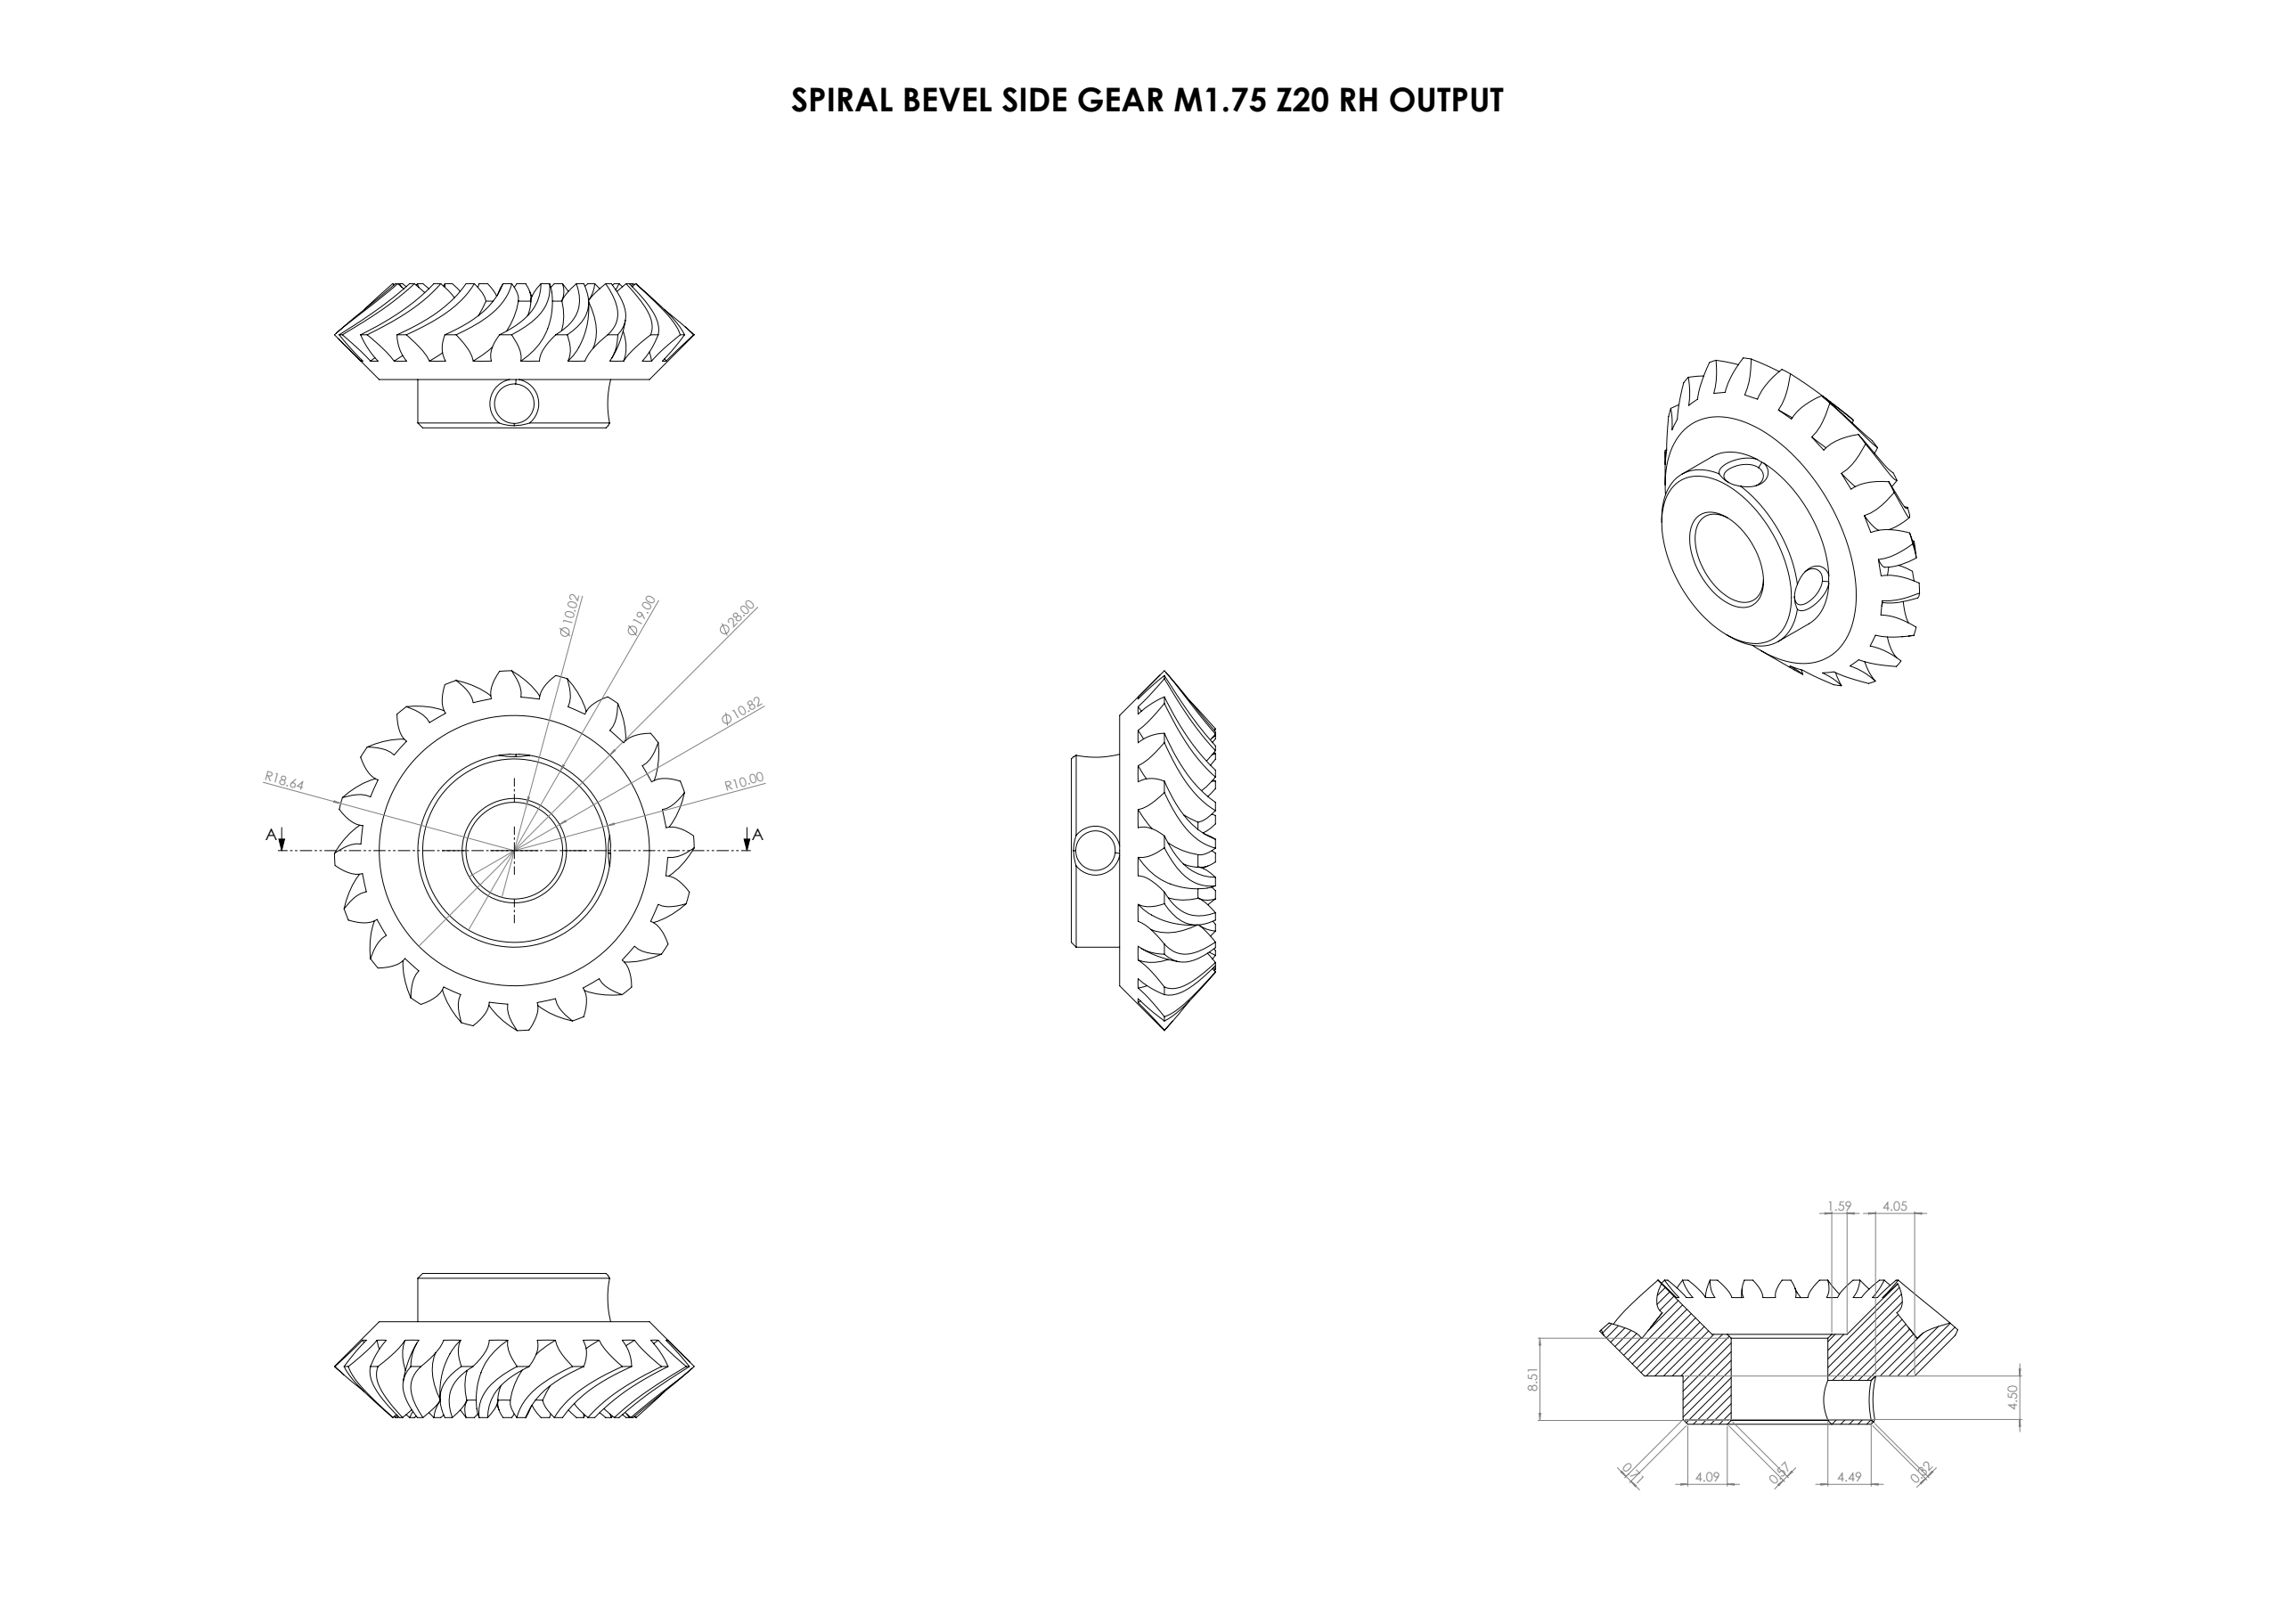
ISO-10303-21;
HEADER;
/* Generated by software containing ST-Developer
 * from STEP Tools, Inc. (www.steptools.com) 
 */

FILE_DESCRIPTION(
/* description */ (''),
/* implementation_level */ '2;1');

FILE_NAME(
/* name */ 
'04_Spiral_Bevel_Side_Gear_m1.75_z20_RH_Output.step',
/* time_stamp */ '2026-10-22T00:21:42-07:00',
/* author */ (''),
/* organization */ (''),
/* preprocessor_version */ 'ST-DEVELOPER v20.2',
/* originating_system */ 'Autodesk Translation Framework v15.15.0.0',
/* authorisation */ '');

FILE_SCHEMA (('AUTOMOTIVE_DESIGN { 1 0 10303 214 3 1 1 }'));
ENDSEC;

DATA;
#10=MECHANICAL_DESIGN_GEOMETRIC_PRESENTATION_REPRESENTATION('',(#208),#31638);
#186=SHAPE_REPRESENTATION_RELATIONSHIP('SRR','None',#31708,#197);
#197=ADVANCED_BREP_SHAPE_REPRESENTATION('',(#219),#31630);
#208=STYLED_ITEM('',(#31823),#219);
#219=MANIFOLD_SOLID_BREP('Spiral bevel gear',#12483);
#272=CYLINDRICAL_SURFACE('',#12901,1.);
#273=CYLINDRICAL_SURFACE('',#12905,1.);
#274=CYLINDRICAL_SURFACE('',#12908,0.205);
#275=CYLINDRICAL_SURFACE('',#12909,0.205);
#276=CYLINDRICAL_SURFACE('',#12981,0.501);
#406=CONICAL_SURFACE('',#12910,0.975,0.785398163397446);
#407=CONICAL_SURFACE('',#12912,1.63192209588552,0.785398163397448);
#408=CONICAL_SURFACE('',#12934,1.56260147929642,0.850360450324169);
#409=CONICAL_SURFACE('',#12936,1.56260147929642,0.850360450324169);
#410=CONICAL_SURFACE('',#12938,1.56260147929642,0.850360450324169);
#411=CONICAL_SURFACE('',#12940,1.56260147929642,0.850360450324169);
#412=CONICAL_SURFACE('',#12942,1.56260147929642,0.850360450324169);
#413=CONICAL_SURFACE('',#12944,1.56260147929642,0.850360450324169);
#414=CONICAL_SURFACE('',#12946,1.56260147929642,0.850360450324169);
#415=CONICAL_SURFACE('',#12948,1.56260147929642,0.850360450324169);
#416=CONICAL_SURFACE('',#12950,1.56260147929642,0.850360450324169);
#417=CONICAL_SURFACE('',#12952,1.56260147929642,0.850360450324169);
#418=CONICAL_SURFACE('',#12954,1.56260147929642,0.850360450324169);
#419=CONICAL_SURFACE('',#12956,1.56260147929642,0.850360450324169);
#420=CONICAL_SURFACE('',#12958,1.56260147929642,0.850360450324169);
#421=CONICAL_SURFACE('',#12960,1.56260147929642,0.850360450324169);
#422=CONICAL_SURFACE('',#12962,1.56260147929642,0.850360450324169);
#423=CONICAL_SURFACE('',#12964,1.56260147929642,0.850360450324169);
#424=CONICAL_SURFACE('',#12966,1.56260147929642,0.850360450324169);
#425=CONICAL_SURFACE('',#12968,1.56260147929642,0.850360450324169);
#426=CONICAL_SURFACE('',#12970,1.56260147929642,0.850360450324169);
#427=CONICAL_SURFACE('',#12972,0.980679383410898,0.785398163397448);
#428=CONICAL_SURFACE('',#12975,1.56260147929642,0.850360450324169);
#429=CONICAL_SURFACE('',#12979,0.521,0.785398163397448);
#430=CONICAL_SURFACE('',#12983,0.521,0.785398163397451);
#723=B_SPLINE_CURVE_WITH_KNOTS('',3,(#21270,#21271,#21272,#21273,#21274,
#21275,#21276,#21277,#21278,#21279,#21280,#21281,#21282,#21283,#21284,#21285,
#21286,#21287,#21288,#21289,#21290,#21291,#21292,#21293,#21294,#21295,#21296,
#21297,#21298,#21299,#21300,#21301,#21302,#21303),.UNSPECIFIED.,.F.,.F.,
(4,3,3,3,3,3,3,3,3,3,3,4),(0.,0.0110116267986798,0.0198365927950272,0.0393688637311641,
0.0455583406049715,0.0493231568143408,0.0527005792502689,0.056916196494854,
0.0651768568763584,0.0788461297337949,0.0828398890027903,0.100882854089343),
 .UNSPECIFIED.);
#724=B_SPLINE_CURVE_WITH_KNOTS('',3,(#21305,#21306,#21307,#21308,#21309,
#21310,#21311,#21312,#21313,#21314,#21315,#21316,#21317,#21318),
 .UNSPECIFIED.,.F.,.F.,(4,1,1,1,1,1,1,1,1,2,4),(-0.889886066635509,-0.843971490026765,
-0.78979558357151,-0.749163653730069,-0.681443770661001,-0.654355817433373,
-0.627267864205746,-0.600179910978118,-0.573091957750491,-0.464740144839981,
-0.44137654239973),.UNSPECIFIED.);
#725=B_SPLINE_CURVE_WITH_KNOTS('',3,(#21320,#21321,#21322,#21323,#21324,
#21325,#21326,#21327,#21328,#21329,#21330,#21331),.UNSPECIFIED.,.F.,.F.,
(4,2,2,2,2,4),(0.,0.0358257028990328,0.131952299625094,0.148884451735932,
0.157379698574708,0.16223106694039),.UNSPECIFIED.);
#726=B_SPLINE_CURVE_WITH_KNOTS('',3,(#21333,#21334,#21335,#21336),
 .UNSPECIFIED.,.F.,.F.,(4,4),(0.549999999941368,1.),.UNSPECIFIED.);
#727=B_SPLINE_CURVE_WITH_KNOTS('',3,(#21338,#21339,#21340,#21341,#21342,
#21343,#21344,#21345,#21346,#21347,#21348,#21349,#21350,#21351,#21352,#21353),
 .UNSPECIFIED.,.F.,.F.,(4,1,2,1,1,1,1,1,1,1,1,1,4),(0.310721506882948,0.387730825861464,
0.464740144839981,0.573091957750491,0.600179910978118,0.627267864205746,
0.654355817433373,0.681443770661001,0.749163653730069,0.78979558357151,
0.843971490026765,0.89814739648202,0.929489890414014),.UNSPECIFIED.);
#728=B_SPLINE_CURVE_WITH_KNOTS('',3,(#21354,#21355,#21356,#21357,#21358,
#21359,#21360,#21361,#21362,#21363,#21364,#21365,#21366,#21367,#21368,#21369,
#21370),.UNSPECIFIED.,.F.,.F.,(4,1,1,1,1,1,1,1,1,1,1,1,1,1,4),(0.929489890414014,
0.952323302937276,1.00649920939253,1.06067511584779,1.11485102230304,1.1690269287583,
1.22320283521355,1.26383476505499,1.33155464812406,1.35864260135169,1.38573055457932,
1.41281850780694,1.43990646103457,1.49408236748983,1.54825827394508),
 .UNSPECIFIED.);
#729=B_SPLINE_CURVE_WITH_KNOTS('',3,(#21372,#21373,#21374,#21375,#21376,
#21377,#21378,#21379,#21380,#21381,#21382,#21383,#21384,#21385),
 .UNSPECIFIED.,.F.,.F.,(4,2,2,2,2,2,4),(0.16223106694039,0.163967550885131,
0.171180716857468,0.182777598096348,0.205784524866042,0.262730804446443,
0.324280670363194),.UNSPECIFIED.);
#730=B_SPLINE_CURVE_WITH_KNOTS('',3,(#21386,#21387,#21388,#21389,#21390,
#21391,#21392,#21393,#21394,#21395,#21396,#21397,#21398,#21399),
 .UNSPECIFIED.,.F.,.F.,(4,1,1,1,1,1,1,1,1,1,1,4),(-1.4176032384283,-1.41281850780694,
-1.38573055457932,-1.35864260135169,-1.33155464812406,-1.26383476505499,
-1.22320283521355,-1.1690269287583,-1.11485102230304,-1.06067511584779,
-1.00649920939253,-0.969093714192518),.UNSPECIFIED.);
#731=B_SPLINE_CURVE_WITH_KNOTS('',3,(#21406,#21407,#21408,#21409,#21410,
#21411,#21412,#21413,#21414,#21415,#21416,#21417),.UNSPECIFIED.,.F.,.F.,
(4,1,1,1,1,1,1,2,4),(-1.50954599357819,-1.43295998077967,-1.38938999215504,
-1.34582000353042,-1.25868002628116,-1.21511003765654,-1.17154004903191,
-1.08440007178266,-1.06103646934241),.UNSPECIFIED.);
#732=B_SPLINE_CURVE_WITH_KNOTS('',3,(#21423,#21424,#21425,#21426,#21427,
#21428,#21429,#21430,#21431,#21432,#21433,#21434,#21435,#21436),
 .UNSPECIFIED.,.F.,.F.,(4,1,1,1,2,2,1,1,1,4),(-2.03726316537097,-2.03275764211163,
-2.01344899085789,-1.93621438584296,-1.85897978082803,-1.78151988977668,
-1.71616490683974,-1.69437991252743,-1.60723993527817,-1.58875364113519),
 .UNSPECIFIED.);
#733=B_SPLINE_CURVE_WITH_KNOTS('',3,(#21442,#21443,#21444,#21445,#21446,
#21447,#21448,#21449,#21450,#21451),.UNSPECIFIED.,.F.,.F.,(4,2,2,2,4),(0.,
0.0782721603764034,0.156544320752807,0.234729089704077,0.312913858655347),
 .UNSPECIFIED.);
#734=B_SPLINE_CURVE_WITH_KNOTS('',3,(#21452,#21453,#21454,#21455,#21456,
#21457,#21458,#21459,#21460,#21461,#21462,#21463,#21464,#21465,#21466,#21467,
#21468,#21469,#21470,#21471,#21472,#21473,#21474,#21475,#21476,#21477),
 .UNSPECIFIED.,.F.,.F.,(4,2,2,2,2,2,2,2,2,2,2,2,4),(0.312913858655347,0.391098627606618,
0.469283396557888,0.547555556934292,0.625827717310695,0.704099877687098,
0.782372038063502,0.860556807014772,0.938741575966043,1.01692634491731,
1.09511111386858,1.17338327424499,1.25165543462139),.UNSPECIFIED.);
#735=B_SPLINE_CURVE_WITH_KNOTS('',3,(#21590,#21591,#21592,#21593,#21594,
#21595,#21596,#21597,#21598,#21599,#21600,#21601,#21602,#21603,#21604,#21605,
#21606,#21607,#21608,#21609,#21610,#21611,#21612,#21613,#21614,#21615,#21616,
#21617,#21618,#21619,#21620,#21621,#21622,#21623,#21624,#21625,#21626),
 .UNSPECIFIED.,.F.,.F.,(4,3,3,3,3,3,3,3,3,3,3,3,4),(0.,0.0140126898858465,
0.0198365927950119,0.0393688637311589,0.0455583406050571,0.0493231568139791,
0.0527005792494364,0.0569161964938546,0.0651768568751002,0.0683276956644967,
0.0828398890011837,0.0964479725722503,0.100882854087323),.UNSPECIFIED.);
#736=B_SPLINE_CURVE_WITH_KNOTS('',3,(#21628,#21629,#21630,#21631,#21632,
#21633,#21634,#21635,#21636,#21637,#21638,#21639),.UNSPECIFIED.,.F.,.F.,
(4,2,2,2,2,4),(0.,0.0358257028990433,0.131952299625135,0.148884451735976,
0.157379698574799,0.162231066940522),.UNSPECIFIED.);
#737=B_SPLINE_CURVE_WITH_KNOTS('',3,(#21641,#21642,#21643,#21644),
 .UNSPECIFIED.,.F.,.F.,(4,4),(0.549999999941368,1.),.UNSPECIFIED.);
#738=B_SPLINE_CURVE_WITH_KNOTS('',3,(#21646,#21647,#21648,#21649,#21650,
#21651,#21652,#21653,#21654,#21655,#21656,#21657,#21658,#21659),
 .UNSPECIFIED.,.F.,.F.,(4,1,2,1,1,1,1,1,1,1,4),(0.930381433825624,1.00739075280414,
1.08440007178266,1.17154004903191,1.21511003765654,1.25868002628116,1.34582000353042,
1.38938999215504,1.43295998077967,1.52009995802892,1.54914981735669),
 .UNSPECIFIED.);
#739=B_SPLINE_CURVE_WITH_KNOTS('',3,(#21660,#21661,#21662,#21663,#21664,
#21665,#21666,#21667,#21668,#21669,#21670,#21671,#21672,#21673,#21674,#21675,
#21676,#21677),.UNSPECIFIED.,.F.,.F.,(4,1,1,1,1,1,2,2,1,1,1,1,1,4),(1.54914981735669,
1.56366994665355,1.58545494096586,1.60723993527817,1.69437991252743,1.71616490683974,
1.78151988977668,1.85897978082803,1.93621438584296,2.01344899085789,2.03275764211163,
2.05206629336536,2.09068359587282,2.16791820088776),.UNSPECIFIED.);
#740=B_SPLINE_CURVE_WITH_KNOTS('',3,(#21678,#21679,#21680,#21681,#21682,
#21683,#21684,#21685,#21686,#21687,#21688,#21689,#21690,#21691),
 .UNSPECIFIED.,.F.,.F.,(4,2,2,2,2,2,4),(0.162231066940522,0.163967550885278,
0.171180716857662,0.182777598096494,0.205784524865831,0.262730804445425,
0.324280670361326),.UNSPECIFIED.);
#741=B_SPLINE_CURVE_WITH_KNOTS('',3,(#21695,#21696,#21697,#21698,#21699,
#21700,#21701,#21702,#21703,#21704,#21705,#21706,#21707,#21708,#21709,#21710,
#21711,#21712,#21713,#21714,#21715,#21716,#21717,#21718,#21719,#21720),
 .UNSPECIFIED.,.F.,.F.,(4,2,2,2,2,2,2,2,2,2,2,2,4),(0.,0.0782721603764034,
0.156544320752807,0.234729089704077,0.312913858655348,0.391098627606618,
0.469283396557888,0.547555556934292,0.625827717310695,0.704099877687099,
0.782372038063502,0.860556807014772,0.938741575966043),.UNSPECIFIED.);
#742=B_SPLINE_CURVE_WITH_KNOTS('',3,(#21721,#21722,#21723,#21724,#21725,
#21726,#21727,#21728,#21729,#21730),.UNSPECIFIED.,.F.,.F.,(4,2,2,2,4),(0.938741575966043,
1.01692634491731,1.09511111386858,1.17338327424499,1.25165543462139),
 .UNSPECIFIED.);
#743=B_SPLINE_CURVE_WITH_KNOTS('',3,(#21762,#21763,#21764,#21765,#21766,
#21767),.UNSPECIFIED.,.F.,.F.,(4,2,4),(0.,0.138207529108851,0.257151380447634),
 .UNSPECIFIED.);
#744=B_SPLINE_CURVE_WITH_KNOTS('',3,(#21769,#21770,#21771,#21772,#21773,
#21774),.UNSPECIFIED.,.F.,.F.,(4,2,4),(0.0638119305867455,0.434740434623819,
0.895232561311264),.UNSPECIFIED.);
#745=B_SPLINE_CURVE_WITH_KNOTS('',3,(#21776,#21777,#21778,#21779,#21780,
#21781,#21782,#21783),.UNSPECIFIED.,.F.,.F.,(4,2,2,4),(0.0650199495982317,
0.170565165416136,0.226763969189742,0.268056752438448),.UNSPECIFIED.);
#746=B_SPLINE_CURVE_WITH_KNOTS('',3,(#21784,#21785,#21786,#21787,#21788,
#21789,#21790,#21791),.UNSPECIFIED.,.F.,.F.,(4,2,2,4),(0.0747583116411992,
0.415738779002342,0.772551101530307,1.04863108973719),.UNSPECIFIED.);
#747=B_SPLINE_CURVE_WITH_KNOTS('',3,(#21818,#21819,#21820,#21821,#21822,
#21823,#21824,#21825),.UNSPECIFIED.,.F.,.F.,(4,2,2,4),(0.0535030672285043,
0.137418922872643,0.199655718694958,0.252976612949483),.UNSPECIFIED.);
#748=B_SPLINE_CURVE_WITH_KNOTS('',3,(#21827,#21828,#21829,#21830,#21831,
#21832,#21833,#21834),.UNSPECIFIED.,.F.,.F.,(4,2,2,4),(0.11834343350373,
0.512336851961602,0.931707568041671,1.28239107793921),.UNSPECIFIED.);
#749=B_SPLINE_CURVE_WITH_KNOTS('',3,(#21836,#21837,#21838,#21839,#21840,
#21841),.UNSPECIFIED.,.F.,.F.,(4,2,4),(0.,0.208309927739493,0.384486154932789),
 .UNSPECIFIED.);
#750=B_SPLINE_CURVE_WITH_KNOTS('',3,(#21842,#21843,#21844,#21845,#21846,
#21847),.UNSPECIFIED.,.F.,.F.,(4,2,4),(0.0638119305867455,0.434740434623819,
0.895232561311264),.UNSPECIFIED.);
#751=B_SPLINE_CURVE_WITH_KNOTS('',3,(#21864,#21865,#21866,#21867,#21868,
#21869,#21870),.UNSPECIFIED.,.F.,.F.,(4,3,4),(0.,0.064975255706308,0.13035708562273),
 .UNSPECIFIED.);
#752=B_SPLINE_CURVE_WITH_KNOTS('',3,(#21871,#21872,#21873,#21874,#21875,
#21876,#21877),.UNSPECIFIED.,.F.,.F.,(4,3,4),(0.,0.0981730480407086,0.191890424805344),
 .UNSPECIFIED.);
#753=B_SPLINE_CURVE_WITH_KNOTS('',3,(#21884,#21885,#21886,#21887),
 .UNSPECIFIED.,.F.,.F.,(4,4),(0.331995637616086,0.384486154832915),
 .UNSPECIFIED.);
#754=B_SPLINE_CURVE_WITH_KNOTS('',3,(#21891,#21892,#21893,#21894,#21895,
#21896,#21897,#21898),.UNSPECIFIED.,.F.,.F.,(4,2,2,4),(0.0542087124698116,
0.203323725897707,0.32378750142016,0.520894956620335),.UNSPECIFIED.);
#755=B_SPLINE_CURVE_WITH_KNOTS('',3,(#21900,#21901,#21902,#21903,#21904,
#21905,#21906),.UNSPECIFIED.,.F.,.F.,(4,3,4),(0.,0.0981730480406908,0.191890424805207),
 .UNSPECIFIED.);
#756=B_SPLINE_CURVE_WITH_KNOTS('',3,(#21908,#21909,#21910,#21911,#21912,
#21913),.UNSPECIFIED.,.F.,.F.,(4,2,4),(0.,0.208309927750236,0.384486155029173),
 .UNSPECIFIED.);
#757=B_SPLINE_CURVE_WITH_KNOTS('',3,(#21917,#21918,#21919,#21920,#21921,
#21922,#21923,#21924),.UNSPECIFIED.,.F.,.F.,(4,2,2,4),(0.0650199496529384,
0.170565165647366,0.226763969524849,0.268056752853526),.UNSPECIFIED.);
#758=B_SPLINE_CURVE_WITH_KNOTS('',3,(#21926,#21927,#21928,#21929,#21930,
#21931,#21932),.UNSPECIFIED.,.F.,.F.,(4,3,4),(0.,0.0981730480406766,0.191890424805293),
 .UNSPECIFIED.);
#759=B_SPLINE_CURVE_WITH_KNOTS('',3,(#21934,#21935,#21936,#21937,#21938,
#21939),.UNSPECIFIED.,.F.,.F.,(4,2,4),(0.,0.208309927746205,0.38448615499989),
 .UNSPECIFIED.);
#760=B_SPLINE_CURVE_WITH_KNOTS('',3,(#21943,#21944,#21945,#21946,#21947,
#21948,#21949,#21950),.UNSPECIFIED.,.F.,.F.,(4,2,2,4),(0.0650199495839021,
0.170565165355256,0.226763969103251,0.268056752329737),.UNSPECIFIED.);
#761=B_SPLINE_CURVE_WITH_KNOTS('',3,(#21952,#21953,#21954,#21955,#21956,
#21957,#21958),.UNSPECIFIED.,.F.,.F.,(4,3,4),(0.,0.0981730480407384,0.191890424805265),
 .UNSPECIFIED.);
#762=B_SPLINE_CURVE_WITH_KNOTS('',3,(#21960,#21961,#21962,#21963,#21964,
#21965),.UNSPECIFIED.,.F.,.F.,(4,2,4),(0.,0.208309927742208,0.384486154882329),
 .UNSPECIFIED.);
#763=B_SPLINE_CURVE_WITH_KNOTS('',3,(#21969,#21970,#21971,#21972,#21973,
#21974,#21975,#21976),.UNSPECIFIED.,.F.,.F.,(4,2,2,4),(0.0650199495860717,
0.170565165364572,0.226763969117006,0.26805675235156),.UNSPECIFIED.);
#764=B_SPLINE_CURVE_WITH_KNOTS('',3,(#21978,#21979,#21980,#21981,#21982,
#21983,#21984),.UNSPECIFIED.,.F.,.F.,(4,3,4),(0.,0.098173048040732,0.191890424805364),
 .UNSPECIFIED.);
#765=B_SPLINE_CURVE_WITH_KNOTS('',3,(#21986,#21987,#21988,#21989,#21990,
#21991),.UNSPECIFIED.,.F.,.F.,(4,2,4),(0.,0.208309927745551,0.38448615497379),
 .UNSPECIFIED.);
#766=B_SPLINE_CURVE_WITH_KNOTS('',3,(#21995,#21996,#21997,#21998,#21999,
#22000,#22001,#22002),.UNSPECIFIED.,.F.,.F.,(4,2,2,4),(0.0650199495587532,
0.170565165249151,0.226763968946711,0.268056752139196),.UNSPECIFIED.);
#767=B_SPLINE_CURVE_WITH_KNOTS('',3,(#22004,#22005,#22006,#22007,#22008,
#22009,#22010),.UNSPECIFIED.,.F.,.F.,(4,3,4),(0.,0.098173048040845,0.191890424805652),
 .UNSPECIFIED.);
#768=B_SPLINE_CURVE_WITH_KNOTS('',3,(#22012,#22013,#22014,#22015,#22016,
#22017),.UNSPECIFIED.,.F.,.F.,(4,2,4),(0.,0.208309927731817,0.384486154823123),
 .UNSPECIFIED.);
#769=B_SPLINE_CURVE_WITH_KNOTS('',3,(#22021,#22022,#22023,#22024,#22025,
#22026,#22027,#22028),.UNSPECIFIED.,.F.,.F.,(4,2,2,4),(0.054208712440581,
0.203323725621083,0.32378750087977,0.520894955605601),.UNSPECIFIED.);
#770=B_SPLINE_CURVE_WITH_KNOTS('',3,(#22030,#22031,#22032,#22033,#22034,
#22035,#22036),.UNSPECIFIED.,.F.,.F.,(4,3,4),(0.,0.0981730480406625,0.19189042480521),
 .UNSPECIFIED.);
#771=B_SPLINE_CURVE_WITH_KNOTS('',3,(#22038,#22039,#22040,#22041,#22042,
#22043),.UNSPECIFIED.,.F.,.F.,(4,2,4),(0.,0.208309927743994,0.384486154966103),
 .UNSPECIFIED.);
#772=B_SPLINE_CURVE_WITH_KNOTS('',3,(#22047,#22048,#22049,#22050,#22051,
#22052,#22053,#22054),.UNSPECIFIED.,.F.,.F.,(4,2,2,4),(0.0650199496372336,
0.170565165580817,0.226763969430302,0.268056752734932),.UNSPECIFIED.);
#773=B_SPLINE_CURVE_WITH_KNOTS('',3,(#22056,#22057,#22058,#22059,#22060,
#22061,#22062),.UNSPECIFIED.,.F.,.F.,(4,3,4),(0.,0.0981730480407077,0.191890424805375),
 .UNSPECIFIED.);
#774=B_SPLINE_CURVE_WITH_KNOTS('',3,(#22064,#22065,#22066,#22067,#22068,
#22069),.UNSPECIFIED.,.F.,.F.,(4,2,4),(0.,0.20830992773469,0.384486154871887),
 .UNSPECIFIED.);
#775=B_SPLINE_CURVE_WITH_KNOTS('',3,(#22073,#22074,#22075,#22076,#22077,
#22078,#22079,#22080),.UNSPECIFIED.,.F.,.F.,(4,2,2,4),(0.0650199495866873,
0.170565165367095,0.226763969117418,0.268056752346729),.UNSPECIFIED.);
#776=B_SPLINE_CURVE_WITH_KNOTS('',3,(#22082,#22083,#22084,#22085,#22086,
#22087,#22088),.UNSPECIFIED.,.F.,.F.,(4,3,4),(0.,0.0981730480407126,0.191890424805348),
 .UNSPECIFIED.);
#777=B_SPLINE_CURVE_WITH_KNOTS('',3,(#22090,#22091,#22092,#22093,#22094,
#22095),.UNSPECIFIED.,.F.,.F.,(4,2,4),(0.,0.208309927751894,0.384486154960954),
 .UNSPECIFIED.);
#778=B_SPLINE_CURVE_WITH_KNOTS('',3,(#22099,#22100,#22101,#22102,#22103,
#22104,#22105,#22106),.UNSPECIFIED.,.F.,.F.,(4,2,2,4),(0.0650199495073989,
0.170565165032043,0.226763968637804,0.268056751759602),.UNSPECIFIED.);
#779=B_SPLINE_CURVE_WITH_KNOTS('',3,(#22108,#22109,#22110,#22111,#22112,
#22113,#22114),.UNSPECIFIED.,.F.,.F.,(4,3,4),(0.,0.0981730480406239,0.191890424805078),
 .UNSPECIFIED.);
#780=B_SPLINE_CURVE_WITH_KNOTS('',3,(#22116,#22117,#22118,#22119,#22120,
#22121),.UNSPECIFIED.,.F.,.F.,(4,2,4),(0.,0.20830992772829,0.384486154840441),
 .UNSPECIFIED.);
#781=B_SPLINE_CURVE_WITH_KNOTS('',3,(#22126,#22127,#22128,#22129,#22130,
#22131,#22132,#22133),.UNSPECIFIED.,.F.,.F.,(4,2,2,4),(0.0542611019730315,
0.202920016768632,0.323128184799993,0.520330951478027),.UNSPECIFIED.);
#782=B_SPLINE_CURVE_WITH_KNOTS('',3,(#22135,#22136,#22137,#22138,#22139,
#22140,#22141),.UNSPECIFIED.,.F.,.F.,(4,3,4),(0.,0.0981730480406862,0.19189042480528),
 .UNSPECIFIED.);
#783=B_SPLINE_CURVE_WITH_KNOTS('',3,(#22143,#22144,#22145,#22146,#22147,
#22148),.UNSPECIFIED.,.F.,.F.,(4,2,4),(0.,0.208309927742973,0.38448615495736),
 .UNSPECIFIED.);
#784=B_SPLINE_CURVE_WITH_KNOTS('',3,(#22152,#22153,#22154,#22155,#22156,
#22157,#22158,#22159),.UNSPECIFIED.,.F.,.F.,(4,2,2,4),(0.0650199495256298,
0.170565165109065,0.226763968747303,0.268056751893518),.UNSPECIFIED.);
#785=B_SPLINE_CURVE_WITH_KNOTS('',3,(#22161,#22162,#22163,#22164,#22165,
#22166,#22167),.UNSPECIFIED.,.F.,.F.,(4,3,4),(0.,0.0981730480407225,0.191890424805355),
 .UNSPECIFIED.);
#786=B_SPLINE_CURVE_WITH_KNOTS('',3,(#22169,#22170,#22171,#22172,#22173,
#22174),.UNSPECIFIED.,.F.,.F.,(4,2,4),(0.,0.208309927727119,0.384486154806359),
 .UNSPECIFIED.);
#787=B_SPLINE_CURVE_WITH_KNOTS('',3,(#22178,#22179,#22180,#22181,#22182,
#22183,#22184,#22185),.UNSPECIFIED.,.F.,.F.,(4,2,2,4),(0.0650199496379536,
0.170565165583986,0.22676396943225,0.26805675273395),.UNSPECIFIED.);
#788=B_SPLINE_CURVE_WITH_KNOTS('',3,(#22187,#22188,#22189,#22190,#22191,
#22192,#22193),.UNSPECIFIED.,.F.,.F.,(4,3,4),(0.,0.0981730480407346,0.191890424805321),
 .UNSPECIFIED.);
#789=B_SPLINE_CURVE_WITH_KNOTS('',3,(#22195,#22196,#22197,#22198,#22199,
#22200),.UNSPECIFIED.,.F.,.F.,(4,2,4),(0.,0.208309927739911,0.384486154953153),
 .UNSPECIFIED.);
#790=B_SPLINE_CURVE_WITH_KNOTS('',3,(#22204,#22205,#22206,#22207,#22208,
#22209,#22210,#22211),.UNSPECIFIED.,.F.,.F.,(4,2,2,4),(0.0650199495498999,
0.170565165211631,0.226763968890252,0.268056752070099),.UNSPECIFIED.);
#791=B_SPLINE_CURVE_WITH_KNOTS('',3,(#22213,#22214,#22215,#22216,#22217,
#22218,#22219),.UNSPECIFIED.,.F.,.F.,(4,3,4),(0.,0.098173048040742,0.191890424805327),
 .UNSPECIFIED.);
#792=B_SPLINE_CURVE_WITH_KNOTS('',3,(#22221,#22222,#22223,#22224,#22225,
#22226),.UNSPECIFIED.,.F.,.F.,(4,2,4),(0.,0.208309927725018,0.384486154743549),
 .UNSPECIFIED.);
#793=B_SPLINE_CURVE_WITH_KNOTS('',3,(#22230,#22231,#22232,#22233,#22234,
#22235,#22236,#22237),.UNSPECIFIED.,.F.,.F.,(4,2,2,4),(0.0650199494135083,
0.170565164635192,0.22676396805462,0.268056751043425),.UNSPECIFIED.);
#794=B_SPLINE_CURVE_WITH_KNOTS('',3,(#22239,#22240,#22241,#22242,#22243,
#22244,#22245),.UNSPECIFIED.,.F.,.F.,(4,3,4),(0.,0.098173048040714,0.191890424805356),
 .UNSPECIFIED.);
#795=B_SPLINE_CURVE_WITH_KNOTS('',3,(#22247,#22248,#22249,#22250,#22251,
#22252),.UNSPECIFIED.,.F.,.F.,(4,2,4),(0.,0.208309927737883,0.384486154890492),
 .UNSPECIFIED.);
#796=B_SPLINE_CURVE_WITH_KNOTS('',3,(#22256,#22257,#22258,#22259,#22260,
#22261,#22262,#22263),.UNSPECIFIED.,.F.,.F.,(4,2,2,4),(0.0542087124218259,
0.203323725443623,0.323787500531832,0.520894954944429),.UNSPECIFIED.);
#797=B_SPLINE_CURVE_WITH_KNOTS('',3,(#22265,#22266,#22267,#22268,#22269,
#22270,#22271),.UNSPECIFIED.,.F.,.F.,(4,3,4),(0.,0.098173048040669,0.191890424805223),
 .UNSPECIFIED.);
#798=B_SPLINE_CURVE_WITH_KNOTS('',3,(#22273,#22274,#22275,#22276,#22277,
#22278),.UNSPECIFIED.,.F.,.F.,(4,2,4),(0.,0.208309927750018,0.384486155023449),
 .UNSPECIFIED.);
#799=B_SPLINE_CURVE_WITH_KNOTS('',3,(#22282,#22283,#22284,#22285,#22286,
#22287,#22288,#22289),.UNSPECIFIED.,.F.,.F.,(4,2,2,4),(0.0650199496369929,
0.170565165579854,0.226763969431761,0.268056752734831),.UNSPECIFIED.);
#800=B_SPLINE_CURVE_WITH_KNOTS('',3,(#22291,#22292,#22293,#22294,#22295,
#22296,#22297),.UNSPECIFIED.,.F.,.F.,(4,3,4),(0.,0.098173048040829,0.191890424805588),
 .UNSPECIFIED.);
#801=B_SPLINE_CURVE_WITH_KNOTS('',3,(#22299,#22300,#22301,#22302,#22303,
#22304),.UNSPECIFIED.,.F.,.F.,(4,2,4),(0.,0.208309927736197,0.384486154842889),
 .UNSPECIFIED.);
#802=B_SPLINE_CURVE_WITH_KNOTS('',3,(#22308,#22309,#22310,#22311,#22312,
#22313,#22314,#22315),.UNSPECIFIED.,.F.,.F.,(4,2,2,4),(0.0650199495839219,
0.170565165355339,0.226763969103371,0.268056752329883),.UNSPECIFIED.);
#803=B_SPLINE_CURVE_WITH_KNOTS('',3,(#22317,#22318,#22319,#22320,#22321,
#22322,#22323),.UNSPECIFIED.,.F.,.F.,(4,3,4),(0.,0.0981730480406805,0.191890424805183),
 .UNSPECIFIED.);
#804=B_SPLINE_CURVE_WITH_KNOTS('',3,(#22325,#22326,#22327,#22328,#22329,
#22330),.UNSPECIFIED.,.F.,.F.,(4,2,4),(0.,0.208309927742222,0.384486154882313),
 .UNSPECIFIED.);
#805=B_SPLINE_CURVE_WITH_KNOTS('',3,(#22334,#22335,#22336,#22337,#22338,
#22339,#22340,#22341),.UNSPECIFIED.,.F.,.F.,(4,2,2,4),(0.0650199495861818,
0.170565165365035,0.226763969117688,0.268056752352361),.UNSPECIFIED.);
#806=B_SPLINE_CURVE_WITH_KNOTS('',3,(#22343,#22344,#22345,#22346,#22347,
#22348,#22349),.UNSPECIFIED.,.F.,.F.,(4,3,4),(0.,0.0981730480406793,0.191890424805241),
 .UNSPECIFIED.);
#807=B_SPLINE_CURVE_WITH_KNOTS('',3,(#22351,#22352,#22353,#22354,#22355,
#22356),.UNSPECIFIED.,.F.,.F.,(4,2,4),(0.,0.208309927745549,0.384486154973776),
 .UNSPECIFIED.);
#808=B_SPLINE_CURVE_WITH_KNOTS('',3,(#22360,#22361,#22362,#22363,#22364,
#22365,#22366,#22367),.UNSPECIFIED.,.F.,.F.,(4,2,2,4),(0.0650199495195806,
0.1705651650837,0.226763968706434,0.268056751843866),.UNSPECIFIED.);
#809=B_SPLINE_CURVE_WITH_KNOTS('',3,(#22369,#22370,#22371,#22372,#22373,
#22374,#22375),.UNSPECIFIED.,.F.,.F.,(4,3,4),(0.,0.0981730480406788,0.191890424805225),
 .UNSPECIFIED.);
#810=B_SPLINE_CURVE_WITH_KNOTS('',3,(#22376,#22377,#22378,#22379,#22380,
#22381),.UNSPECIFIED.,.F.,.F.,(4,2,4),(0.,0.208309927731304,0.331995637616086),
 .UNSPECIFIED.);
#811=B_SPLINE_CURVE_WITH_KNOTS('',3,(#22385,#22386,#22387,#22388,#22389,
#22390,#22391,#22392),.UNSPECIFIED.,.F.,.F.,(4,2,2,4),(0.0747583116412021,
0.415738779002311,0.753026862713569,1.0479673638265),.UNSPECIFIED.);
#812=B_SPLINE_CURVE_WITH_KNOTS('',3,(#22395,#22396,#22397,#22398,#22399,
#22400,#22401,#22402),.UNSPECIFIED.,.F.,.F.,(4,2,2,4),(0.154059232628148,
0.534434525764867,0.968745967316882,1.33329265533026),.UNSPECIFIED.);
#813=B_SPLINE_CURVE_WITH_KNOTS('',3,(#22430,#22431,#22432,#22433,#22434,
#22435),.UNSPECIFIED.,.F.,.F.,(4,2,4),(0.,0.138207529109353,0.25715138045422),
 .UNSPECIFIED.);
#814=B_SPLINE_CURVE_WITH_KNOTS('',3,(#22436,#22437,#22438,#22439,#22440,
#22441),.UNSPECIFIED.,.F.,.F.,(4,2,4),(0.0638119305867454,0.434740434623819,
0.895232561311264),.UNSPECIFIED.);
#815=B_SPLINE_CURVE_WITH_KNOTS('',3,(#22442,#22443,#22444,#22445,#22446,
#22447,#22448,#22449),.UNSPECIFIED.,.F.,.F.,(4,2,2,4),(0.0747583116411993,
0.415738779002422,0.772551101530389,1.0486310897372),.UNSPECIFIED.);
#816=B_SPLINE_CURVE_WITH_KNOTS('',3,(#22475,#22476,#22477,#22478,#22479,
#22480,#22481,#22482),.UNSPECIFIED.,.F.,.F.,(4,2,2,4),(0.053503067227966,
0.137418922870269,0.199655718696157,0.252976612954111),.UNSPECIFIED.);
#817=B_SPLINE_CURVE_WITH_KNOTS('',3,(#22483,#22484,#22485,#22486,#22487,
#22488),.UNSPECIFIED.,.F.,.F.,(4,2,4),(0.0638119305867453,0.434740434623819,
0.895232561311263),.UNSPECIFIED.);
#818=B_SPLINE_CURVE_WITH_KNOTS('',3,(#22505,#22506,#22507,#22508,#22509,
#22510,#22511),.UNSPECIFIED.,.F.,.F.,(4,3,4),(0.,0.0649752557063318,0.130357085622803),
 .UNSPECIFIED.);
#819=B_SPLINE_CURVE_WITH_KNOTS('',3,(#22514,#22515,#22516,#22517,#22518,
#22519,#22520,#22521),.UNSPECIFIED.,.F.,.F.,(4,2,2,4),(0.154059232628334,
0.534434525767114,0.968745967322665,1.33329265533901),.UNSPECIFIED.);
#820=B_SPLINE_CURVE_WITH_KNOTS('',3,(#22549,#22550,#22551,#22552,#22553,
#22554),.UNSPECIFIED.,.F.,.F.,(4,2,4),(0.,0.138207529109416,0.257151380444098),
 .UNSPECIFIED.);
#821=B_SPLINE_CURVE_WITH_KNOTS('',3,(#22555,#22556,#22557,#22558,#22559,
#22560),.UNSPECIFIED.,.F.,.F.,(4,2,4),(0.0638119305867455,0.434740434623819,
0.895232561311264),.UNSPECIFIED.);
#822=B_SPLINE_CURVE_WITH_KNOTS('',3,(#22561,#22562,#22563,#22564,#22565,
#22566,#22567,#22568),.UNSPECIFIED.,.F.,.F.,(4,2,2,4),(0.0747583116412007,
0.41573877900245,0.772551101530441,1.04863108973726),.UNSPECIFIED.);
#823=B_SPLINE_CURVE_WITH_KNOTS('',3,(#22594,#22595,#22596,#22597,#22598,
#22599,#22600,#22601),.UNSPECIFIED.,.F.,.F.,(4,2,2,4),(0.0535030672291814,
0.137418922876081,0.19965571870634,0.252976612971294),.UNSPECIFIED.);
#824=B_SPLINE_CURVE_WITH_KNOTS('',3,(#22602,#22603,#22604,#22605,#22606,
#22607),.UNSPECIFIED.,.F.,.F.,(4,2,4),(0.0638119305867455,0.434740434623819,
0.895232561311264),.UNSPECIFIED.);
#825=B_SPLINE_CURVE_WITH_KNOTS('',3,(#22624,#22625,#22626,#22627,#22628,
#22629,#22630),.UNSPECIFIED.,.F.,.F.,(4,3,4),(0.,0.0649752557062639,0.130357085622636),
 .UNSPECIFIED.);
#826=B_SPLINE_CURVE_WITH_KNOTS('',3,(#22633,#22634,#22635,#22636,#22637,
#22638,#22639,#22640),.UNSPECIFIED.,.F.,.F.,(4,2,2,4),(0.154059232628307,
0.534434525766854,0.968745967321853,1.33329265533773),.UNSPECIFIED.);
#827=B_SPLINE_CURVE_WITH_KNOTS('',3,(#22668,#22669,#22670,#22671,#22672,
#22673),.UNSPECIFIED.,.F.,.F.,(4,2,4),(0.,0.138207529110581,0.257151380456836),
 .UNSPECIFIED.);
#828=B_SPLINE_CURVE_WITH_KNOTS('',3,(#22674,#22675,#22676,#22677,#22678,
#22679),.UNSPECIFIED.,.F.,.F.,(4,2,4),(0.0638119305867455,0.434740434623819,
0.895232561311264),.UNSPECIFIED.);
#829=B_SPLINE_CURVE_WITH_KNOTS('',3,(#22680,#22681,#22682,#22683,#22684,
#22685,#22686,#22687),.UNSPECIFIED.,.F.,.F.,(4,2,2,4),(0.0747583116412006,
0.415738779002382,0.772551101530378,1.04863108973727),.UNSPECIFIED.);
#830=B_SPLINE_CURVE_WITH_KNOTS('',3,(#22713,#22714,#22715,#22716,#22717,
#22718,#22719,#22720),.UNSPECIFIED.,.F.,.F.,(4,2,2,4),(0.0535030672284625,
0.137418922872139,0.199655718694633,0.252976612947559),.UNSPECIFIED.);
#831=B_SPLINE_CURVE_WITH_KNOTS('',3,(#22721,#22722,#22723,#22724,#22725,
#22726),.UNSPECIFIED.,.F.,.F.,(4,2,4),(0.0638119305867455,0.434740434623819,
0.895232561311264),.UNSPECIFIED.);
#832=B_SPLINE_CURVE_WITH_KNOTS('',3,(#22743,#22744,#22745,#22746,#22747,
#22748,#22749),.UNSPECIFIED.,.F.,.F.,(4,3,4),(0.,0.0649752557062745,0.130357085622644),
 .UNSPECIFIED.);
#833=B_SPLINE_CURVE_WITH_KNOTS('',3,(#22752,#22753,#22754,#22755,#22756,
#22757,#22758,#22759),.UNSPECIFIED.,.F.,.F.,(4,2,2,4),(0.154059232628089,
0.534434525764075,0.968745967315031,1.33329265532752),.UNSPECIFIED.);
#834=B_SPLINE_CURVE_WITH_KNOTS('',3,(#22787,#22788,#22789,#22790,#22791,
#22792),.UNSPECIFIED.,.F.,.F.,(4,2,4),(0.,0.138207529113509,0.257151380470495),
 .UNSPECIFIED.);
#835=B_SPLINE_CURVE_WITH_KNOTS('',3,(#22793,#22794,#22795,#22796,#22797,
#22798),.UNSPECIFIED.,.F.,.F.,(4,2,4),(0.0638119305867455,0.434740434623819,
0.895232561311264),.UNSPECIFIED.);
#836=B_SPLINE_CURVE_WITH_KNOTS('',3,(#22799,#22800,#22801,#22802,#22803,
#22804,#22805,#22806),.UNSPECIFIED.,.F.,.F.,(4,2,2,4),(0.0747583116412008,
0.415738779002339,0.752886816639909,1.04796308482473),.UNSPECIFIED.);
#837=B_SPLINE_CURVE_WITH_KNOTS('',3,(#22832,#22833,#22834,#22835,#22836,
#22837,#22838,#22839),.UNSPECIFIED.,.F.,.F.,(4,2,2,4),(0.0535030672285657,
0.137418922872968,0.199655718696181,0.252976612951919),.UNSPECIFIED.);
#838=B_SPLINE_CURVE_WITH_KNOTS('',3,(#22840,#22841,#22842,#22843,#22844,
#22845),.UNSPECIFIED.,.F.,.F.,(4,2,4),(0.0638119305867455,0.434740434623819,
0.895232561311264),.UNSPECIFIED.);
#839=B_SPLINE_CURVE_WITH_KNOTS('',3,(#22862,#22863,#22864,#22865,#22866,
#22867,#22868),.UNSPECIFIED.,.F.,.F.,(4,3,4),(0.,0.0649752557062603,0.130357085622615),
 .UNSPECIFIED.);
#840=B_SPLINE_CURVE_WITH_KNOTS('',3,(#22871,#22872,#22873,#22874,#22875,
#22876,#22877,#22878),.UNSPECIFIED.,.F.,.F.,(4,2,2,4),(0.118343433503666,
0.512336851960316,0.93170756803854,1.28239107793455),.UNSPECIFIED.);
#841=B_SPLINE_CURVE_WITH_KNOTS('',3,(#22906,#22907,#22908,#22909,#22910,
#22911),.UNSPECIFIED.,.F.,.F.,(4,2,4),(0.,0.138207529110136,0.257151380458292),
 .UNSPECIFIED.);
#842=B_SPLINE_CURVE_WITH_KNOTS('',3,(#22912,#22913,#22914,#22915,#22916,
#22917),.UNSPECIFIED.,.F.,.F.,(4,2,4),(0.0638119305867455,0.434740434623819,
0.895232561311264),.UNSPECIFIED.);
#843=B_SPLINE_CURVE_WITH_KNOTS('',3,(#22918,#22919,#22920,#22921,#22922,
#22923,#22924,#22925),.UNSPECIFIED.,.F.,.F.,(4,2,2,4),(0.0747583116411991,
0.415738779002339,0.772551101530305,1.04863108973718),.UNSPECIFIED.);
#844=B_SPLINE_CURVE_WITH_KNOTS('',3,(#22951,#22952,#22953,#22954,#22955,
#22956,#22957,#22958),.UNSPECIFIED.,.F.,.F.,(4,2,2,4),(0.0535030672288839,
0.137418922874274,0.199655718698583,0.252976612955408),.UNSPECIFIED.);
#845=B_SPLINE_CURVE_WITH_KNOTS('',3,(#22959,#22960,#22961,#22962,#22963,
#22964),.UNSPECIFIED.,.F.,.F.,(4,2,4),(0.0638119305867455,0.434740434623819,
0.895232561311264),.UNSPECIFIED.);
#846=B_SPLINE_CURVE_WITH_KNOTS('',3,(#22981,#22982,#22983,#22984,#22985,
#22986,#22987),.UNSPECIFIED.,.F.,.F.,(4,3,4),(0.,0.0649752557063269,0.130357085622762),
 .UNSPECIFIED.);
#847=B_SPLINE_CURVE_WITH_KNOTS('',3,(#22990,#22991,#22992,#22993,#22994,
#22995,#22996,#22997),.UNSPECIFIED.,.F.,.F.,(4,2,2,4),(0.154059232628121,
0.53443452576449,0.968745967316035,1.33329265532902),.UNSPECIFIED.);
#848=B_SPLINE_CURVE_WITH_KNOTS('',3,(#23025,#23026,#23027,#23028,#23029,
#23030),.UNSPECIFIED.,.F.,.F.,(4,2,4),(0.,0.138207529111244,0.257151380457893),
 .UNSPECIFIED.);
#849=B_SPLINE_CURVE_WITH_KNOTS('',3,(#23031,#23032,#23033,#23034,#23035,
#23036),.UNSPECIFIED.,.F.,.F.,(4,2,4),(0.0638119305867455,0.434740434623819,
0.895232561311264),.UNSPECIFIED.);
#850=B_SPLINE_CURVE_WITH_KNOTS('',3,(#23037,#23038,#23039,#23040,#23041,
#23042,#23043,#23044),.UNSPECIFIED.,.F.,.F.,(4,2,2,4),(0.074758311641198,
0.415738779002409,0.772551101530352,1.04863108973713),.UNSPECIFIED.);
#851=B_SPLINE_CURVE_WITH_KNOTS('',3,(#23070,#23071,#23072,#23073,#23074,
#23075,#23076,#23077),.UNSPECIFIED.,.F.,.F.,(4,2,2,4),(0.0535030672292633,
0.137418922876037,0.199655718701109,0.252976612961143),.UNSPECIFIED.);
#852=B_SPLINE_CURVE_WITH_KNOTS('',3,(#23078,#23079,#23080,#23081,#23082,
#23083),.UNSPECIFIED.,.F.,.F.,(4,2,4),(0.0638119305867455,0.434740434623819,
0.895232561311264),.UNSPECIFIED.);
#853=B_SPLINE_CURVE_WITH_KNOTS('',3,(#23100,#23101,#23102,#23103,#23104,
#23105,#23106),.UNSPECIFIED.,.F.,.F.,(4,3,4),(0.,0.064975255706295,0.130357085622655),
 .UNSPECIFIED.);
#854=B_SPLINE_CURVE_WITH_KNOTS('',3,(#23109,#23110,#23111,#23112,#23113,
#23114,#23115,#23116),.UNSPECIFIED.,.F.,.F.,(4,2,2,4),(0.154059232628213,
0.53443452576567,0.968745967318966,1.33329265533342),.UNSPECIFIED.);
#855=B_SPLINE_CURVE_WITH_KNOTS('',3,(#23144,#23145,#23146,#23147,#23148,
#23149),.UNSPECIFIED.,.F.,.F.,(4,2,4),(0.,0.138207529110641,0.257151380449519),
 .UNSPECIFIED.);
#856=B_SPLINE_CURVE_WITH_KNOTS('',3,(#23150,#23151,#23152,#23153,#23154,
#23155),.UNSPECIFIED.,.F.,.F.,(4,2,4),(0.0638119305867454,0.434740434623819,
0.895232561311263),.UNSPECIFIED.);
#857=B_SPLINE_CURVE_WITH_KNOTS('',3,(#23156,#23157,#23158,#23159,#23160,
#23161,#23162,#23163),.UNSPECIFIED.,.F.,.F.,(4,2,2,4),(0.0747583116411987,
0.415738779002504,0.772551101530452,1.04863108973715),.UNSPECIFIED.);
#858=B_SPLINE_CURVE_WITH_KNOTS('',3,(#23189,#23190,#23191,#23192,#23193,
#23194,#23195,#23196),.UNSPECIFIED.,.F.,.F.,(4,2,2,4),(0.0535030672291719,
0.137418922876308,0.199655718705506,0.252976612970481),.UNSPECIFIED.);
#859=B_SPLINE_CURVE_WITH_KNOTS('',3,(#23197,#23198,#23199,#23200,#23201,
#23202),.UNSPECIFIED.,.F.,.F.,(4,2,4),(0.0638119305867453,0.434740434623819,
0.895232561311264),.UNSPECIFIED.);
#860=B_SPLINE_CURVE_WITH_KNOTS('',3,(#23219,#23220,#23221,#23222,#23223,
#23224,#23225),.UNSPECIFIED.,.F.,.F.,(4,3,4),(0.,0.0649752557063512,0.130357085622858),
 .UNSPECIFIED.);
#861=B_SPLINE_CURVE_WITH_KNOTS('',3,(#23228,#23229,#23230,#23231,#23232,
#23233,#23234,#23235),.UNSPECIFIED.,.F.,.F.,(4,2,2,4),(0.15405923262826,
0.534434525766248,0.968745967320369,1.33329265533552),.UNSPECIFIED.);
#862=B_SPLINE_CURVE_WITH_KNOTS('',3,(#23263,#23264,#23265,#23266,#23267,
#23268),.UNSPECIFIED.,.F.,.F.,(4,2,4),(0.,0.138207529110164,0.257151380454439),
 .UNSPECIFIED.);
#863=B_SPLINE_CURVE_WITH_KNOTS('',3,(#23269,#23270,#23271,#23272,#23273,
#23274),.UNSPECIFIED.,.F.,.F.,(4,2,4),(0.0638119305867455,0.434740434623819,
0.895232561311264),.UNSPECIFIED.);
#864=B_SPLINE_CURVE_WITH_KNOTS('',3,(#23275,#23276,#23277,#23278,#23279,
#23280,#23281,#23282),.UNSPECIFIED.,.F.,.F.,(4,2,2,4),(0.0747583116411995,
0.415738779002478,0.772551101530437,1.04863108973718),.UNSPECIFIED.);
#865=B_SPLINE_CURVE_WITH_KNOTS('',3,(#23308,#23309,#23310,#23311,#23312,
#23313,#23314,#23315),.UNSPECIFIED.,.F.,.F.,(4,2,2,4),(0.0535030672281601,
0.137418922870713,0.199655718691404,0.252976612943466),.UNSPECIFIED.);
#866=B_SPLINE_CURVE_WITH_KNOTS('',3,(#23316,#23317,#23318,#23319,#23320,
#23321),.UNSPECIFIED.,.F.,.F.,(4,2,4),(0.0638119305867454,0.434740434623819,
0.895232561311264),.UNSPECIFIED.);
#867=B_SPLINE_CURVE_WITH_KNOTS('',3,(#23338,#23339,#23340,#23341,#23342,
#23343,#23344),.UNSPECIFIED.,.F.,.F.,(4,3,4),(0.,0.0649752557063186,0.130357085622797),
 .UNSPECIFIED.);
#868=B_SPLINE_CURVE_WITH_KNOTS('',3,(#23347,#23348,#23349,#23350,#23351,
#23352,#23353,#23354),.UNSPECIFIED.,.F.,.F.,(4,2,2,4),(0.154059232628401,
0.534434525767925,0.968745967324708,1.33329265534209),.UNSPECIFIED.);
#869=B_SPLINE_CURVE_WITH_KNOTS('',3,(#23382,#23383,#23384,#23385,#23386,
#23387),.UNSPECIFIED.,.F.,.F.,(4,2,4),(0.,0.138207529107339,0.257151380437116),
 .UNSPECIFIED.);
#870=B_SPLINE_CURVE_WITH_KNOTS('',3,(#23388,#23389,#23390,#23391,#23392,
#23393),.UNSPECIFIED.,.F.,.F.,(4,2,4),(0.0638119305867455,0.434740434623819,
0.895232561311264),.UNSPECIFIED.);
#871=B_SPLINE_CURVE_WITH_KNOTS('',3,(#23394,#23395,#23396,#23397,#23398,
#23399,#23400,#23401),.UNSPECIFIED.,.F.,.F.,(4,2,2,4),(0.0747583116412006,
0.41573877900234,0.752886816639902,1.0479630848247),.UNSPECIFIED.);
#872=B_SPLINE_CURVE_WITH_KNOTS('',3,(#23427,#23428,#23429,#23430),
 .UNSPECIFIED.,.F.,.F.,(4,4),(0.053503067228538,0.100640802838924),
 .UNSPECIFIED.);
#873=B_SPLINE_CURVE_WITH_KNOTS('',3,(#23432,#23433,#23434,#23435,#23436,
#23437),.UNSPECIFIED.,.F.,.F.,(4,2,4),(0.0638119305867455,0.434740434623819,
0.895232561311264),.UNSPECIFIED.);
#874=B_SPLINE_CURVE_WITH_KNOTS('',3,(#23438,#23439,#23440,#23441,#23442,
#23443,#23444,#23445),.UNSPECIFIED.,.F.,.F.,(4,2,2,4),(0.100640802838924,
0.13741892287284,0.199655718695611,0.252976612950919),.UNSPECIFIED.);
#875=B_SPLINE_CURVE_WITH_KNOTS('',3,(#23462,#23463,#23464,#23465,#23466,
#23467,#23468),.UNSPECIFIED.,.F.,.F.,(4,3,4),(0.,0.0649752557062351,0.130357085622553),
 .UNSPECIFIED.);
#876=B_SPLINE_CURVE_WITH_KNOTS('',3,(#23471,#23472,#23473,#23474,#23475,
#23476,#23477,#23478),.UNSPECIFIED.,.F.,.F.,(4,2,2,4),(0.11834343350374,
0.512336851961745,0.931707568042095,1.28239107793988),.UNSPECIFIED.);
#877=B_SPLINE_CURVE_WITH_KNOTS('',3,(#23506,#23507,#23508,#23509,#23510,
#23511),.UNSPECIFIED.,.F.,.F.,(4,2,4),(0.,0.138207529109375,0.257151380450338),
 .UNSPECIFIED.);
#878=B_SPLINE_CURVE_WITH_KNOTS('',3,(#23512,#23513,#23514,#23515,#23516,
#23517),.UNSPECIFIED.,.F.,.F.,(4,2,4),(0.0638119305867455,0.434740434623819,
0.895232561311264),.UNSPECIFIED.);
#879=B_SPLINE_CURVE_WITH_KNOTS('',3,(#23518,#23519,#23520,#23521,#23522,
#23523,#23524,#23525),.UNSPECIFIED.,.F.,.F.,(4,2,2,4),(0.0747583116412016,
0.415738779002347,0.772551101530358,1.04863108973731),.UNSPECIFIED.);
#880=B_SPLINE_CURVE_WITH_KNOTS('',3,(#23551,#23552,#23553,#23554,#23555,
#23556,#23557,#23558),.UNSPECIFIED.,.F.,.F.,(4,2,2,4),(0.0535030672288559,
0.13741892287429,0.199655718700123,0.252976612958485),.UNSPECIFIED.);
#881=B_SPLINE_CURVE_WITH_KNOTS('',3,(#23559,#23560,#23561,#23562,#23563,
#23564),.UNSPECIFIED.,.F.,.F.,(4,2,4),(0.0638119305867455,0.434740434623819,
0.895232561311264),.UNSPECIFIED.);
#882=B_SPLINE_CURVE_WITH_KNOTS('',3,(#23581,#23582,#23583,#23584,#23585,
#23586,#23587),.UNSPECIFIED.,.F.,.F.,(4,3,4),(0.,0.0649752557062924,0.130357085622708),
 .UNSPECIFIED.);
#883=B_SPLINE_CURVE_WITH_KNOTS('',3,(#23590,#23591,#23592,#23593,#23594,
#23595,#23596,#23597),.UNSPECIFIED.,.F.,.F.,(4,2,2,4),(0.154059232628241,
0.534434525766006,0.968745967319776,1.33329265533462),.UNSPECIFIED.);
#884=B_SPLINE_CURVE_WITH_KNOTS('',3,(#23625,#23626,#23627,#23628,#23629,
#23630),.UNSPECIFIED.,.F.,.F.,(4,2,4),(0.,0.138207529111243,0.257151380457902),
 .UNSPECIFIED.);
#885=B_SPLINE_CURVE_WITH_KNOTS('',3,(#23631,#23632,#23633,#23634,#23635,
#23636),.UNSPECIFIED.,.F.,.F.,(4,2,4),(0.0638119305867455,0.434740434623819,
0.895232561311264),.UNSPECIFIED.);
#886=B_SPLINE_CURVE_WITH_KNOTS('',3,(#23637,#23638,#23639,#23640,#23641,
#23642,#23643,#23644),.UNSPECIFIED.,.F.,.F.,(4,2,2,4),(0.0747583116411995,
0.415738779002564,0.772551101530526,1.04863108973719),.UNSPECIFIED.);
#887=B_SPLINE_CURVE_WITH_KNOTS('',3,(#23670,#23671,#23672,#23673,#23674,
#23675,#23676,#23677),.UNSPECIFIED.,.F.,.F.,(4,2,2,4),(0.0535030672292643,
0.13741892287604,0.199655718701115,0.252976612961142),.UNSPECIFIED.);
#888=B_SPLINE_CURVE_WITH_KNOTS('',3,(#23678,#23679,#23680,#23681,#23682,
#23683),.UNSPECIFIED.,.F.,.F.,(4,2,4),(0.0638119305867455,0.434740434623819,
0.895232561311264),.UNSPECIFIED.);
#889=B_SPLINE_CURVE_WITH_KNOTS('',3,(#23700,#23701,#23702,#23703,#23704,
#23705,#23706),.UNSPECIFIED.,.F.,.F.,(4,3,4),(0.,0.0649752557062854,0.130357085622667),
 .UNSPECIFIED.);
#890=B_SPLINE_CURVE_WITH_KNOTS('',3,(#23709,#23710,#23711,#23712,#23713,
#23714,#23715,#23716),.UNSPECIFIED.,.F.,.F.,(4,2,2,4),(0.154059232628168,
0.534434525765134,0.968745967317506,1.33329265533118),.UNSPECIFIED.);
#891=B_SPLINE_CURVE_WITH_KNOTS('',3,(#23744,#23745,#23746,#23747,#23748,
#23749),.UNSPECIFIED.,.F.,.F.,(4,2,4),(0.,0.138207529112972,0.257151380462745),
 .UNSPECIFIED.);
#892=B_SPLINE_CURVE_WITH_KNOTS('',3,(#23750,#23751,#23752,#23753,#23754,
#23755),.UNSPECIFIED.,.F.,.F.,(4,2,4),(0.0638119305867454,0.434740434623819,
0.895232561311263),.UNSPECIFIED.);
#893=B_SPLINE_CURVE_WITH_KNOTS('',3,(#23756,#23757,#23758,#23759,#23760,
#23761,#23762,#23763),.UNSPECIFIED.,.F.,.F.,(4,2,2,4),(0.0747583116411983,
0.415738779002571,0.772551101530515,1.04863108973714),.UNSPECIFIED.);
#894=B_SPLINE_CURVE_WITH_KNOTS('',3,(#23789,#23790,#23791,#23792,#23793,
#23794,#23795,#23796),.UNSPECIFIED.,.F.,.F.,(4,2,2,4),(0.0535030672291713,
0.137418922876305,0.199655718705507,0.252976612970469),.UNSPECIFIED.);
#895=B_SPLINE_CURVE_WITH_KNOTS('',3,(#23797,#23798,#23799,#23800,#23801,
#23802),.UNSPECIFIED.,.F.,.F.,(4,2,4),(0.0638119305867453,0.434740434623819,
0.895232561311264),.UNSPECIFIED.);
#896=B_SPLINE_CURVE_WITH_KNOTS('',3,(#23819,#23820,#23821,#23822,#23823,
#23824,#23825),.UNSPECIFIED.,.F.,.F.,(4,3,4),(0.,0.0649752557062912,0.130357085622682),
 .UNSPECIFIED.);
#897=B_SPLINE_CURVE_WITH_KNOTS('',3,(#23828,#23829,#23830,#23831,#23832,
#23833,#23834,#23835),.UNSPECIFIED.,.F.,.F.,(4,2,2,4),(0.154059232628393,
0.534434525767844,0.968745967324445,1.33329265534166),.UNSPECIFIED.);
#898=B_SPLINE_CURVE_WITH_KNOTS('',3,(#23863,#23864,#23865,#23866,#23867,
#23868),.UNSPECIFIED.,.F.,.F.,(4,2,4),(0.,0.138207529110578,0.257151380453696),
 .UNSPECIFIED.);
#899=B_SPLINE_CURVE_WITH_KNOTS('',3,(#23869,#23870,#23871,#23872,#23873,
#23874),.UNSPECIFIED.,.F.,.F.,(4,2,4),(0.0638119305867454,0.434740434623819,
0.895232561311264),.UNSPECIFIED.);
#900=B_SPLINE_CURVE_WITH_KNOTS('',3,(#23875,#23876,#23877,#23878,#23879,
#23880,#23881,#23882),.UNSPECIFIED.,.F.,.F.,(4,2,2,4),(0.0747583116412008,
0.415738779002461,0.77255110153044,1.04863108973723),.UNSPECIFIED.);
#901=B_SPLINE_CURVE_WITH_KNOTS('',3,(#23908,#23909,#23910,#23911,#23912,
#23913,#23914,#23915),.UNSPECIFIED.,.F.,.F.,(4,2,2,4),(0.0535030672281967,
0.137418922870822,0.199655718691029,0.252976612941727),.UNSPECIFIED.);
#902=B_SPLINE_CURVE_WITH_KNOTS('',3,(#23916,#23917,#23918,#23919,#23920,
#23921),.UNSPECIFIED.,.F.,.F.,(4,2,4),(0.0638119305867454,0.434740434623819,
0.895232561311264),.UNSPECIFIED.);
#903=B_SPLINE_CURVE_WITH_KNOTS('',3,(#23938,#23939,#23940,#23941,#23942,
#23943,#23944),.UNSPECIFIED.,.F.,.F.,(4,3,4),(0.,0.0649752557062974,0.130357085622712),
 .UNSPECIFIED.);
#904=B_SPLINE_CURVE_WITH_KNOTS('',3,(#23947,#23948,#23949,#23950,#23951,
#23952,#23953,#23954),.UNSPECIFIED.,.F.,.F.,(4,2,2,4),(0.154059232628199,
0.534434525765498,0.968745967318458,1.33329265533263),.UNSPECIFIED.);
#905=B_SPLINE_CURVE_WITH_KNOTS('',3,(#23982,#23983,#23984,#23985,#23986,
#23987),.UNSPECIFIED.,.F.,.F.,(4,2,4),(0.,0.138207529113734,0.257151380471648),
 .UNSPECIFIED.);
#906=B_SPLINE_CURVE_WITH_KNOTS('',3,(#23988,#23989,#23990,#23991,#23992,
#23993),.UNSPECIFIED.,.F.,.F.,(4,2,4),(0.0638119305867455,0.434740434623819,
0.895232561311264),.UNSPECIFIED.);
#907=B_SPLINE_CURVE_WITH_KNOTS('',3,(#23994,#23995,#23996,#23997,#23998,
#23999,#24000,#24001),.UNSPECIFIED.,.F.,.F.,(4,2,2,4),(0.074758311641198,
0.41573877900249,0.752886816639918,1.0479630848246),.UNSPECIFIED.);
#908=B_SPLINE_CURVE_WITH_KNOTS('',3,(#24027,#24028,#24029,#24030,#24031,
#24032,#24033,#24034),.UNSPECIFIED.,.F.,.F.,(4,2,2,4),(0.0535030672285459,
0.137418922872875,0.199655718695463,0.252976612950634),.UNSPECIFIED.);
#909=B_SPLINE_CURVE_WITH_KNOTS('',3,(#24035,#24036,#24037,#24038,#24039,
#24040),.UNSPECIFIED.,.F.,.F.,(4,2,4),(0.0638119305867455,0.434740434623819,
0.895232561311264),.UNSPECIFIED.);
#910=B_SPLINE_CURVE_WITH_KNOTS('',3,(#24057,#24058,#24059,#24060,#24061,
#24062,#24063),.UNSPECIFIED.,.F.,.F.,(4,3,4),(0.,0.0649752557063032,0.130357085622734),
 .UNSPECIFIED.);
#911=B_SPLINE_CURVE_WITH_KNOTS('',3,(#24066,#24067,#24068,#24069,#24070,
#24071,#24072,#24073),.UNSPECIFIED.,.F.,.F.,(4,2,2,4),(0.118343433503678,
0.512336851960549,0.931707568039129,1.28239107793543),.UNSPECIFIED.);
#912=B_SPLINE_CURVE_WITH_KNOTS('',3,(#24101,#24102,#24103,#24104,#24105,
#24106),.UNSPECIFIED.,.F.,.F.,(4,2,4),(0.,0.138207529112825,0.257151380461063),
 .UNSPECIFIED.);
#913=B_SPLINE_CURVE_WITH_KNOTS('',3,(#24107,#24108,#24109,#24110,#24111,
#24112),.UNSPECIFIED.,.F.,.F.,(4,2,4),(0.0638119305867454,0.434740434623819,
0.895232561311264),.UNSPECIFIED.);
#914=B_SPLINE_CURVE_WITH_KNOTS('',3,(#24113,#24114,#24115,#24116,#24117,
#24118,#24119,#24120),.UNSPECIFIED.,.F.,.F.,(4,2,2,4),(0.0747583116412005,
0.415738779002413,0.772551101530409,1.04863108973728),.UNSPECIFIED.);
#915=B_SPLINE_CURVE_WITH_KNOTS('',3,(#24146,#24147,#24148,#24149,#24150,
#24151,#24152,#24153),.UNSPECIFIED.,.F.,.F.,(4,2,2,4),(0.0535030672285232,
0.137418922872583,0.199655718694823,0.252976612949017),.UNSPECIFIED.);
#916=B_SPLINE_CURVE_WITH_KNOTS('',3,(#24154,#24155,#24156,#24157,#24158,
#24159),.UNSPECIFIED.,.F.,.F.,(4,2,4),(0.0638119305867454,0.434740434623819,
0.895232561311264),.UNSPECIFIED.);
#917=B_SPLINE_CURVE_WITH_KNOTS('',3,(#24176,#24177,#24178,#24179,#24180,
#24181,#24182),.UNSPECIFIED.,.F.,.F.,(4,3,4),(0.,0.0649752557062746,0.130357085622654),
 .UNSPECIFIED.);
#918=B_SPLINE_CURVE_WITH_KNOTS('',3,(#24185,#24186,#24187,#24188,#24189,
#24190,#24191,#24192),.UNSPECIFIED.,.F.,.F.,(4,2,2,4),(0.154059232628271,
0.534434525766387,0.968745967320721,1.33329265533604),.UNSPECIFIED.);
#919=B_SPLINE_CURVE_WITH_KNOTS('',3,(#24220,#24221,#24222,#24223,#24224,
#24225),.UNSPECIFIED.,.F.,.F.,(4,2,4),(0.,0.138207529114044,0.257151380464847),
 .UNSPECIFIED.);
#920=B_SPLINE_CURVE_WITH_KNOTS('',3,(#24226,#24227,#24228,#24229,#24230,
#24231),.UNSPECIFIED.,.F.,.F.,(4,2,4),(0.0638119305867455,0.434740434623819,
0.895232561311264),.UNSPECIFIED.);
#921=B_SPLINE_CURVE_WITH_KNOTS('',3,(#24232,#24233,#24234,#24235,#24236,
#24237,#24238,#24239),.UNSPECIFIED.,.F.,.F.,(4,2,2,4),(0.0747583116412018,
0.415738779002431,0.772551101530457,1.04863108973735),.UNSPECIFIED.);
#922=B_SPLINE_CURVE_WITH_KNOTS('',3,(#24265,#24266,#24267,#24268,#24269,
#24270,#24271,#24272),.UNSPECIFIED.,.F.,.F.,(4,2,2,4),(0.053503067228947,
0.137418922874791,0.199655718705812,0.252976612970407),.UNSPECIFIED.);
#923=B_SPLINE_CURVE_WITH_KNOTS('',3,(#24273,#24274,#24275,#24276,#24277,
#24278),.UNSPECIFIED.,.F.,.F.,(4,2,4),(0.0638119305867455,0.434740434623819,
0.895232561311264),.UNSPECIFIED.);
#924=B_SPLINE_CURVE_WITH_KNOTS('',3,(#24295,#24296,#24297,#24298,#24299,
#24300,#24301),.UNSPECIFIED.,.F.,.F.,(4,3,4),(0.,0.0649752557062623,0.130357085622632),
 .UNSPECIFIED.);
#925=B_SPLINE_CURVE_WITH_KNOTS('',3,(#24304,#24305,#24306,#24307,#24308,
#24309,#24310,#24311),.UNSPECIFIED.,.F.,.F.,(4,2,2,4),(0.154059232628193,
0.534434525765401,0.968745967318279,1.33329265533237),.UNSPECIFIED.);
#926=B_SPLINE_CURVE_WITH_KNOTS('',3,(#24339,#24340,#24341,#24342,#24343,
#24344),.UNSPECIFIED.,.F.,.F.,(4,2,4),(0.,0.13820752911105,0.257151380454454),
 .UNSPECIFIED.);
#927=B_SPLINE_CURVE_WITH_KNOTS('',3,(#24345,#24346,#24347,#24348,#24349,
#24350),.UNSPECIFIED.,.F.,.F.,(4,2,4),(0.0638119305867455,0.434740434623819,
0.895232561311264),.UNSPECIFIED.);
#928=B_SPLINE_CURVE_WITH_KNOTS('',3,(#24351,#24352,#24353,#24354,#24355,
#24356,#24357,#24358),.UNSPECIFIED.,.F.,.F.,(4,2,2,4),(0.074758311641201,
0.415738779002626,0.772551101530626,1.0486310897373),.UNSPECIFIED.);
#929=B_SPLINE_CURVE_WITH_KNOTS('',3,(#24384,#24385,#24386,#24387,#24388,
#24389,#24390,#24391),.UNSPECIFIED.,.F.,.F.,(4,2,2,4),(0.0535030672290782,
0.137418922874952,0.199655718700024,0.252976612958131),.UNSPECIFIED.);
#930=B_SPLINE_CURVE_WITH_KNOTS('',3,(#24392,#24393,#24394,#24395,#24396,
#24397),.UNSPECIFIED.,.F.,.F.,(4,2,4),(0.0638119305867455,0.434740434623819,
0.895232561311264),.UNSPECIFIED.);
#931=B_SPLINE_CURVE_WITH_KNOTS('',3,(#24414,#24415,#24416,#24417,#24418,
#24419,#24420),.UNSPECIFIED.,.F.,.F.,(4,3,4),(0.,0.0649752557062915,0.130357085622713),
 .UNSPECIFIED.);
#932=B_SPLINE_CURVE_WITH_KNOTS('',3,(#24423,#24424,#24425,#24426,#24427,
#24428,#24429,#24430),.UNSPECIFIED.,.F.,.F.,(4,2,2,4),(0.154059232628257,
0.534434525766122,0.968745967320132,1.33329265533518),.UNSPECIFIED.);
#933=B_SPLINE_CURVE_WITH_KNOTS('',3,(#24457,#24458,#24459,#24460,#24461,
#24462),.UNSPECIFIED.,.F.,.F.,(4,2,4),(0.0638119305867453,0.434740434623819,
0.895232561311263),.UNSPECIFIED.);
#934=B_SPLINE_CURVE_WITH_KNOTS('',3,(#24463,#24464,#24465,#24466,#24467,
#24468,#24469,#24470),.UNSPECIFIED.,.F.,.F.,(4,2,2,4),(0.0535030672280216,
0.137418922870031,0.199655718689467,0.2529766129386),.UNSPECIFIED.);
#935=B_SPLINE_CURVE_WITH_KNOTS('',3,(#24488,#24489,#24490,#24491,#24492,
#24493),.UNSPECIFIED.,.F.,.F.,(4,2,4),(0.0638119305867453,0.434740434623819,
0.895232561311264),.UNSPECIFIED.);
#936=B_SPLINE_CURVE_WITH_KNOTS('',3,(#24494,#24495,#24496,#24497,#24498,
#24499,#24500),.UNSPECIFIED.,.F.,.F.,(4,3,4),(0.,0.0649752557062552,0.130357085622604),
 .UNSPECIFIED.);
#937=B_SPLINE_CURVE_WITH_KNOTS('',3,(#24526,#24527,#24528,#24529,#24530,
#24531,#24532,#24533),.UNSPECIFIED.,.F.,.F.,(4,2,2,4),(0.074758311641199,
0.415738779002503,0.77255110153046,1.04863108973717),.UNSPECIFIED.);
#938=B_SPLINE_CURVE_WITH_KNOTS('',3,(#24534,#24535,#24536,#24537,#24538,
#24539),.UNSPECIFIED.,.F.,.F.,(4,2,4),(0.,0.138207529110333,0.257151380458365),
 .UNSPECIFIED.);
#939=B_SPLINE_CURVE_WITH_KNOTS('',3,(#24565,#24566,#24567,#24568,#24569,
#24570),.UNSPECIFIED.,.F.,.F.,(4,2,4),(0.0638119305867455,0.434740434623819,
0.895232561311264),.UNSPECIFIED.);
#940=B_SPLINE_CURVE_WITH_KNOTS('',3,(#24572,#24573,#24574,#24575,#24576,
#24577,#24578,#24579),.UNSPECIFIED.,.F.,.F.,(4,2,2,4),(0.0535030672285654,
0.137418922872966,0.199655718695898,0.252976612951402),.UNSPECIFIED.);
#941=B_SPLINE_CURVE_WITH_KNOTS('',3,(#24580,#24581,#24582,#24583,#24584,
#24585,#24586,#24587),.UNSPECIFIED.,.F.,.F.,(4,2,2,4),(0.154059232628261,
0.534434525766262,0.96874596732043,1.33329265533561),.UNSPECIFIED.);
#942=B_SPLINE_CURVE_WITH_KNOTS('',3,(#24605,#24606,#24607,#24608,#24609,
#24610),.UNSPECIFIED.,.F.,.F.,(4,2,4),(0.0638119305867455,0.434740434623819,
0.895232561311264),.UNSPECIFIED.);
#943=B_SPLINE_CURVE_WITH_KNOTS('',3,(#24611,#24612,#24613,#24614,#24615,
#24616,#24617),.UNSPECIFIED.,.F.,.F.,(4,3,4),(0.,0.0649752557063237,0.130357085622785),
 .UNSPECIFIED.);
#944=B_SPLINE_CURVE_WITH_KNOTS('',3,(#24642,#24643,#24644,#24645,#24646,
#24647),.UNSPECIFIED.,.F.,.F.,(4,2,4),(0.,0.13820752910729,0.257151380436842),
 .UNSPECIFIED.);
#1268=B_SPLINE_SURFACE_WITH_KNOTS('',3,3,((#21152,#21153,#21154,#21155,
#21156,#21157,#21158,#21159,#21160,#21161,#21162,#21163,#21164,#21165,#21166,
#21167,#21168,#21169,#21170,#21171,#21172,#21173,#21174,#21175,#21176,#21177,
#21178,#21179,#21180),(#21181,#21182,#21183,#21184,#21185,#21186,#21187,
#21188,#21189,#21190,#21191,#21192,#21193,#21194,#21195,#21196,#21197,#21198,
#21199,#21200,#21201,#21202,#21203,#21204,#21205,#21206,#21207,#21208,#21209),
(#21210,#21211,#21212,#21213,#21214,#21215,#21216,#21217,#21218,#21219,
#21220,#21221,#21222,#21223,#21224,#21225,#21226,#21227,#21228,#21229,#21230,
#21231,#21232,#21233,#21234,#21235,#21236,#21237,#21238),(#21239,#21240,
#21241,#21242,#21243,#21244,#21245,#21246,#21247,#21248,#21249,#21250,#21251,
#21252,#21253,#21254,#21255,#21256,#21257,#21258,#21259,#21260,#21261,#21262,
#21263,#21264,#21265,#21266,#21267)),.UNSPECIFIED.,.F.,.T.,.F.,(4,4),(4,
1,2,1,1,1,1,1,1,1,1,1,1,1,1,1,1,1,1,1,1,1,1,1,1,4),(0.,1.),(0.310721506882948,
0.387730825861464,0.464740144839981,0.573091957750491,0.600179910978118,
0.627267864205746,0.654355817433373,0.681443770661001,0.749163653730069,
0.78979558357151,0.843971490026765,0.89814739648202,0.952323302937276,1.00649920939253,
1.06067511584779,1.11485102230304,1.1690269287583,1.22320283521355,1.26383476505499,
1.33155464812406,1.35864260135169,1.38573055457932,1.41281850780694,1.43990646103457,
1.49408236748983,1.54825827394508),.UNSPECIFIED.);
#1269=B_SPLINE_SURFACE_WITH_KNOTS('',3,3,((#21478,#21479,#21480,#21481,
#21482,#21483,#21484,#21485,#21486,#21487,#21488,#21489,#21490,#21491,#21492,
#21493,#21494,#21495,#21496,#21497,#21498,#21499,#21500,#21501,#21502,#21503,
#21504,#21505),(#21506,#21507,#21508,#21509,#21510,#21511,#21512,#21513,
#21514,#21515,#21516,#21517,#21518,#21519,#21520,#21521,#21522,#21523,#21524,
#21525,#21526,#21527,#21528,#21529,#21530,#21531,#21532,#21533),(#21534,
#21535,#21536,#21537,#21538,#21539,#21540,#21541,#21542,#21543,#21544,#21545,
#21546,#21547,#21548,#21549,#21550,#21551,#21552,#21553,#21554,#21555,#21556,
#21557,#21558,#21559,#21560,#21561),(#21562,#21563,#21564,#21565,#21566,
#21567,#21568,#21569,#21570,#21571,#21572,#21573,#21574,#21575,#21576,#21577,
#21578,#21579,#21580,#21581,#21582,#21583,#21584,#21585,#21586,#21587,#21588,
#21589)),.UNSPECIFIED.,.F.,.T.,.F.,(4,4),(4,1,2,1,1,1,1,1,1,1,1,1,1,1,1,
2,2,1,1,1,1,1,4),(0.,1.),(0.930381433825624,1.00739075280414,1.08440007178266,
1.17154004903191,1.21511003765654,1.25868002628116,1.34582000353042,1.38938999215504,
1.43295998077967,1.52009995802892,1.56366994665355,1.58545494096586,1.60723993527817,
1.69437991252743,1.71616490683974,1.78151988977668,1.85897978082803,1.93621438584296,
2.01344899085789,2.03275764211163,2.05206629336536,2.09068359587282,2.16791820088776),
 .UNSPECIFIED.);
#1270=B_SPLINE_SURFACE_WITH_KNOTS('',3,3,((#21736,#21737,#21738,#21739),
(#21740,#21741,#21742,#21743),(#21744,#21745,#21746,#21747),(#21748,#21749,
#21750,#21751),(#21752,#21753,#21754,#21755),(#21756,#21757,#21758,#21759)),
 .UNSPECIFIED.,.F.,.F.,.F.,(4,1,1,4),(4,4),(0.,0.243643268493762,0.487286536987524,
0.852751439728166),(0.0593287711114826,0.89552230135485),.UNSPECIFIED.);
#1271=B_SPLINE_SURFACE_WITH_KNOTS('',3,3,((#21792,#21793,#21794,#21795),
(#21796,#21797,#21798,#21799),(#21800,#21801,#21802,#21803),(#21804,#21805,
#21806,#21807),(#21808,#21809,#21810,#21811),(#21812,#21813,#21814,#21815)),
 .UNSPECIFIED.,.F.,.F.,.F.,(4,1,1,4),(4,4),(0.145114332397141,0.511493904226938,
0.755746952113469,1.),(0.0593282329032902,0.895635080262268),
 .UNSPECIFIED.);
#1272=B_SPLINE_SURFACE_WITH_KNOTS('',3,3,((#21848,#21849,#21850,#21851),
(#21852,#21853,#21854,#21855),(#21856,#21857,#21858,#21859),(#21860,#21861,
#21862,#21863)),.UNSPECIFIED.,.F.,.F.,.F.,(4,4),(4,4),(0.,1.),(0.0638119305867453,
0.897818175643156),.UNSPECIFIED.);
#1273=B_SPLINE_SURFACE_WITH_KNOTS('',3,3,((#22404,#22405,#22406,#22407),
(#22408,#22409,#22410,#22411),(#22412,#22413,#22414,#22415),(#22416,#22417,
#22418,#22419),(#22420,#22421,#22422,#22423),(#22424,#22425,#22426,#22427)),
 .UNSPECIFIED.,.F.,.F.,.F.,(4,1,1,4),(4,4),(0.,0.182732451370321,0.365464902740643,
0.852751439728166),(0.0593287711114824,0.895522301354867),.UNSPECIFIED.);
#1274=B_SPLINE_SURFACE_WITH_KNOTS('',3,3,((#22450,#22451,#22452,#22453),
(#22454,#22455,#22456,#22457),(#22458,#22459,#22460,#22461),(#22462,#22463,
#22464,#22465),(#22466,#22467,#22468,#22469),(#22470,#22471,#22472,#22473)),
 .UNSPECIFIED.,.F.,.F.,.F.,(4,1,1,4),(4,4),(0.145491947870824,0.63378226337321,
0.816891131686605,1.),(0.0593282329020183,0.895635080262244),
 .UNSPECIFIED.);
#1275=B_SPLINE_SURFACE_WITH_KNOTS('',3,3,((#22489,#22490,#22491,#22492),
(#22493,#22494,#22495,#22496),(#22497,#22498,#22499,#22500),(#22501,#22502,
#22503,#22504)),.UNSPECIFIED.,.F.,.F.,.F.,(4,4),(4,4),(0.,1.),(0.0638119305867452,
0.897818175643156),.UNSPECIFIED.);
#1276=B_SPLINE_SURFACE_WITH_KNOTS('',3,3,((#22523,#22524,#22525,#22526),
(#22527,#22528,#22529,#22530),(#22531,#22532,#22533,#22534),(#22535,#22536,
#22537,#22538),(#22539,#22540,#22541,#22542),(#22543,#22544,#22545,#22546)),
 .UNSPECIFIED.,.F.,.F.,.F.,(4,1,1,4),(4,4),(0.,0.182732451370321,0.365464902740643,
0.852751439728167),(0.0593287711114828,0.895522301354858),.UNSPECIFIED.);
#1277=B_SPLINE_SURFACE_WITH_KNOTS('',3,3,((#22569,#22570,#22571,#22572),
(#22573,#22574,#22575,#22576),(#22577,#22578,#22579,#22580),(#22581,#22582,
#22583,#22584),(#22585,#22586,#22587,#22588),(#22589,#22590,#22591,#22592)),
 .UNSPECIFIED.,.F.,.F.,.F.,(4,1,1,4),(4,4),(0.145491947870788,0.633782263373195,
0.816891131686597,1.),(0.0593282329020185,0.89563508026229),
 .UNSPECIFIED.);
#1278=B_SPLINE_SURFACE_WITH_KNOTS('',3,3,((#22608,#22609,#22610,#22611),
(#22612,#22613,#22614,#22615),(#22616,#22617,#22618,#22619),(#22620,#22621,
#22622,#22623)),.UNSPECIFIED.,.F.,.F.,.F.,(4,4),(4,4),(0.,1.),(0.0638119305867454,
0.897818175643156),.UNSPECIFIED.);
#1279=B_SPLINE_SURFACE_WITH_KNOTS('',3,3,((#22642,#22643,#22644,#22645),
(#22646,#22647,#22648,#22649),(#22650,#22651,#22652,#22653),(#22654,#22655,
#22656,#22657),(#22658,#22659,#22660,#22661),(#22662,#22663,#22664,#22665)),
 .UNSPECIFIED.,.F.,.F.,.F.,(4,1,1,4),(4,4),(0.,0.182732451370321,0.365464902740643,
0.852751439728166),(0.0593287711114824,0.895522301354853),.UNSPECIFIED.);
#1280=B_SPLINE_SURFACE_WITH_KNOTS('',3,3,((#22688,#22689,#22690,#22691),
(#22692,#22693,#22694,#22695),(#22696,#22697,#22698,#22699),(#22700,#22701,
#22702,#22703),(#22704,#22705,#22706,#22707),(#22708,#22709,#22710,#22711)),
 .UNSPECIFIED.,.F.,.F.,.F.,(4,1,1,4),(4,4),(0.145491947870791,0.633782263373196,
0.816891131686598,1.),(0.0593282329020185,0.895635080262257),
 .UNSPECIFIED.);
#1281=B_SPLINE_SURFACE_WITH_KNOTS('',3,3,((#22727,#22728,#22729,#22730),
(#22731,#22732,#22733,#22734),(#22735,#22736,#22737,#22738),(#22739,#22740,
#22741,#22742)),.UNSPECIFIED.,.F.,.F.,.F.,(4,4),(4,4),(0.,1.),(0.0638119305867454,
0.897818175643157),.UNSPECIFIED.);
#1282=B_SPLINE_SURFACE_WITH_KNOTS('',3,3,((#22761,#22762,#22763,#22764),
(#22765,#22766,#22767,#22768),(#22769,#22770,#22771,#22772),(#22773,#22774,
#22775,#22776),(#22777,#22778,#22779,#22780),(#22781,#22782,#22783,#22784)),
 .UNSPECIFIED.,.F.,.F.,.F.,(4,1,1,4),(4,4),(0.,0.243691231740892,0.487382463481784,
0.852919311093121),(0.0593287711114826,0.895503416457802),.UNSPECIFIED.);
#1283=B_SPLINE_SURFACE_WITH_KNOTS('',3,3,((#22807,#22808,#22809,#22810),
(#22811,#22812,#22813,#22814),(#22815,#22816,#22817,#22818),(#22819,#22820,
#22821,#22822),(#22823,#22824,#22825,#22826),(#22827,#22828,#22829,#22830)),
 .UNSPECIFIED.,.F.,.F.,.F.,(4,1,1,4),(4,4),(0.145491947870838,0.511709684497622,
0.755854842248811,1.),(0.0593282329020186,0.895635080262274),
 .UNSPECIFIED.);
#1284=B_SPLINE_SURFACE_WITH_KNOTS('',3,3,((#22846,#22847,#22848,#22849),
(#22850,#22851,#22852,#22853),(#22854,#22855,#22856,#22857),(#22858,#22859,
#22860,#22861)),.UNSPECIFIED.,.F.,.F.,.F.,(4,4),(4,4),(0.,1.),(0.0638119305867452,
0.897818175643157),.UNSPECIFIED.);
#1285=B_SPLINE_SURFACE_WITH_KNOTS('',3,3,((#22880,#22881,#22882,#22883),
(#22884,#22885,#22886,#22887),(#22888,#22889,#22890,#22891),(#22892,#22893,
#22894,#22895),(#22896,#22897,#22898,#22899),(#22900,#22901,#22902,#22903)),
 .UNSPECIFIED.,.F.,.F.,.F.,(4,1,1,4),(4,4),(0.,0.182732451370321,0.365464902740643,
0.852751439728166),(0.0593287711114825,0.895522301354848),.UNSPECIFIED.);
#1286=B_SPLINE_SURFACE_WITH_KNOTS('',3,3,((#22926,#22927,#22928,#22929),
(#22930,#22931,#22932,#22933),(#22934,#22935,#22936,#22937),(#22938,#22939,
#22940,#22941),(#22942,#22943,#22944,#22945),(#22946,#22947,#22948,#22949)),
 .UNSPECIFIED.,.F.,.F.,.F.,(4,1,1,4),(4,4),(0.145114332397166,0.511493904226952,
0.755746952113476,1.),(0.0593282329032902,0.895635080262249),
 .UNSPECIFIED.);
#1287=B_SPLINE_SURFACE_WITH_KNOTS('',3,3,((#22965,#22966,#22967,#22968),
(#22969,#22970,#22971,#22972),(#22973,#22974,#22975,#22976),(#22977,#22978,
#22979,#22980)),.UNSPECIFIED.,.F.,.F.,.F.,(4,4),(4,4),(0.,1.),(0.0638119305867454,
0.897818175643156),.UNSPECIFIED.);
#1288=B_SPLINE_SURFACE_WITH_KNOTS('',3,3,((#22999,#23000,#23001,#23002),
(#23003,#23004,#23005,#23006),(#23007,#23008,#23009,#23010),(#23011,#23012,
#23013,#23014),(#23015,#23016,#23017,#23018),(#23019,#23020,#23021,#23022)),
 .UNSPECIFIED.,.F.,.F.,.F.,(4,1,1,4),(4,4),(0.,0.182732451370321,0.365464902740642,
0.852751439728166),(0.0593287711114824,0.895522301354846),.UNSPECIFIED.);
#1289=B_SPLINE_SURFACE_WITH_KNOTS('',3,3,((#23045,#23046,#23047,#23048),
(#23049,#23050,#23051,#23052),(#23053,#23054,#23055,#23056),(#23057,#23058,
#23059,#23060),(#23061,#23062,#23063,#23064),(#23065,#23066,#23067,#23068)),
 .UNSPECIFIED.,.F.,.F.,.F.,(4,1,1,4),(4,4),(0.145491947870832,0.511709684497618,
0.755854842248809,1.),(0.0593282329020186,0.895635080262275),
 .UNSPECIFIED.);
#1290=B_SPLINE_SURFACE_WITH_KNOTS('',3,3,((#23084,#23085,#23086,#23087),
(#23088,#23089,#23090,#23091),(#23092,#23093,#23094,#23095),(#23096,#23097,
#23098,#23099)),.UNSPECIFIED.,.F.,.F.,.F.,(4,4),(4,4),(0.,1.),(0.0638119305867453,
0.897818175643157),.UNSPECIFIED.);
#1291=B_SPLINE_SURFACE_WITH_KNOTS('',3,3,((#23118,#23119,#23120,#23121),
(#23122,#23123,#23124,#23125),(#23126,#23127,#23128,#23129),(#23130,#23131,
#23132,#23133),(#23134,#23135,#23136,#23137),(#23138,#23139,#23140,#23141)),
 .UNSPECIFIED.,.F.,.F.,.F.,(4,1,1,4),(4,4),(0.,0.243643268493762,0.487286536987524,
0.852751439728166),(0.0593287711114823,0.895522301354865),.UNSPECIFIED.);
#1292=B_SPLINE_SURFACE_WITH_KNOTS('',3,3,((#23164,#23165,#23166,#23167),
(#23168,#23169,#23170,#23171),(#23172,#23173,#23174,#23175),(#23176,#23177,
#23178,#23179),(#23180,#23181,#23182,#23183),(#23184,#23185,#23186,#23187)),
 .UNSPECIFIED.,.F.,.F.,.F.,(4,1,1,4),(4,4),(0.145491947870811,0.633782263373205,
0.816891131686602,1.),(0.0593282329020184,0.895635080262268),
 .UNSPECIFIED.);
#1293=B_SPLINE_SURFACE_WITH_KNOTS('',3,3,((#23203,#23204,#23205,#23206),
(#23207,#23208,#23209,#23210),(#23211,#23212,#23213,#23214),(#23215,#23216,
#23217,#23218)),.UNSPECIFIED.,.F.,.F.,.F.,(4,4),(4,4),(0.,1.),(0.0638119305867452,
0.897818175643156),.UNSPECIFIED.);
#1294=B_SPLINE_SURFACE_WITH_KNOTS('',3,3,((#23237,#23238,#23239,#23240),
(#23241,#23242,#23243,#23244),(#23245,#23246,#23247,#23248),(#23249,#23250,
#23251,#23252),(#23253,#23254,#23255,#23256),(#23257,#23258,#23259,#23260)),
 .UNSPECIFIED.,.F.,.F.,.F.,(4,1,1,4),(4,4),(0.,0.182732451370321,0.365464902740643,
0.852751439728167),(0.0593287711114826,0.895522301354835),.UNSPECIFIED.);
#1295=B_SPLINE_SURFACE_WITH_KNOTS('',3,3,((#23283,#23284,#23285,#23286),
(#23287,#23288,#23289,#23290),(#23291,#23292,#23293,#23294),(#23295,#23296,
#23297,#23298),(#23299,#23300,#23301,#23302),(#23303,#23304,#23305,#23306)),
 .UNSPECIFIED.,.F.,.F.,.F.,(4,1,1,4),(4,4),(0.145491947870803,0.511709684497601,
0.755854842248801,1.),(0.0593282329020183,0.895635080262279),
 .UNSPECIFIED.);
#1296=B_SPLINE_SURFACE_WITH_KNOTS('',3,3,((#23322,#23323,#23324,#23325),
(#23326,#23327,#23328,#23329),(#23330,#23331,#23332,#23333),(#23334,#23335,
#23336,#23337)),.UNSPECIFIED.,.F.,.F.,.F.,(4,4),(4,4),(0.,1.),(0.063811930586745,
0.897818175643157),.UNSPECIFIED.);
#1297=B_SPLINE_SURFACE_WITH_KNOTS('',3,3,((#23356,#23357,#23358,#23359),
(#23360,#23361,#23362,#23363),(#23364,#23365,#23366,#23367),(#23368,#23369,
#23370,#23371),(#23372,#23373,#23374,#23375),(#23376,#23377,#23378,#23379)),
 .UNSPECIFIED.,.F.,.F.,.F.,(4,1,1,4),(4,4),(0.,0.182768423805669,0.365536847611337,
0.852919311093121),(0.0593287711114827,0.895503416457805),.UNSPECIFIED.);
#1298=B_SPLINE_SURFACE_WITH_KNOTS('',3,3,((#23402,#23403,#23404,#23405),
(#23406,#23407,#23408,#23409),(#23410,#23411,#23412,#23413),(#23414,#23415,
#23416,#23417),(#23418,#23419,#23420,#23421),(#23422,#23423,#23424,#23425)),
 .UNSPECIFIED.,.F.,.F.,.F.,(4,1,1,4),(4,4),(0.145491947870775,0.511709684497586,
0.755854842248793,1.),(0.0593282329020186,0.895635080262287),
 .UNSPECIFIED.);
#1299=B_SPLINE_SURFACE_WITH_KNOTS('',3,3,((#23446,#23447,#23448,#23449),
(#23450,#23451,#23452,#23453),(#23454,#23455,#23456,#23457),(#23458,#23459,
#23460,#23461)),.UNSPECIFIED.,.F.,.F.,.F.,(4,4),(4,4),(0.,1.),(0.0638119305867453,
0.897818175643156),.UNSPECIFIED.);
#1300=B_SPLINE_SURFACE_WITH_KNOTS('',3,3,((#23480,#23481,#23482,#23483),
(#23484,#23485,#23486,#23487),(#23488,#23489,#23490,#23491),(#23492,#23493,
#23494,#23495),(#23496,#23497,#23498,#23499),(#23500,#23501,#23502,#23503)),
 .UNSPECIFIED.,.F.,.F.,.F.,(4,1,1,4),(4,4),(0.,0.182732451370321,0.365464902740643,
0.852751439728167),(0.0593287711114827,0.895522301354846),.UNSPECIFIED.);
#1301=B_SPLINE_SURFACE_WITH_KNOTS('',3,3,((#23526,#23527,#23528,#23529),
(#23530,#23531,#23532,#23533),(#23534,#23535,#23536,#23537),(#23538,#23539,
#23540,#23541),(#23542,#23543,#23544,#23545),(#23546,#23547,#23548,#23549)),
 .UNSPECIFIED.,.F.,.F.,.F.,(4,1,1,4),(4,4),(0.145114332397139,0.511493904226937,
0.755746952113468,1.),(0.0593282329032903,0.895635080262252),
 .UNSPECIFIED.);
#1302=B_SPLINE_SURFACE_WITH_KNOTS('',3,3,((#23565,#23566,#23567,#23568),
(#23569,#23570,#23571,#23572),(#23573,#23574,#23575,#23576),(#23577,#23578,
#23579,#23580)),.UNSPECIFIED.,.F.,.F.,.F.,(4,4),(4,4),(0.,1.),(0.0638119305867454,
0.897818175643156),.UNSPECIFIED.);
#1303=B_SPLINE_SURFACE_WITH_KNOTS('',3,3,((#23599,#23600,#23601,#23602),
(#23603,#23604,#23605,#23606),(#23607,#23608,#23609,#23610),(#23611,#23612,
#23613,#23614),(#23615,#23616,#23617,#23618),(#23619,#23620,#23621,#23622)),
 .UNSPECIFIED.,.F.,.F.,.F.,(4,1,1,4),(4,4),(0.,0.182732451370321,0.365464902740643,
0.852751439728166),(0.0593287711114825,0.895522301354846),.UNSPECIFIED.);
#1304=B_SPLINE_SURFACE_WITH_KNOTS('',3,3,((#23645,#23646,#23647,#23648),
(#23649,#23650,#23651,#23652),(#23653,#23654,#23655,#23656),(#23657,#23658,
#23659,#23660),(#23661,#23662,#23663,#23664),(#23665,#23666,#23667,#23668)),
 .UNSPECIFIED.,.F.,.F.,.F.,(4,1,1,4),(4,4),(0.145491947870806,0.511709684497604,
0.755854842248802,1.),(0.0593282329020184,0.895635080262275),
 .UNSPECIFIED.);
#1305=B_SPLINE_SURFACE_WITH_KNOTS('',3,3,((#23684,#23685,#23686,#23687),
(#23688,#23689,#23690,#23691),(#23692,#23693,#23694,#23695),(#23696,#23697,
#23698,#23699)),.UNSPECIFIED.,.F.,.F.,.F.,(4,4),(4,4),(0.,1.),(0.0638119305867451,
0.897818175643157),.UNSPECIFIED.);
#1306=B_SPLINE_SURFACE_WITH_KNOTS('',3,3,((#23718,#23719,#23720,#23721),
(#23722,#23723,#23724,#23725),(#23726,#23727,#23728,#23729),(#23730,#23731,
#23732,#23733),(#23734,#23735,#23736,#23737),(#23738,#23739,#23740,#23741)),
 .UNSPECIFIED.,.F.,.F.,.F.,(4,1,1,4),(4,4),(0.,0.243643268493762,0.487286536987524,
0.852751439728167),(0.0593287711114822,0.895522301354865),.UNSPECIFIED.);
#1307=B_SPLINE_SURFACE_WITH_KNOTS('',3,3,((#23764,#23765,#23766,#23767),
(#23768,#23769,#23770,#23771),(#23772,#23773,#23774,#23775),(#23776,#23777,
#23778,#23779),(#23780,#23781,#23782,#23783),(#23784,#23785,#23786,#23787)),
 .UNSPECIFIED.,.F.,.F.,.F.,(4,1,1,4),(4,4),(0.14549194787082,0.633782263373209,
0.816891131686604,1.),(0.0593282329020183,0.895635080262269),
 .UNSPECIFIED.);
#1308=B_SPLINE_SURFACE_WITH_KNOTS('',3,3,((#23803,#23804,#23805,#23806),
(#23807,#23808,#23809,#23810),(#23811,#23812,#23813,#23814),(#23815,#23816,
#23817,#23818)),.UNSPECIFIED.,.F.,.F.,.F.,(4,4),(4,4),(0.,1.),(0.0638119305867451,
0.897818175643156),.UNSPECIFIED.);
#1309=B_SPLINE_SURFACE_WITH_KNOTS('',3,3,((#23837,#23838,#23839,#23840),
(#23841,#23842,#23843,#23844),(#23845,#23846,#23847,#23848),(#23849,#23850,
#23851,#23852),(#23853,#23854,#23855,#23856),(#23857,#23858,#23859,#23860)),
 .UNSPECIFIED.,.F.,.F.,.F.,(4,1,1,4),(4,4),(0.,0.182732451370321,0.365464902740643,
0.852751439728167),(0.0593287711114825,0.895522301354872),.UNSPECIFIED.);
#1310=B_SPLINE_SURFACE_WITH_KNOTS('',3,3,((#23883,#23884,#23885,#23886),
(#23887,#23888,#23889,#23890),(#23891,#23892,#23893,#23894),(#23895,#23896,
#23897,#23898),(#23899,#23900,#23901,#23902),(#23903,#23904,#23905,#23906)),
 .UNSPECIFIED.,.F.,.F.,.F.,(4,1,1,4),(4,4),(0.145491947870777,0.511709684497587,
0.755854842248793,1.),(0.0593282329020184,0.895635080262259),
 .UNSPECIFIED.);
#1311=B_SPLINE_SURFACE_WITH_KNOTS('',3,3,((#23922,#23923,#23924,#23925),
(#23926,#23927,#23928,#23929),(#23930,#23931,#23932,#23933),(#23934,#23935,
#23936,#23937)),.UNSPECIFIED.,.F.,.F.,.F.,(4,4),(4,4),(0.,1.),(0.0638119305867454,
0.897818175643156),.UNSPECIFIED.);
#1312=B_SPLINE_SURFACE_WITH_KNOTS('',3,3,((#23956,#23957,#23958,#23959),
(#23960,#23961,#23962,#23963),(#23964,#23965,#23966,#23967),(#23968,#23969,
#23970,#23971),(#23972,#23973,#23974,#23975),(#23976,#23977,#23978,#23979)),
 .UNSPECIFIED.,.F.,.F.,.F.,(4,1,1,4),(4,4),(0.,0.182768423805668,0.365536847611337,
0.852919311093119),(0.0593287711114823,0.895503416457802),.UNSPECIFIED.);
#1313=B_SPLINE_SURFACE_WITH_KNOTS('',3,3,((#24002,#24003,#24004,#24005),
(#24006,#24007,#24008,#24009),(#24010,#24011,#24012,#24013),(#24014,#24015,
#24016,#24017),(#24018,#24019,#24020,#24021),(#24022,#24023,#24024,#24025)),
 .UNSPECIFIED.,.F.,.F.,.F.,(4,1,1,4),(4,4),(0.145491947870815,0.511709684497608,
0.755854842248804,1.),(0.0593282329020187,0.895635080262285),
 .UNSPECIFIED.);
#1314=B_SPLINE_SURFACE_WITH_KNOTS('',3,3,((#24041,#24042,#24043,#24044),
(#24045,#24046,#24047,#24048),(#24049,#24050,#24051,#24052),(#24053,#24054,
#24055,#24056)),.UNSPECIFIED.,.F.,.F.,.F.,(4,4),(4,4),(0.,1.),(0.0638119305867453,
0.897818175643157),.UNSPECIFIED.);
#1315=B_SPLINE_SURFACE_WITH_KNOTS('',3,3,((#24075,#24076,#24077,#24078),
(#24079,#24080,#24081,#24082),(#24083,#24084,#24085,#24086),(#24087,#24088,
#24089,#24090),(#24091,#24092,#24093,#24094),(#24095,#24096,#24097,#24098)),
 .UNSPECIFIED.,.F.,.F.,.F.,(4,1,1,4),(4,4),(0.,0.182732451370321,0.365464902740643,
0.852751439728166),(0.0593287711114823,0.895522301354835),.UNSPECIFIED.);
#1316=B_SPLINE_SURFACE_WITH_KNOTS('',3,3,((#24121,#24122,#24123,#24124),
(#24125,#24126,#24127,#24128),(#24129,#24130,#24131,#24132),(#24133,#24134,
#24135,#24136),(#24137,#24138,#24139,#24140),(#24141,#24142,#24143,#24144)),
 .UNSPECIFIED.,.F.,.F.,.F.,(4,1,1,4),(4,4),(0.145114332397162,0.51149390422695,
0.755746952113475,1.),(0.0593282329032904,0.895635080262261),
 .UNSPECIFIED.);
#1317=B_SPLINE_SURFACE_WITH_KNOTS('',3,3,((#24160,#24161,#24162,#24163),
(#24164,#24165,#24166,#24167),(#24168,#24169,#24170,#24171),(#24172,#24173,
#24174,#24175)),.UNSPECIFIED.,.F.,.F.,.F.,(4,4),(4,4),(0.,1.),(0.0638119305867451,
0.897818175643156),.UNSPECIFIED.);
#1318=B_SPLINE_SURFACE_WITH_KNOTS('',3,3,((#24194,#24195,#24196,#24197),
(#24198,#24199,#24200,#24201),(#24202,#24203,#24204,#24205),(#24206,#24207,
#24208,#24209),(#24210,#24211,#24212,#24213),(#24214,#24215,#24216,#24217)),
 .UNSPECIFIED.,.F.,.F.,.F.,(4,1,1,4),(4,4),(0.,0.182732451370321,0.365464902740642,
0.852751439728166),(0.0593287711114828,0.895522301354838),.UNSPECIFIED.);
#1319=B_SPLINE_SURFACE_WITH_KNOTS('',3,3,((#24240,#24241,#24242,#24243),
(#24244,#24245,#24246,#24247),(#24248,#24249,#24250,#24251),(#24252,#24253,
#24254,#24255),(#24256,#24257,#24258,#24259),(#24260,#24261,#24262,#24263)),
 .UNSPECIFIED.,.F.,.F.,.F.,(4,1,1,4),(4,4),(0.1454919478708,0.5117096844976,
0.7558548422488,1.),(0.0593282329020184,0.895635080262241),
 .UNSPECIFIED.);
#1320=B_SPLINE_SURFACE_WITH_KNOTS('',3,3,((#24279,#24280,#24281,#24282),
(#24283,#24284,#24285,#24286),(#24287,#24288,#24289,#24290),(#24291,#24292,
#24293,#24294)),.UNSPECIFIED.,.F.,.F.,.F.,(4,4),(4,4),(0.,1.),(0.0638119305867454,
0.897818175643156),.UNSPECIFIED.);
#1321=B_SPLINE_SURFACE_WITH_KNOTS('',3,3,((#24313,#24314,#24315,#24316),
(#24317,#24318,#24319,#24320),(#24321,#24322,#24323,#24324),(#24325,#24326,
#24327,#24328),(#24329,#24330,#24331,#24332),(#24333,#24334,#24335,#24336)),
 .UNSPECIFIED.,.F.,.F.,.F.,(4,1,1,4),(4,4),(0.,0.182732451370321,0.365464902740643,
0.852751439728166),(0.0593287711114826,0.895522301354858),.UNSPECIFIED.);
#1322=B_SPLINE_SURFACE_WITH_KNOTS('',3,3,((#24359,#24360,#24361,#24362),
(#24363,#24364,#24365,#24366),(#24367,#24368,#24369,#24370),(#24371,#24372,
#24373,#24374),(#24375,#24376,#24377,#24378),(#24379,#24380,#24381,#24382)),
 .UNSPECIFIED.,.F.,.F.,.F.,(4,1,1,4),(4,4),(0.145491947870816,0.511709684497609,
0.755854842248805,1.),(0.0593282329020187,0.89563508026227),
 .UNSPECIFIED.);
#1323=B_SPLINE_SURFACE_WITH_KNOTS('',3,3,((#24398,#24399,#24400,#24401),
(#24402,#24403,#24404,#24405),(#24406,#24407,#24408,#24409),(#24410,#24411,
#24412,#24413)),.UNSPECIFIED.,.F.,.F.,.F.,(4,4),(4,4),(0.,1.),(0.0638119305867453,
0.897818175643156),.UNSPECIFIED.);
#1324=B_SPLINE_SURFACE_WITH_KNOTS('',3,3,((#24432,#24433,#24434,#24435),
(#24436,#24437,#24438,#24439),(#24440,#24441,#24442,#24443),(#24444,#24445,
#24446,#24447),(#24448,#24449,#24450,#24451),(#24452,#24453,#24454,#24455)),
 .UNSPECIFIED.,.F.,.F.,.F.,(4,1,1,4),(4,4),(0.145491947870804,0.511709684497602,
0.755854842248801,1.),(0.0593282329020183,0.895635080262241),
 .UNSPECIFIED.);
#1325=B_SPLINE_SURFACE_WITH_KNOTS('',3,3,((#24471,#24472,#24473,#24474),
(#24475,#24476,#24477,#24478),(#24479,#24480,#24481,#24482),(#24483,#24484,
#24485,#24486)),.UNSPECIFIED.,.F.,.F.,.F.,(4,4),(4,4),(0.,1.),(0.0638119305867451,
0.897818175643156),.UNSPECIFIED.);
#1326=B_SPLINE_SURFACE_WITH_KNOTS('',3,3,((#24501,#24502,#24503,#24504),
(#24505,#24506,#24507,#24508),(#24509,#24510,#24511,#24512),(#24513,#24514,
#24515,#24516),(#24517,#24518,#24519,#24520),(#24521,#24522,#24523,#24524)),
 .UNSPECIFIED.,.F.,.F.,.F.,(4,1,1,4),(4,4),(0.,0.182732451370321,0.365464902740643,
0.852751439728167),(0.0593287711114822,0.895522301354863),.UNSPECIFIED.);
#1327=B_SPLINE_SURFACE_WITH_KNOTS('',3,3,((#24540,#24541,#24542,#24543),
(#24544,#24545,#24546,#24547),(#24548,#24549,#24550,#24551),(#24552,#24553,
#24554,#24555),(#24556,#24557,#24558,#24559),(#24560,#24561,#24562,#24563)),
 .UNSPECIFIED.,.F.,.F.,.F.,(4,1,1,4),(4,4),(0.145491947870802,0.633782263373201,
0.8168911316866,1.),(0.0593282329020185,0.895635080262271),
 .UNSPECIFIED.);
#1328=B_SPLINE_SURFACE_WITH_KNOTS('',3,3,((#24588,#24589,#24590,#24591),
(#24592,#24593,#24594,#24595),(#24596,#24597,#24598,#24599),(#24600,#24601,
#24602,#24603)),.UNSPECIFIED.,.F.,.F.,.F.,(4,4),(4,4),(0.,1.),(0.0638119305867454,
0.897818175643156),.UNSPECIFIED.);
#1329=B_SPLINE_SURFACE_WITH_KNOTS('',3,3,((#24618,#24619,#24620,#24621),
(#24622,#24623,#24624,#24625),(#24626,#24627,#24628,#24629),(#24630,#24631,
#24632,#24633),(#24634,#24635,#24636,#24637),(#24638,#24639,#24640,#24641)),
 .UNSPECIFIED.,.F.,.F.,.F.,(4,1,1,4),(4,4),(0.,0.182767788823199,0.365535577646398,
0.852916347841596),(0.0593287711114826,0.895503517333978),.UNSPECIFIED.);
#1370=FACE_BOUND('',#2876,.T.);
#1371=FACE_BOUND('',#2878,.T.);
#1372=FACE_BOUND('',#2881,.T.);
#1373=FACE_BOUND('',#2882,.T.);
#1374=FACE_BOUND('',#2885,.T.);
#1527=CIRCLE('',#12902,1.);
#1528=CIRCLE('',#12903,1.);
#1529=CIRCLE('',#12904,1.);
#1530=CIRCLE('',#12906,1.);
#1531=CIRCLE('',#12907,1.);
#1532=CIRCLE('',#12911,0.95);
#1533=CIRCLE('',#12913,1.4);
#1534=CIRCLE('',#12914,1.86384419177103);
#1535=CIRCLE('',#12915,1.86384419177103);
#1536=CIRCLE('',#12916,1.86384419177103);
#1537=CIRCLE('',#12917,1.86384419177103);
#1538=CIRCLE('',#12918,1.86384419177103);
#1539=CIRCLE('',#12919,1.86384419177103);
#1540=CIRCLE('',#12920,1.86384419177103);
#1541=CIRCLE('',#12921,1.86384419177103);
#1542=CIRCLE('',#12922,1.86384419177103);
#1543=CIRCLE('',#12923,1.86384419177103);
#1544=CIRCLE('',#12924,1.86384419177103);
#1545=CIRCLE('',#12925,1.86384419177103);
#1546=CIRCLE('',#12926,1.86384419177103);
#1547=CIRCLE('',#12927,1.86384419177103);
#1548=CIRCLE('',#12928,1.86384419177103);
#1549=CIRCLE('',#12929,1.86384419177103);
#1550=CIRCLE('',#12930,1.86384419177103);
#1551=CIRCLE('',#12931,1.86384419177103);
#1552=CIRCLE('',#12932,1.86384419177103);
#1553=CIRCLE('',#12933,1.86384419177103);
#1554=CIRCLE('',#12935,1.2613587668218);
#1555=CIRCLE('',#12937,1.2613587668218);
#1556=CIRCLE('',#12939,1.2613587668218);
#1557=CIRCLE('',#12941,1.2613587668218);
#1558=CIRCLE('',#12943,1.2613587668218);
#1559=CIRCLE('',#12945,1.2613587668218);
#1560=CIRCLE('',#12947,1.2613587668218);
#1561=CIRCLE('',#12949,1.2613587668218);
#1562=CIRCLE('',#12951,1.2613587668218);
#1563=CIRCLE('',#12953,1.2613587668218);
#1564=CIRCLE('',#12955,1.2613587668218);
#1565=CIRCLE('',#12957,1.2613587668218);
#1566=CIRCLE('',#12959,1.2613587668218);
#1567=CIRCLE('',#12961,1.2613587668218);
#1568=CIRCLE('',#12963,1.2613587668218);
#1569=CIRCLE('',#12965,1.2613587668218);
#1570=CIRCLE('',#12967,1.2613587668218);
#1571=CIRCLE('',#12969,1.2613587668218);
#1572=CIRCLE('',#12971,1.2613587668218);
#1573=CIRCLE('',#12973,0.7);
#1574=CIRCLE('',#12974,1.2613587668218);
#1575=CIRCLE('',#12978,0.541);
#1576=CIRCLE('',#12980,0.501);
#1577=CIRCLE('',#12982,0.501);
#1578=CIRCLE('',#12984,0.541);
#2062=FACE_OUTER_BOUND('',#2786,.T.);
#2063=FACE_OUTER_BOUND('',#2787,.T.);
#2064=FACE_OUTER_BOUND('',#2788,.T.);
#2065=FACE_OUTER_BOUND('',#2789,.T.);
#2066=FACE_OUTER_BOUND('',#2790,.T.);
#2067=FACE_OUTER_BOUND('',#2791,.T.);
#2068=FACE_OUTER_BOUND('',#2792,.T.);
#2069=FACE_OUTER_BOUND('',#2793,.T.);
#2070=FACE_OUTER_BOUND('',#2794,.T.);
#2071=FACE_OUTER_BOUND('',#2795,.T.);
#2072=FACE_OUTER_BOUND('',#2796,.T.);
#2073=FACE_OUTER_BOUND('',#2797,.T.);
#2074=FACE_OUTER_BOUND('',#2798,.T.);
#2075=FACE_OUTER_BOUND('',#2799,.T.);
#2076=FACE_OUTER_BOUND('',#2800,.T.);
#2077=FACE_OUTER_BOUND('',#2801,.T.);
#2078=FACE_OUTER_BOUND('',#2802,.T.);
#2079=FACE_OUTER_BOUND('',#2803,.T.);
#2080=FACE_OUTER_BOUND('',#2804,.T.);
#2081=FACE_OUTER_BOUND('',#2805,.T.);
#2082=FACE_OUTER_BOUND('',#2806,.T.);
#2083=FACE_OUTER_BOUND('',#2807,.T.);
#2084=FACE_OUTER_BOUND('',#2808,.T.);
#2085=FACE_OUTER_BOUND('',#2809,.T.);
#2086=FACE_OUTER_BOUND('',#2810,.T.);
#2087=FACE_OUTER_BOUND('',#2811,.T.);
#2088=FACE_OUTER_BOUND('',#2812,.T.);
#2089=FACE_OUTER_BOUND('',#2813,.T.);
#2090=FACE_OUTER_BOUND('',#2814,.T.);
#2091=FACE_OUTER_BOUND('',#2815,.T.);
#2092=FACE_OUTER_BOUND('',#2816,.T.);
#2093=FACE_OUTER_BOUND('',#2817,.T.);
#2094=FACE_OUTER_BOUND('',#2818,.T.);
#2095=FACE_OUTER_BOUND('',#2819,.T.);
#2096=FACE_OUTER_BOUND('',#2820,.T.);
#2097=FACE_OUTER_BOUND('',#2821,.T.);
#2098=FACE_OUTER_BOUND('',#2822,.T.);
#2099=FACE_OUTER_BOUND('',#2823,.T.);
#2100=FACE_OUTER_BOUND('',#2824,.T.);
#2101=FACE_OUTER_BOUND('',#2825,.T.);
#2102=FACE_OUTER_BOUND('',#2826,.T.);
#2103=FACE_OUTER_BOUND('',#2827,.T.);
#2104=FACE_OUTER_BOUND('',#2828,.T.);
#2105=FACE_OUTER_BOUND('',#2829,.T.);
#2106=FACE_OUTER_BOUND('',#2830,.T.);
#2107=FACE_OUTER_BOUND('',#2831,.T.);
#2108=FACE_OUTER_BOUND('',#2832,.T.);
#2109=FACE_OUTER_BOUND('',#2833,.T.);
#2110=FACE_OUTER_BOUND('',#2834,.T.);
#2111=FACE_OUTER_BOUND('',#2835,.T.);
#2112=FACE_OUTER_BOUND('',#2836,.T.);
#2113=FACE_OUTER_BOUND('',#2837,.T.);
#2114=FACE_OUTER_BOUND('',#2838,.T.);
#2115=FACE_OUTER_BOUND('',#2839,.T.);
#2116=FACE_OUTER_BOUND('',#2840,.T.);
#2117=FACE_OUTER_BOUND('',#2841,.T.);
#2118=FACE_OUTER_BOUND('',#2842,.T.);
#2119=FACE_OUTER_BOUND('',#2843,.T.);
#2120=FACE_OUTER_BOUND('',#2844,.T.);
#2121=FACE_OUTER_BOUND('',#2845,.T.);
#2122=FACE_OUTER_BOUND('',#2846,.T.);
#2123=FACE_OUTER_BOUND('',#2847,.T.);
#2124=FACE_OUTER_BOUND('',#2848,.T.);
#2125=FACE_OUTER_BOUND('',#2849,.T.);
#2126=FACE_OUTER_BOUND('',#2850,.T.);
#2127=FACE_OUTER_BOUND('',#2851,.T.);
#2128=FACE_OUTER_BOUND('',#2852,.T.);
#2129=FACE_OUTER_BOUND('',#2853,.T.);
#2130=FACE_OUTER_BOUND('',#2854,.T.);
#2131=FACE_OUTER_BOUND('',#2855,.T.);
#2132=FACE_OUTER_BOUND('',#2856,.T.);
#2133=FACE_OUTER_BOUND('',#2857,.T.);
#2134=FACE_OUTER_BOUND('',#2858,.T.);
#2135=FACE_OUTER_BOUND('',#2859,.T.);
#2136=FACE_OUTER_BOUND('',#2860,.T.);
#2137=FACE_OUTER_BOUND('',#2861,.T.);
#2138=FACE_OUTER_BOUND('',#2862,.T.);
#2139=FACE_OUTER_BOUND('',#2863,.T.);
#2140=FACE_OUTER_BOUND('',#2864,.T.);
#2141=FACE_OUTER_BOUND('',#2865,.T.);
#2142=FACE_OUTER_BOUND('',#2866,.T.);
#2143=FACE_OUTER_BOUND('',#2867,.T.);
#2144=FACE_OUTER_BOUND('',#2868,.T.);
#2145=FACE_OUTER_BOUND('',#2869,.T.);
#2146=FACE_OUTER_BOUND('',#2870,.T.);
#2147=FACE_OUTER_BOUND('',#2871,.T.);
#2148=FACE_OUTER_BOUND('',#2872,.T.);
#2149=FACE_OUTER_BOUND('',#2873,.T.);
#2150=FACE_OUTER_BOUND('',#2874,.T.);
#2151=FACE_OUTER_BOUND('',#2875,.T.);
#2152=FACE_OUTER_BOUND('',#2877,.T.);
#2153=FACE_OUTER_BOUND('',#2879,.T.);
#2154=FACE_OUTER_BOUND('',#2880,.T.);
#2155=FACE_OUTER_BOUND('',#2883,.T.);
#2156=FACE_OUTER_BOUND('',#2884,.T.);
#2786=EDGE_LOOP('',(#9045,#9046,#9047,#9048,#9049,#9050,#9051,#9052,#9053));
#2787=EDGE_LOOP('',(#9054,#9055,#9056,#9057,#9058));
#2788=EDGE_LOOP('',(#9059,#9060,#9061,#9062));
#2789=EDGE_LOOP('',(#9063,#9064,#9065,#9066,#9067,#9068));
#2790=EDGE_LOOP('',(#9069,#9070,#9071,#9072,#9073,#9074,#9075,#9076,#9077));
#2791=EDGE_LOOP('',(#9078,#9079,#9080,#9081,#9082,#9083));
#2792=EDGE_LOOP('',(#9084,#9085,#9086,#9087,#9088,#9089,#9090,#9091,#9092,
#9093));
#2793=EDGE_LOOP('',(#9094,#9095,#9096,#9097));
#2794=EDGE_LOOP('',(#9098,#9099,#9100,#9101));
#2795=EDGE_LOOP('',(#9102,#9103,#9104,#9105));
#2796=EDGE_LOOP('',(#9106,#9107,#9108,#9109,#9110,#9111,#9112,#9113,#9114,
#9115,#9116,#9117,#9118,#9119,#9120,#9121,#9122,#9123,#9124,#9125,#9126,
#9127,#9128,#9129,#9130,#9131,#9132,#9133,#9134,#9135,#9136,#9137,#9138,
#9139,#9140,#9141,#9142,#9143,#9144,#9145,#9146,#9147,#9148,#9149,#9150,
#9151,#9152,#9153,#9154,#9155,#9156,#9157,#9158,#9159,#9160,#9161,#9162,
#9163,#9164,#9165,#9166,#9167,#9168,#9169,#9170,#9171,#9172,#9173,#9174,
#9175,#9176,#9177,#9178,#9179,#9180,#9181,#9182,#9183,#9184,#9185,#9186,
#9187,#9188,#9189));
#2797=EDGE_LOOP('',(#9190,#9191,#9192,#9193));
#2798=EDGE_LOOP('',(#9194,#9195,#9196,#9197));
#2799=EDGE_LOOP('',(#9198,#9199,#9200,#9201));
#2800=EDGE_LOOP('',(#9202,#9203,#9204,#9205));
#2801=EDGE_LOOP('',(#9206,#9207,#9208,#9209));
#2802=EDGE_LOOP('',(#9210,#9211,#9212,#9213));
#2803=EDGE_LOOP('',(#9214,#9215,#9216,#9217));
#2804=EDGE_LOOP('',(#9218,#9219,#9220,#9221));
#2805=EDGE_LOOP('',(#9222,#9223,#9224,#9225));
#2806=EDGE_LOOP('',(#9226,#9227,#9228,#9229));
#2807=EDGE_LOOP('',(#9230,#9231,#9232,#9233));
#2808=EDGE_LOOP('',(#9234,#9235,#9236,#9237));
#2809=EDGE_LOOP('',(#9238,#9239,#9240,#9241));
#2810=EDGE_LOOP('',(#9242,#9243,#9244,#9245));
#2811=EDGE_LOOP('',(#9246,#9247,#9248,#9249));
#2812=EDGE_LOOP('',(#9250,#9251,#9252,#9253));
#2813=EDGE_LOOP('',(#9254,#9255,#9256,#9257));
#2814=EDGE_LOOP('',(#9258,#9259,#9260,#9261));
#2815=EDGE_LOOP('',(#9262,#9263,#9264,#9265));
#2816=EDGE_LOOP('',(#9266,#9267,#9268,#9269));
#2817=EDGE_LOOP('',(#9270,#9271,#9272,#9273));
#2818=EDGE_LOOP('',(#9274,#9275,#9276,#9277));
#2819=EDGE_LOOP('',(#9278,#9279,#9280,#9281));
#2820=EDGE_LOOP('',(#9282,#9283,#9284,#9285));
#2821=EDGE_LOOP('',(#9286,#9287,#9288,#9289));
#2822=EDGE_LOOP('',(#9290,#9291,#9292,#9293));
#2823=EDGE_LOOP('',(#9294,#9295,#9296,#9297));
#2824=EDGE_LOOP('',(#9298,#9299,#9300,#9301));
#2825=EDGE_LOOP('',(#9302,#9303,#9304,#9305));
#2826=EDGE_LOOP('',(#9306,#9307,#9308,#9309));
#2827=EDGE_LOOP('',(#9310,#9311,#9312,#9313));
#2828=EDGE_LOOP('',(#9314,#9315,#9316,#9317));
#2829=EDGE_LOOP('',(#9318,#9319,#9320,#9321));
#2830=EDGE_LOOP('',(#9322,#9323,#9324,#9325));
#2831=EDGE_LOOP('',(#9326,#9327,#9328,#9329));
#2832=EDGE_LOOP('',(#9330,#9331,#9332,#9333,#9334));
#2833=EDGE_LOOP('',(#9335,#9336,#9337,#9338));
#2834=EDGE_LOOP('',(#9339,#9340,#9341,#9342));
#2835=EDGE_LOOP('',(#9343,#9344,#9345,#9346));
#2836=EDGE_LOOP('',(#9347,#9348,#9349,#9350,#9351));
#2837=EDGE_LOOP('',(#9352,#9353,#9354,#9355));
#2838=EDGE_LOOP('',(#9356,#9357,#9358,#9359));
#2839=EDGE_LOOP('',(#9360,#9361,#9362,#9363));
#2840=EDGE_LOOP('',(#9364,#9365,#9366,#9367));
#2841=EDGE_LOOP('',(#9368,#9369,#9370,#9371));
#2842=EDGE_LOOP('',(#9372,#9373,#9374,#9375));
#2843=EDGE_LOOP('',(#9376,#9377,#9378,#9379));
#2844=EDGE_LOOP('',(#9380,#9381,#9382,#9383));
#2845=EDGE_LOOP('',(#9384,#9385,#9386,#9387));
#2846=EDGE_LOOP('',(#9388,#9389,#9390,#9391));
#2847=EDGE_LOOP('',(#9392,#9393,#9394,#9395));
#2848=EDGE_LOOP('',(#9396,#9397,#9398,#9399));
#2849=EDGE_LOOP('',(#9400,#9401,#9402,#9403));
#2850=EDGE_LOOP('',(#9404,#9405,#9406,#9407));
#2851=EDGE_LOOP('',(#9408,#9409,#9410,#9411));
#2852=EDGE_LOOP('',(#9412,#9413,#9414,#9415));
#2853=EDGE_LOOP('',(#9416,#9417,#9418,#9419));
#2854=EDGE_LOOP('',(#9420,#9421,#9422,#9423));
#2855=EDGE_LOOP('',(#9424,#9425,#9426,#9427));
#2856=EDGE_LOOP('',(#9428,#9429,#9430,#9431));
#2857=EDGE_LOOP('',(#9432,#9433,#9434,#9435));
#2858=EDGE_LOOP('',(#9436,#9437,#9438,#9439));
#2859=EDGE_LOOP('',(#9440,#9441,#9442,#9443));
#2860=EDGE_LOOP('',(#9444,#9445,#9446,#9447));
#2861=EDGE_LOOP('',(#9448,#9449,#9450,#9451));
#2862=EDGE_LOOP('',(#9452,#9453,#9454,#9455));
#2863=EDGE_LOOP('',(#9456,#9457,#9458,#9459));
#2864=EDGE_LOOP('',(#9460,#9461,#9462,#9463));
#2865=EDGE_LOOP('',(#9464,#9465,#9466,#9467));
#2866=EDGE_LOOP('',(#9468,#9469,#9470,#9471));
#2867=EDGE_LOOP('',(#9472,#9473,#9474,#9475));
#2868=EDGE_LOOP('',(#9476,#9477,#9478,#9479));
#2869=EDGE_LOOP('',(#9480,#9481,#9482,#9483));
#2870=EDGE_LOOP('',(#9484,#9485,#9486,#9487));
#2871=EDGE_LOOP('',(#9488,#9489,#9490,#9491));
#2872=EDGE_LOOP('',(#9492,#9493,#9494,#9495));
#2873=EDGE_LOOP('',(#9496,#9497,#9498,#9499,#9500,#9501,#9502,#9503,#9504,
#9505,#9506,#9507,#9508,#9509,#9510,#9511,#9512,#9513,#9514,#9515,#9516,
#9517,#9518,#9519,#9520,#9521,#9522,#9523,#9524,#9525,#9526,#9527,#9528,
#9529,#9530,#9531,#9532,#9533,#9534,#9535,#9536,#9537,#9538,#9539,#9540,
#9541,#9542,#9543,#9544,#9545,#9546,#9547,#9548,#9549,#9550,#9551,#9552,
#9553,#9554,#9555,#9556,#9557,#9558,#9559,#9560,#9561,#9562,#9563,#9564,
#9565,#9566,#9567,#9568,#9569,#9570,#9571,#9572,#9573,#9574,#9575,#9576,
#9577,#9578,#9579));
#2874=EDGE_LOOP('',(#9580,#9581,#9582,#9583));
#2875=EDGE_LOOP('',(#9584));
#2876=EDGE_LOOP('',(#9585,#9586,#9587,#9588));
#2877=EDGE_LOOP('',(#9589));
#2878=EDGE_LOOP('',(#9590));
#2879=EDGE_LOOP('',(#9591,#9592,#9593,#9594));
#2880=EDGE_LOOP('',(#9595,#9596,#9597,#9598));
#2881=EDGE_LOOP('',(#9599,#9600));
#2882=EDGE_LOOP('',(#9601,#9602));
#2883=EDGE_LOOP('',(#9603,#9604,#9605,#9606));
#2884=EDGE_LOOP('',(#9607));
#2885=EDGE_LOOP('',(#9608));
#3530=LINE('',#21440,#4235);
#3531=LINE('',#21731,#4236);
#3532=LINE('',#21735,#4237);
#3533=LINE('',#21882,#4238);
#3534=LINE('',#24651,#4239);
#3535=LINE('',#24660,#4240);
#3536=LINE('',#24664,#4241);
#3537=LINE('',#24668,#4242);
#4235=VECTOR('',#14470,0.205);
#4236=VECTOR('',#14473,0.205);
#4237=VECTOR('',#14478,0.975);
#4238=VECTOR('',#14483,1.63192209588552);
#4239=VECTOR('',#14604,0.980679383410898);
#4240=VECTOR('',#14617,0.521);
#4241=VECTOR('',#14622,0.501);
#4242=VECTOR('',#14627,0.521);
#5101=VERTEX_POINT('',#21268);
#5102=VERTEX_POINT('',#21269);
#5103=VERTEX_POINT('',#21304);
#5104=VERTEX_POINT('',#21319);
#5105=VERTEX_POINT('',#21332);
#5106=VERTEX_POINT('',#21337);
#5107=VERTEX_POINT('',#21371);
#5108=VERTEX_POINT('',#21401);
#5109=VERTEX_POINT('',#21403);
#5110=VERTEX_POINT('',#21405);
#5111=VERTEX_POINT('',#21420);
#5112=VERTEX_POINT('',#21422);
#5113=VERTEX_POINT('',#21439);
#5114=VERTEX_POINT('',#21441);
#5115=VERTEX_POINT('',#21627);
#5116=VERTEX_POINT('',#21640);
#5117=VERTEX_POINT('',#21645);
#5118=VERTEX_POINT('',#21693);
#5119=VERTEX_POINT('',#21694);
#5120=VERTEX_POINT('',#21733);
#5121=VERTEX_POINT('',#21760);
#5122=VERTEX_POINT('',#21761);
#5123=VERTEX_POINT('',#21768);
#5124=VERTEX_POINT('',#21775);
#5125=VERTEX_POINT('',#21816);
#5126=VERTEX_POINT('',#21817);
#5127=VERTEX_POINT('',#21826);
#5128=VERTEX_POINT('',#21835);
#5129=VERTEX_POINT('',#21879);
#5130=VERTEX_POINT('',#21881);
#5131=VERTEX_POINT('',#21883);
#5132=VERTEX_POINT('',#21888);
#5133=VERTEX_POINT('',#21890);
#5134=VERTEX_POINT('',#21899);
#5135=VERTEX_POINT('',#21907);
#5136=VERTEX_POINT('',#21914);
#5137=VERTEX_POINT('',#21916);
#5138=VERTEX_POINT('',#21925);
#5139=VERTEX_POINT('',#21933);
#5140=VERTEX_POINT('',#21940);
#5141=VERTEX_POINT('',#21942);
#5142=VERTEX_POINT('',#21951);
#5143=VERTEX_POINT('',#21959);
#5144=VERTEX_POINT('',#21966);
#5145=VERTEX_POINT('',#21968);
#5146=VERTEX_POINT('',#21977);
#5147=VERTEX_POINT('',#21985);
#5148=VERTEX_POINT('',#21992);
#5149=VERTEX_POINT('',#21994);
#5150=VERTEX_POINT('',#22003);
#5151=VERTEX_POINT('',#22011);
#5152=VERTEX_POINT('',#22018);
#5153=VERTEX_POINT('',#22020);
#5154=VERTEX_POINT('',#22029);
#5155=VERTEX_POINT('',#22037);
#5156=VERTEX_POINT('',#22044);
#5157=VERTEX_POINT('',#22046);
#5158=VERTEX_POINT('',#22055);
#5159=VERTEX_POINT('',#22063);
#5160=VERTEX_POINT('',#22070);
#5161=VERTEX_POINT('',#22072);
#5162=VERTEX_POINT('',#22081);
#5163=VERTEX_POINT('',#22089);
#5164=VERTEX_POINT('',#22096);
#5165=VERTEX_POINT('',#22098);
#5166=VERTEX_POINT('',#22107);
#5167=VERTEX_POINT('',#22115);
#5168=VERTEX_POINT('',#22123);
#5169=VERTEX_POINT('',#22125);
#5170=VERTEX_POINT('',#22134);
#5171=VERTEX_POINT('',#22142);
#5172=VERTEX_POINT('',#22149);
#5173=VERTEX_POINT('',#22151);
#5174=VERTEX_POINT('',#22160);
#5175=VERTEX_POINT('',#22168);
#5176=VERTEX_POINT('',#22175);
#5177=VERTEX_POINT('',#22177);
#5178=VERTEX_POINT('',#22186);
#5179=VERTEX_POINT('',#22194);
#5180=VERTEX_POINT('',#22201);
#5181=VERTEX_POINT('',#22203);
#5182=VERTEX_POINT('',#22212);
#5183=VERTEX_POINT('',#22220);
#5184=VERTEX_POINT('',#22227);
#5185=VERTEX_POINT('',#22229);
#5186=VERTEX_POINT('',#22238);
#5187=VERTEX_POINT('',#22246);
#5188=VERTEX_POINT('',#22253);
#5189=VERTEX_POINT('',#22255);
#5190=VERTEX_POINT('',#22264);
#5191=VERTEX_POINT('',#22272);
#5192=VERTEX_POINT('',#22279);
#5193=VERTEX_POINT('',#22281);
#5194=VERTEX_POINT('',#22290);
#5195=VERTEX_POINT('',#22298);
#5196=VERTEX_POINT('',#22305);
#5197=VERTEX_POINT('',#22307);
#5198=VERTEX_POINT('',#22316);
#5199=VERTEX_POINT('',#22324);
#5200=VERTEX_POINT('',#22331);
#5201=VERTEX_POINT('',#22333);
#5202=VERTEX_POINT('',#22342);
#5203=VERTEX_POINT('',#22350);
#5204=VERTEX_POINT('',#22357);
#5205=VERTEX_POINT('',#22359);
#5206=VERTEX_POINT('',#22368);
#5207=VERTEX_POINT('',#22383);
#5208=VERTEX_POINT('',#22394);
#5209=VERTEX_POINT('',#22428);
#5210=VERTEX_POINT('',#22429);
#5211=VERTEX_POINT('',#22474);
#5212=VERTEX_POINT('',#22513);
#5213=VERTEX_POINT('',#22547);
#5214=VERTEX_POINT('',#22548);
#5215=VERTEX_POINT('',#22593);
#5216=VERTEX_POINT('',#22632);
#5217=VERTEX_POINT('',#22666);
#5218=VERTEX_POINT('',#22667);
#5219=VERTEX_POINT('',#22712);
#5220=VERTEX_POINT('',#22751);
#5221=VERTEX_POINT('',#22785);
#5222=VERTEX_POINT('',#22786);
#5223=VERTEX_POINT('',#22831);
#5224=VERTEX_POINT('',#22870);
#5225=VERTEX_POINT('',#22904);
#5226=VERTEX_POINT('',#22905);
#5227=VERTEX_POINT('',#22950);
#5228=VERTEX_POINT('',#22989);
#5229=VERTEX_POINT('',#23023);
#5230=VERTEX_POINT('',#23024);
#5231=VERTEX_POINT('',#23069);
#5232=VERTEX_POINT('',#23108);
#5233=VERTEX_POINT('',#23142);
#5234=VERTEX_POINT('',#23143);
#5235=VERTEX_POINT('',#23188);
#5236=VERTEX_POINT('',#23227);
#5237=VERTEX_POINT('',#23261);
#5238=VERTEX_POINT('',#23262);
#5239=VERTEX_POINT('',#23307);
#5240=VERTEX_POINT('',#23346);
#5241=VERTEX_POINT('',#23380);
#5242=VERTEX_POINT('',#23381);
#5243=VERTEX_POINT('',#23426);
#5244=VERTEX_POINT('',#23431);
#5245=VERTEX_POINT('',#23470);
#5246=VERTEX_POINT('',#23504);
#5247=VERTEX_POINT('',#23505);
#5248=VERTEX_POINT('',#23550);
#5249=VERTEX_POINT('',#23589);
#5250=VERTEX_POINT('',#23623);
#5251=VERTEX_POINT('',#23624);
#5252=VERTEX_POINT('',#23669);
#5253=VERTEX_POINT('',#23708);
#5254=VERTEX_POINT('',#23742);
#5255=VERTEX_POINT('',#23743);
#5256=VERTEX_POINT('',#23788);
#5257=VERTEX_POINT('',#23827);
#5258=VERTEX_POINT('',#23861);
#5259=VERTEX_POINT('',#23862);
#5260=VERTEX_POINT('',#23907);
#5261=VERTEX_POINT('',#23946);
#5262=VERTEX_POINT('',#23980);
#5263=VERTEX_POINT('',#23981);
#5264=VERTEX_POINT('',#24026);
#5265=VERTEX_POINT('',#24065);
#5266=VERTEX_POINT('',#24099);
#5267=VERTEX_POINT('',#24100);
#5268=VERTEX_POINT('',#24145);
#5269=VERTEX_POINT('',#24184);
#5270=VERTEX_POINT('',#24218);
#5271=VERTEX_POINT('',#24219);
#5272=VERTEX_POINT('',#24264);
#5273=VERTEX_POINT('',#24303);
#5274=VERTEX_POINT('',#24337);
#5275=VERTEX_POINT('',#24338);
#5276=VERTEX_POINT('',#24383);
#5277=VERTEX_POINT('',#24422);
#5278=VERTEX_POINT('',#24456);
#5279=VERTEX_POINT('',#24487);
#5280=VERTEX_POINT('',#24525);
#5281=VERTEX_POINT('',#24564);
#5282=VERTEX_POINT('',#24571);
#5283=VERTEX_POINT('',#24604);
#5284=VERTEX_POINT('',#24649);
#5285=VERTEX_POINT('',#24656);
#5286=VERTEX_POINT('',#24659);
#5287=VERTEX_POINT('',#24663);
#5288=VERTEX_POINT('',#24667);
#6534=EDGE_CURVE('',#5101,#5102,#723,.T.);
#6535=EDGE_CURVE('',#5101,#5103,#724,.T.);
#6536=EDGE_CURVE('',#5103,#5104,#725,.T.);
#6537=EDGE_CURVE('',#5104,#5105,#726,.T.);
#6538=EDGE_CURVE('',#5105,#5106,#727,.T.);
#6539=EDGE_CURVE('',#5106,#5105,#728,.T.);
#6540=EDGE_CURVE('',#5104,#5107,#729,.T.);
#6541=EDGE_CURVE('',#5107,#5102,#730,.T.);
#6542=EDGE_CURVE('',#5108,#5107,#1527,.T.);
#6543=EDGE_CURVE('',#5109,#5108,#1528,.T.);
#6544=EDGE_CURVE('',#5110,#5109,#731,.T.);
#6545=EDGE_CURVE('',#5110,#5102,#1529,.T.);
#6546=EDGE_CURVE('',#5101,#5111,#1530,.T.);
#6547=EDGE_CURVE('',#5112,#5111,#732,.T.);
#6548=EDGE_CURVE('',#5103,#5112,#1531,.T.);
#6549=EDGE_CURVE('',#5106,#5113,#3530,.T.);
#6550=EDGE_CURVE('',#5114,#5113,#733,.T.);
#6551=EDGE_CURVE('',#5113,#5114,#734,.T.);
#6552=EDGE_CURVE('',#5110,#5111,#735,.T.);
#6553=EDGE_CURVE('',#5109,#5115,#736,.T.);
#6554=EDGE_CURVE('',#5115,#5116,#737,.T.);
#6555=EDGE_CURVE('',#5116,#5117,#738,.T.);
#6556=EDGE_CURVE('',#5117,#5116,#739,.T.);
#6557=EDGE_CURVE('',#5115,#5112,#740,.T.);
#6558=EDGE_CURVE('',#5118,#5119,#741,.T.);
#6559=EDGE_CURVE('',#5119,#5118,#742,.T.);
#6560=EDGE_CURVE('',#5119,#5117,#3531,.T.);
#6561=EDGE_CURVE('',#5120,#5120,#1532,.T.);
#6562=EDGE_CURVE('',#5120,#5108,#3532,.T.);
#6563=EDGE_CURVE('',#5121,#5122,#743,.T.);
#6564=EDGE_CURVE('',#5121,#5123,#744,.T.);
#6565=EDGE_CURVE('',#5124,#5123,#745,.T.);
#6566=EDGE_CURVE('',#5122,#5124,#746,.T.);
#6567=EDGE_CURVE('',#5125,#5126,#747,.T.);
#6568=EDGE_CURVE('',#5127,#5125,#748,.T.);
#6569=EDGE_CURVE('',#5128,#5127,#749,.T.);
#6570=EDGE_CURVE('',#5126,#5128,#750,.T.);
#6571=EDGE_CURVE('',#5126,#5121,#751,.T.);
#6572=EDGE_CURVE('',#5123,#5128,#752,.T.);
#6573=EDGE_CURVE('',#5129,#5129,#1533,.T.);
#6574=EDGE_CURVE('',#5129,#5130,#3533,.T.);
#6575=EDGE_CURVE('',#5130,#5131,#753,.T.);
#6576=EDGE_CURVE('',#5131,#5132,#1534,.T.);
#6577=EDGE_CURVE('',#5132,#5133,#754,.T.);
#6578=EDGE_CURVE('',#5133,#5134,#755,.T.);
#6579=EDGE_CURVE('',#5134,#5135,#756,.T.);
#6580=EDGE_CURVE('',#5135,#5136,#1535,.T.);
#6581=EDGE_CURVE('',#5136,#5137,#757,.T.);
#6582=EDGE_CURVE('',#5137,#5138,#758,.T.);
#6583=EDGE_CURVE('',#5138,#5139,#759,.T.);
#6584=EDGE_CURVE('',#5139,#5140,#1536,.T.);
#6585=EDGE_CURVE('',#5140,#5141,#760,.T.);
#6586=EDGE_CURVE('',#5141,#5142,#761,.T.);
#6587=EDGE_CURVE('',#5142,#5143,#762,.T.);
#6588=EDGE_CURVE('',#5143,#5144,#1537,.T.);
#6589=EDGE_CURVE('',#5144,#5145,#763,.T.);
#6590=EDGE_CURVE('',#5145,#5146,#764,.T.);
#6591=EDGE_CURVE('',#5146,#5147,#765,.T.);
#6592=EDGE_CURVE('',#5147,#5148,#1538,.T.);
#6593=EDGE_CURVE('',#5148,#5149,#766,.T.);
#6594=EDGE_CURVE('',#5149,#5150,#767,.T.);
#6595=EDGE_CURVE('',#5150,#5151,#768,.T.);
#6596=EDGE_CURVE('',#5151,#5152,#1539,.T.);
#6597=EDGE_CURVE('',#5152,#5153,#769,.T.);
#6598=EDGE_CURVE('',#5153,#5154,#770,.T.);
#6599=EDGE_CURVE('',#5154,#5155,#771,.T.);
#6600=EDGE_CURVE('',#5155,#5156,#1540,.T.);
#6601=EDGE_CURVE('',#5156,#5157,#772,.T.);
#6602=EDGE_CURVE('',#5157,#5158,#773,.T.);
#6603=EDGE_CURVE('',#5158,#5159,#774,.T.);
#6604=EDGE_CURVE('',#5159,#5160,#1541,.T.);
#6605=EDGE_CURVE('',#5160,#5161,#775,.T.);
#6606=EDGE_CURVE('',#5161,#5162,#776,.T.);
#6607=EDGE_CURVE('',#5162,#5163,#777,.T.);
#6608=EDGE_CURVE('',#5163,#5164,#1542,.T.);
#6609=EDGE_CURVE('',#5164,#5165,#778,.T.);
#6610=EDGE_CURVE('',#5165,#5166,#779,.T.);
#6611=EDGE_CURVE('',#5166,#5167,#780,.T.);
#6612=EDGE_CURVE('',#5167,#5124,#1543,.T.);
#6613=EDGE_CURVE('',#5127,#5168,#1544,.T.);
#6614=EDGE_CURVE('',#5168,#5169,#781,.T.);
#6615=EDGE_CURVE('',#5169,#5170,#782,.T.);
#6616=EDGE_CURVE('',#5170,#5171,#783,.T.);
#6617=EDGE_CURVE('',#5171,#5172,#1545,.T.);
#6618=EDGE_CURVE('',#5172,#5173,#784,.T.);
#6619=EDGE_CURVE('',#5173,#5174,#785,.T.);
#6620=EDGE_CURVE('',#5174,#5175,#786,.T.);
#6621=EDGE_CURVE('',#5175,#5176,#1546,.T.);
#6622=EDGE_CURVE('',#5176,#5177,#787,.T.);
#6623=EDGE_CURVE('',#5177,#5178,#788,.T.);
#6624=EDGE_CURVE('',#5178,#5179,#789,.T.);
#6625=EDGE_CURVE('',#5179,#5180,#1547,.T.);
#6626=EDGE_CURVE('',#5180,#5181,#790,.T.);
#6627=EDGE_CURVE('',#5181,#5182,#791,.T.);
#6628=EDGE_CURVE('',#5182,#5183,#792,.T.);
#6629=EDGE_CURVE('',#5183,#5184,#1548,.T.);
#6630=EDGE_CURVE('',#5184,#5185,#793,.T.);
#6631=EDGE_CURVE('',#5185,#5186,#794,.T.);
#6632=EDGE_CURVE('',#5186,#5187,#795,.T.);
#6633=EDGE_CURVE('',#5187,#5188,#1549,.T.);
#6634=EDGE_CURVE('',#5188,#5189,#796,.T.);
#6635=EDGE_CURVE('',#5189,#5190,#797,.T.);
#6636=EDGE_CURVE('',#5190,#5191,#798,.T.);
#6637=EDGE_CURVE('',#5191,#5192,#1550,.T.);
#6638=EDGE_CURVE('',#5192,#5193,#799,.T.);
#6639=EDGE_CURVE('',#5193,#5194,#800,.T.);
#6640=EDGE_CURVE('',#5194,#5195,#801,.T.);
#6641=EDGE_CURVE('',#5195,#5196,#1551,.T.);
#6642=EDGE_CURVE('',#5196,#5197,#802,.T.);
#6643=EDGE_CURVE('',#5197,#5198,#803,.T.);
#6644=EDGE_CURVE('',#5198,#5199,#804,.T.);
#6645=EDGE_CURVE('',#5199,#5200,#1552,.T.);
#6646=EDGE_CURVE('',#5200,#5201,#805,.T.);
#6647=EDGE_CURVE('',#5201,#5202,#806,.T.);
#6648=EDGE_CURVE('',#5202,#5203,#807,.T.);
#6649=EDGE_CURVE('',#5203,#5204,#1553,.T.);
#6650=EDGE_CURVE('',#5204,#5205,#808,.T.);
#6651=EDGE_CURVE('',#5205,#5206,#809,.T.);
#6652=EDGE_CURVE('',#5206,#5130,#810,.T.);
#6653=EDGE_CURVE('',#5125,#5207,#1554,.T.);
#6654=EDGE_CURVE('',#5207,#5168,#811,.T.);
#6655=EDGE_CURVE('',#5167,#5208,#812,.T.);
#6656=EDGE_CURVE('',#5208,#5122,#1555,.T.);
#6657=EDGE_CURVE('',#5209,#5210,#813,.T.);
#6658=EDGE_CURVE('',#5209,#5165,#814,.T.);
#6659=EDGE_CURVE('',#5210,#5164,#815,.T.);
#6660=EDGE_CURVE('',#5208,#5211,#816,.T.);
#6661=EDGE_CURVE('',#5211,#5166,#817,.T.);
#6662=EDGE_CURVE('',#5211,#5209,#818,.T.);
#6663=EDGE_CURVE('',#5163,#5212,#819,.T.);
#6664=EDGE_CURVE('',#5212,#5210,#1556,.T.);
#6665=EDGE_CURVE('',#5213,#5214,#820,.T.);
#6666=EDGE_CURVE('',#5213,#5161,#821,.T.);
#6667=EDGE_CURVE('',#5214,#5160,#822,.T.);
#6668=EDGE_CURVE('',#5212,#5215,#823,.T.);
#6669=EDGE_CURVE('',#5215,#5162,#824,.T.);
#6670=EDGE_CURVE('',#5215,#5213,#825,.T.);
#6671=EDGE_CURVE('',#5159,#5216,#826,.T.);
#6672=EDGE_CURVE('',#5216,#5214,#1557,.T.);
#6673=EDGE_CURVE('',#5217,#5218,#827,.T.);
#6674=EDGE_CURVE('',#5217,#5157,#828,.T.);
#6675=EDGE_CURVE('',#5218,#5156,#829,.T.);
#6676=EDGE_CURVE('',#5216,#5219,#830,.T.);
#6677=EDGE_CURVE('',#5219,#5158,#831,.T.);
#6678=EDGE_CURVE('',#5219,#5217,#832,.T.);
#6679=EDGE_CURVE('',#5155,#5220,#833,.T.);
#6680=EDGE_CURVE('',#5220,#5218,#1558,.T.);
#6681=EDGE_CURVE('',#5221,#5222,#834,.T.);
#6682=EDGE_CURVE('',#5221,#5153,#835,.T.);
#6683=EDGE_CURVE('',#5222,#5152,#836,.T.);
#6684=EDGE_CURVE('',#5220,#5223,#837,.T.);
#6685=EDGE_CURVE('',#5223,#5154,#838,.T.);
#6686=EDGE_CURVE('',#5223,#5221,#839,.T.);
#6687=EDGE_CURVE('',#5151,#5224,#840,.T.);
#6688=EDGE_CURVE('',#5224,#5222,#1559,.T.);
#6689=EDGE_CURVE('',#5225,#5226,#841,.T.);
#6690=EDGE_CURVE('',#5225,#5149,#842,.T.);
#6691=EDGE_CURVE('',#5226,#5148,#843,.T.);
#6692=EDGE_CURVE('',#5224,#5227,#844,.T.);
#6693=EDGE_CURVE('',#5227,#5150,#845,.T.);
#6694=EDGE_CURVE('',#5227,#5225,#846,.T.);
#6695=EDGE_CURVE('',#5147,#5228,#847,.T.);
#6696=EDGE_CURVE('',#5228,#5226,#1560,.T.);
#6697=EDGE_CURVE('',#5229,#5230,#848,.T.);
#6698=EDGE_CURVE('',#5229,#5145,#849,.T.);
#6699=EDGE_CURVE('',#5230,#5144,#850,.T.);
#6700=EDGE_CURVE('',#5228,#5231,#851,.T.);
#6701=EDGE_CURVE('',#5231,#5146,#852,.T.);
#6702=EDGE_CURVE('',#5231,#5229,#853,.T.);
#6703=EDGE_CURVE('',#5143,#5232,#854,.T.);
#6704=EDGE_CURVE('',#5232,#5230,#1561,.T.);
#6705=EDGE_CURVE('',#5233,#5234,#855,.T.);
#6706=EDGE_CURVE('',#5233,#5141,#856,.T.);
#6707=EDGE_CURVE('',#5234,#5140,#857,.T.);
#6708=EDGE_CURVE('',#5232,#5235,#858,.T.);
#6709=EDGE_CURVE('',#5235,#5142,#859,.T.);
#6710=EDGE_CURVE('',#5235,#5233,#860,.T.);
#6711=EDGE_CURVE('',#5139,#5236,#861,.T.);
#6712=EDGE_CURVE('',#5236,#5234,#1562,.T.);
#6713=EDGE_CURVE('',#5237,#5238,#862,.T.);
#6714=EDGE_CURVE('',#5237,#5137,#863,.T.);
#6715=EDGE_CURVE('',#5238,#5136,#864,.T.);
#6716=EDGE_CURVE('',#5236,#5239,#865,.T.);
#6717=EDGE_CURVE('',#5239,#5138,#866,.T.);
#6718=EDGE_CURVE('',#5239,#5237,#867,.T.);
#6719=EDGE_CURVE('',#5135,#5240,#868,.T.);
#6720=EDGE_CURVE('',#5240,#5238,#1563,.T.);
#6721=EDGE_CURVE('',#5241,#5242,#869,.T.);
#6722=EDGE_CURVE('',#5241,#5133,#870,.T.);
#6723=EDGE_CURVE('',#5242,#5132,#871,.T.);
#6724=EDGE_CURVE('',#5240,#5243,#872,.T.);
#6725=EDGE_CURVE('',#5244,#5134,#873,.T.);
#6726=EDGE_CURVE('',#5243,#5244,#874,.T.);
#6727=EDGE_CURVE('',#5244,#5241,#875,.T.);
#6728=EDGE_CURVE('',#5131,#5245,#876,.T.);
#6729=EDGE_CURVE('',#5245,#5242,#1564,.T.);
#6730=EDGE_CURVE('',#5246,#5247,#877,.T.);
#6731=EDGE_CURVE('',#5246,#5205,#878,.T.);
#6732=EDGE_CURVE('',#5247,#5204,#879,.T.);
#6733=EDGE_CURVE('',#5245,#5248,#880,.T.);
#6734=EDGE_CURVE('',#5248,#5206,#881,.T.);
#6735=EDGE_CURVE('',#5248,#5246,#882,.T.);
#6736=EDGE_CURVE('',#5203,#5249,#883,.T.);
#6737=EDGE_CURVE('',#5249,#5247,#1565,.T.);
#6738=EDGE_CURVE('',#5250,#5251,#884,.T.);
#6739=EDGE_CURVE('',#5250,#5201,#885,.T.);
#6740=EDGE_CURVE('',#5251,#5200,#886,.T.);
#6741=EDGE_CURVE('',#5249,#5252,#887,.T.);
#6742=EDGE_CURVE('',#5252,#5202,#888,.T.);
#6743=EDGE_CURVE('',#5252,#5250,#889,.T.);
#6744=EDGE_CURVE('',#5199,#5253,#890,.T.);
#6745=EDGE_CURVE('',#5253,#5251,#1566,.T.);
#6746=EDGE_CURVE('',#5254,#5255,#891,.T.);
#6747=EDGE_CURVE('',#5254,#5197,#892,.T.);
#6748=EDGE_CURVE('',#5255,#5196,#893,.T.);
#6749=EDGE_CURVE('',#5253,#5256,#894,.T.);
#6750=EDGE_CURVE('',#5256,#5198,#895,.T.);
#6751=EDGE_CURVE('',#5256,#5254,#896,.T.);
#6752=EDGE_CURVE('',#5195,#5257,#897,.T.);
#6753=EDGE_CURVE('',#5257,#5255,#1567,.T.);
#6754=EDGE_CURVE('',#5258,#5259,#898,.T.);
#6755=EDGE_CURVE('',#5258,#5193,#899,.T.);
#6756=EDGE_CURVE('',#5259,#5192,#900,.T.);
#6757=EDGE_CURVE('',#5257,#5260,#901,.T.);
#6758=EDGE_CURVE('',#5260,#5194,#902,.T.);
#6759=EDGE_CURVE('',#5260,#5258,#903,.T.);
#6760=EDGE_CURVE('',#5191,#5261,#904,.T.);
#6761=EDGE_CURVE('',#5261,#5259,#1568,.T.);
#6762=EDGE_CURVE('',#5262,#5263,#905,.T.);
#6763=EDGE_CURVE('',#5262,#5189,#906,.T.);
#6764=EDGE_CURVE('',#5263,#5188,#907,.T.);
#6765=EDGE_CURVE('',#5261,#5264,#908,.T.);
#6766=EDGE_CURVE('',#5264,#5190,#909,.T.);
#6767=EDGE_CURVE('',#5264,#5262,#910,.T.);
#6768=EDGE_CURVE('',#5187,#5265,#911,.T.);
#6769=EDGE_CURVE('',#5265,#5263,#1569,.T.);
#6770=EDGE_CURVE('',#5266,#5267,#912,.T.);
#6771=EDGE_CURVE('',#5266,#5185,#913,.T.);
#6772=EDGE_CURVE('',#5267,#5184,#914,.T.);
#6773=EDGE_CURVE('',#5265,#5268,#915,.T.);
#6774=EDGE_CURVE('',#5268,#5186,#916,.T.);
#6775=EDGE_CURVE('',#5268,#5266,#917,.T.);
#6776=EDGE_CURVE('',#5183,#5269,#918,.T.);
#6777=EDGE_CURVE('',#5269,#5267,#1570,.T.);
#6778=EDGE_CURVE('',#5270,#5271,#919,.T.);
#6779=EDGE_CURVE('',#5270,#5181,#920,.T.);
#6780=EDGE_CURVE('',#5271,#5180,#921,.T.);
#6781=EDGE_CURVE('',#5269,#5272,#922,.T.);
#6782=EDGE_CURVE('',#5272,#5182,#923,.T.);
#6783=EDGE_CURVE('',#5272,#5270,#924,.T.);
#6784=EDGE_CURVE('',#5179,#5273,#925,.T.);
#6785=EDGE_CURVE('',#5273,#5271,#1571,.T.);
#6786=EDGE_CURVE('',#5274,#5275,#926,.T.);
#6787=EDGE_CURVE('',#5274,#5177,#927,.T.);
#6788=EDGE_CURVE('',#5275,#5176,#928,.T.);
#6789=EDGE_CURVE('',#5273,#5276,#929,.T.);
#6790=EDGE_CURVE('',#5276,#5178,#930,.T.);
#6791=EDGE_CURVE('',#5276,#5274,#931,.T.);
#6792=EDGE_CURVE('',#5175,#5277,#932,.T.);
#6793=EDGE_CURVE('',#5277,#5275,#1572,.T.);
#6794=EDGE_CURVE('',#5278,#5174,#933,.T.);
#6795=EDGE_CURVE('',#5277,#5278,#934,.T.);
#6796=EDGE_CURVE('',#5279,#5173,#935,.T.);
#6797=EDGE_CURVE('',#5278,#5279,#936,.T.);
#6798=EDGE_CURVE('',#5280,#5172,#937,.T.);
#6799=EDGE_CURVE('',#5279,#5280,#938,.T.);
#6800=EDGE_CURVE('',#5281,#5170,#939,.T.);
#6801=EDGE_CURVE('',#5282,#5281,#940,.T.);
#6802=EDGE_CURVE('',#5171,#5282,#941,.T.);
#6803=EDGE_CURVE('',#5283,#5169,#942,.T.);
#6804=EDGE_CURVE('',#5281,#5283,#943,.T.);
#6805=EDGE_CURVE('',#5283,#5207,#944,.T.);
#6806=EDGE_CURVE('',#5284,#5284,#1573,.T.);
#6807=EDGE_CURVE('',#5284,#5243,#3534,.T.);
#6808=EDGE_CURVE('',#5282,#5280,#1574,.T.);
#6809=EDGE_CURVE('',#5285,#5285,#1575,.T.);
#6810=EDGE_CURVE('',#5285,#5286,#3535,.T.);
#6811=EDGE_CURVE('',#5286,#5286,#1576,.T.);
#6812=EDGE_CURVE('',#5286,#5287,#3536,.T.);
#6813=EDGE_CURVE('',#5287,#5287,#1577,.T.);
#6814=EDGE_CURVE('',#5287,#5288,#3537,.T.);
#6815=EDGE_CURVE('',#5288,#5288,#1578,.T.);
#9045=ORIENTED_EDGE('',*,*,#6534,.F.);
#9046=ORIENTED_EDGE('',*,*,#6535,.T.);
#9047=ORIENTED_EDGE('',*,*,#6536,.T.);
#9048=ORIENTED_EDGE('',*,*,#6537,.T.);
#9049=ORIENTED_EDGE('',*,*,#6538,.T.);
#9050=ORIENTED_EDGE('',*,*,#6539,.T.);
#9051=ORIENTED_EDGE('',*,*,#6537,.F.);
#9052=ORIENTED_EDGE('',*,*,#6540,.T.);
#9053=ORIENTED_EDGE('',*,*,#6541,.T.);
#9054=ORIENTED_EDGE('',*,*,#6541,.F.);
#9055=ORIENTED_EDGE('',*,*,#6542,.F.);
#9056=ORIENTED_EDGE('',*,*,#6543,.F.);
#9057=ORIENTED_EDGE('',*,*,#6544,.F.);
#9058=ORIENTED_EDGE('',*,*,#6545,.T.);
#9059=ORIENTED_EDGE('',*,*,#6535,.F.);
#9060=ORIENTED_EDGE('',*,*,#6546,.T.);
#9061=ORIENTED_EDGE('',*,*,#6547,.F.);
#9062=ORIENTED_EDGE('',*,*,#6548,.F.);
#9063=ORIENTED_EDGE('',*,*,#6538,.F.);
#9064=ORIENTED_EDGE('',*,*,#6539,.F.);
#9065=ORIENTED_EDGE('',*,*,#6549,.T.);
#9066=ORIENTED_EDGE('',*,*,#6550,.F.);
#9067=ORIENTED_EDGE('',*,*,#6551,.F.);
#9068=ORIENTED_EDGE('',*,*,#6549,.F.);
#9069=ORIENTED_EDGE('',*,*,#6552,.F.);
#9070=ORIENTED_EDGE('',*,*,#6544,.T.);
#9071=ORIENTED_EDGE('',*,*,#6553,.T.);
#9072=ORIENTED_EDGE('',*,*,#6554,.T.);
#9073=ORIENTED_EDGE('',*,*,#6555,.T.);
#9074=ORIENTED_EDGE('',*,*,#6556,.T.);
#9075=ORIENTED_EDGE('',*,*,#6554,.F.);
#9076=ORIENTED_EDGE('',*,*,#6557,.T.);
#9077=ORIENTED_EDGE('',*,*,#6547,.T.);
#9078=ORIENTED_EDGE('',*,*,#6558,.F.);
#9079=ORIENTED_EDGE('',*,*,#6559,.F.);
#9080=ORIENTED_EDGE('',*,*,#6560,.T.);
#9081=ORIENTED_EDGE('',*,*,#6555,.F.);
#9082=ORIENTED_EDGE('',*,*,#6556,.F.);
#9083=ORIENTED_EDGE('',*,*,#6560,.F.);
#9084=ORIENTED_EDGE('',*,*,#6561,.F.);
#9085=ORIENTED_EDGE('',*,*,#6562,.T.);
#9086=ORIENTED_EDGE('',*,*,#6542,.T.);
#9087=ORIENTED_EDGE('',*,*,#6540,.F.);
#9088=ORIENTED_EDGE('',*,*,#6536,.F.);
#9089=ORIENTED_EDGE('',*,*,#6548,.T.);
#9090=ORIENTED_EDGE('',*,*,#6557,.F.);
#9091=ORIENTED_EDGE('',*,*,#6553,.F.);
#9092=ORIENTED_EDGE('',*,*,#6543,.T.);
#9093=ORIENTED_EDGE('',*,*,#6562,.F.);
#9094=ORIENTED_EDGE('',*,*,#6563,.F.);
#9095=ORIENTED_EDGE('',*,*,#6564,.T.);
#9096=ORIENTED_EDGE('',*,*,#6565,.F.);
#9097=ORIENTED_EDGE('',*,*,#6566,.F.);
#9098=ORIENTED_EDGE('',*,*,#6567,.F.);
#9099=ORIENTED_EDGE('',*,*,#6568,.F.);
#9100=ORIENTED_EDGE('',*,*,#6569,.F.);
#9101=ORIENTED_EDGE('',*,*,#6570,.F.);
#9102=ORIENTED_EDGE('',*,*,#6571,.F.);
#9103=ORIENTED_EDGE('',*,*,#6570,.T.);
#9104=ORIENTED_EDGE('',*,*,#6572,.F.);
#9105=ORIENTED_EDGE('',*,*,#6564,.F.);
#9106=ORIENTED_EDGE('',*,*,#6573,.F.);
#9107=ORIENTED_EDGE('',*,*,#6574,.T.);
#9108=ORIENTED_EDGE('',*,*,#6575,.T.);
#9109=ORIENTED_EDGE('',*,*,#6576,.T.);
#9110=ORIENTED_EDGE('',*,*,#6577,.T.);
#9111=ORIENTED_EDGE('',*,*,#6578,.T.);
#9112=ORIENTED_EDGE('',*,*,#6579,.T.);
#9113=ORIENTED_EDGE('',*,*,#6580,.T.);
#9114=ORIENTED_EDGE('',*,*,#6581,.T.);
#9115=ORIENTED_EDGE('',*,*,#6582,.T.);
#9116=ORIENTED_EDGE('',*,*,#6583,.T.);
#9117=ORIENTED_EDGE('',*,*,#6584,.T.);
#9118=ORIENTED_EDGE('',*,*,#6585,.T.);
#9119=ORIENTED_EDGE('',*,*,#6586,.T.);
#9120=ORIENTED_EDGE('',*,*,#6587,.T.);
#9121=ORIENTED_EDGE('',*,*,#6588,.T.);
#9122=ORIENTED_EDGE('',*,*,#6589,.T.);
#9123=ORIENTED_EDGE('',*,*,#6590,.T.);
#9124=ORIENTED_EDGE('',*,*,#6591,.T.);
#9125=ORIENTED_EDGE('',*,*,#6592,.T.);
#9126=ORIENTED_EDGE('',*,*,#6593,.T.);
#9127=ORIENTED_EDGE('',*,*,#6594,.T.);
#9128=ORIENTED_EDGE('',*,*,#6595,.T.);
#9129=ORIENTED_EDGE('',*,*,#6596,.T.);
#9130=ORIENTED_EDGE('',*,*,#6597,.T.);
#9131=ORIENTED_EDGE('',*,*,#6598,.T.);
#9132=ORIENTED_EDGE('',*,*,#6599,.T.);
#9133=ORIENTED_EDGE('',*,*,#6600,.T.);
#9134=ORIENTED_EDGE('',*,*,#6601,.T.);
#9135=ORIENTED_EDGE('',*,*,#6602,.T.);
#9136=ORIENTED_EDGE('',*,*,#6603,.T.);
#9137=ORIENTED_EDGE('',*,*,#6604,.T.);
#9138=ORIENTED_EDGE('',*,*,#6605,.T.);
#9139=ORIENTED_EDGE('',*,*,#6606,.T.);
#9140=ORIENTED_EDGE('',*,*,#6607,.T.);
#9141=ORIENTED_EDGE('',*,*,#6608,.T.);
#9142=ORIENTED_EDGE('',*,*,#6609,.T.);
#9143=ORIENTED_EDGE('',*,*,#6610,.T.);
#9144=ORIENTED_EDGE('',*,*,#6611,.T.);
#9145=ORIENTED_EDGE('',*,*,#6612,.T.);
#9146=ORIENTED_EDGE('',*,*,#6565,.T.);
#9147=ORIENTED_EDGE('',*,*,#6572,.T.);
#9148=ORIENTED_EDGE('',*,*,#6569,.T.);
#9149=ORIENTED_EDGE('',*,*,#6613,.T.);
#9150=ORIENTED_EDGE('',*,*,#6614,.T.);
#9151=ORIENTED_EDGE('',*,*,#6615,.T.);
#9152=ORIENTED_EDGE('',*,*,#6616,.T.);
#9153=ORIENTED_EDGE('',*,*,#6617,.T.);
#9154=ORIENTED_EDGE('',*,*,#6618,.T.);
#9155=ORIENTED_EDGE('',*,*,#6619,.T.);
#9156=ORIENTED_EDGE('',*,*,#6620,.T.);
#9157=ORIENTED_EDGE('',*,*,#6621,.T.);
#9158=ORIENTED_EDGE('',*,*,#6622,.T.);
#9159=ORIENTED_EDGE('',*,*,#6623,.T.);
#9160=ORIENTED_EDGE('',*,*,#6624,.T.);
#9161=ORIENTED_EDGE('',*,*,#6625,.T.);
#9162=ORIENTED_EDGE('',*,*,#6626,.T.);
#9163=ORIENTED_EDGE('',*,*,#6627,.T.);
#9164=ORIENTED_EDGE('',*,*,#6628,.T.);
#9165=ORIENTED_EDGE('',*,*,#6629,.T.);
#9166=ORIENTED_EDGE('',*,*,#6630,.T.);
#9167=ORIENTED_EDGE('',*,*,#6631,.T.);
#9168=ORIENTED_EDGE('',*,*,#6632,.T.);
#9169=ORIENTED_EDGE('',*,*,#6633,.T.);
#9170=ORIENTED_EDGE('',*,*,#6634,.T.);
#9171=ORIENTED_EDGE('',*,*,#6635,.T.);
#9172=ORIENTED_EDGE('',*,*,#6636,.T.);
#9173=ORIENTED_EDGE('',*,*,#6637,.T.);
#9174=ORIENTED_EDGE('',*,*,#6638,.T.);
#9175=ORIENTED_EDGE('',*,*,#6639,.T.);
#9176=ORIENTED_EDGE('',*,*,#6640,.T.);
#9177=ORIENTED_EDGE('',*,*,#6641,.T.);
#9178=ORIENTED_EDGE('',*,*,#6642,.T.);
#9179=ORIENTED_EDGE('',*,*,#6643,.T.);
#9180=ORIENTED_EDGE('',*,*,#6644,.T.);
#9181=ORIENTED_EDGE('',*,*,#6645,.T.);
#9182=ORIENTED_EDGE('',*,*,#6646,.T.);
#9183=ORIENTED_EDGE('',*,*,#6647,.T.);
#9184=ORIENTED_EDGE('',*,*,#6648,.T.);
#9185=ORIENTED_EDGE('',*,*,#6649,.T.);
#9186=ORIENTED_EDGE('',*,*,#6650,.T.);
#9187=ORIENTED_EDGE('',*,*,#6651,.T.);
#9188=ORIENTED_EDGE('',*,*,#6652,.T.);
#9189=ORIENTED_EDGE('',*,*,#6574,.F.);
#9190=ORIENTED_EDGE('',*,*,#6568,.T.);
#9191=ORIENTED_EDGE('',*,*,#6653,.T.);
#9192=ORIENTED_EDGE('',*,*,#6654,.T.);
#9193=ORIENTED_EDGE('',*,*,#6613,.F.);
#9194=ORIENTED_EDGE('',*,*,#6566,.T.);
#9195=ORIENTED_EDGE('',*,*,#6612,.F.);
#9196=ORIENTED_EDGE('',*,*,#6655,.T.);
#9197=ORIENTED_EDGE('',*,*,#6656,.T.);
#9198=ORIENTED_EDGE('',*,*,#6657,.F.);
#9199=ORIENTED_EDGE('',*,*,#6658,.T.);
#9200=ORIENTED_EDGE('',*,*,#6609,.F.);
#9201=ORIENTED_EDGE('',*,*,#6659,.F.);
#9202=ORIENTED_EDGE('',*,*,#6660,.F.);
#9203=ORIENTED_EDGE('',*,*,#6655,.F.);
#9204=ORIENTED_EDGE('',*,*,#6611,.F.);
#9205=ORIENTED_EDGE('',*,*,#6661,.F.);
#9206=ORIENTED_EDGE('',*,*,#6662,.F.);
#9207=ORIENTED_EDGE('',*,*,#6661,.T.);
#9208=ORIENTED_EDGE('',*,*,#6610,.F.);
#9209=ORIENTED_EDGE('',*,*,#6658,.F.);
#9210=ORIENTED_EDGE('',*,*,#6659,.T.);
#9211=ORIENTED_EDGE('',*,*,#6608,.F.);
#9212=ORIENTED_EDGE('',*,*,#6663,.T.);
#9213=ORIENTED_EDGE('',*,*,#6664,.T.);
#9214=ORIENTED_EDGE('',*,*,#6665,.F.);
#9215=ORIENTED_EDGE('',*,*,#6666,.T.);
#9216=ORIENTED_EDGE('',*,*,#6605,.F.);
#9217=ORIENTED_EDGE('',*,*,#6667,.F.);
#9218=ORIENTED_EDGE('',*,*,#6668,.F.);
#9219=ORIENTED_EDGE('',*,*,#6663,.F.);
#9220=ORIENTED_EDGE('',*,*,#6607,.F.);
#9221=ORIENTED_EDGE('',*,*,#6669,.F.);
#9222=ORIENTED_EDGE('',*,*,#6670,.F.);
#9223=ORIENTED_EDGE('',*,*,#6669,.T.);
#9224=ORIENTED_EDGE('',*,*,#6606,.F.);
#9225=ORIENTED_EDGE('',*,*,#6666,.F.);
#9226=ORIENTED_EDGE('',*,*,#6667,.T.);
#9227=ORIENTED_EDGE('',*,*,#6604,.F.);
#9228=ORIENTED_EDGE('',*,*,#6671,.T.);
#9229=ORIENTED_EDGE('',*,*,#6672,.T.);
#9230=ORIENTED_EDGE('',*,*,#6673,.F.);
#9231=ORIENTED_EDGE('',*,*,#6674,.T.);
#9232=ORIENTED_EDGE('',*,*,#6601,.F.);
#9233=ORIENTED_EDGE('',*,*,#6675,.F.);
#9234=ORIENTED_EDGE('',*,*,#6676,.F.);
#9235=ORIENTED_EDGE('',*,*,#6671,.F.);
#9236=ORIENTED_EDGE('',*,*,#6603,.F.);
#9237=ORIENTED_EDGE('',*,*,#6677,.F.);
#9238=ORIENTED_EDGE('',*,*,#6678,.F.);
#9239=ORIENTED_EDGE('',*,*,#6677,.T.);
#9240=ORIENTED_EDGE('',*,*,#6602,.F.);
#9241=ORIENTED_EDGE('',*,*,#6674,.F.);
#9242=ORIENTED_EDGE('',*,*,#6675,.T.);
#9243=ORIENTED_EDGE('',*,*,#6600,.F.);
#9244=ORIENTED_EDGE('',*,*,#6679,.T.);
#9245=ORIENTED_EDGE('',*,*,#6680,.T.);
#9246=ORIENTED_EDGE('',*,*,#6681,.F.);
#9247=ORIENTED_EDGE('',*,*,#6682,.T.);
#9248=ORIENTED_EDGE('',*,*,#6597,.F.);
#9249=ORIENTED_EDGE('',*,*,#6683,.F.);
#9250=ORIENTED_EDGE('',*,*,#6684,.F.);
#9251=ORIENTED_EDGE('',*,*,#6679,.F.);
#9252=ORIENTED_EDGE('',*,*,#6599,.F.);
#9253=ORIENTED_EDGE('',*,*,#6685,.F.);
#9254=ORIENTED_EDGE('',*,*,#6686,.F.);
#9255=ORIENTED_EDGE('',*,*,#6685,.T.);
#9256=ORIENTED_EDGE('',*,*,#6598,.F.);
#9257=ORIENTED_EDGE('',*,*,#6682,.F.);
#9258=ORIENTED_EDGE('',*,*,#6683,.T.);
#9259=ORIENTED_EDGE('',*,*,#6596,.F.);
#9260=ORIENTED_EDGE('',*,*,#6687,.T.);
#9261=ORIENTED_EDGE('',*,*,#6688,.T.);
#9262=ORIENTED_EDGE('',*,*,#6689,.F.);
#9263=ORIENTED_EDGE('',*,*,#6690,.T.);
#9264=ORIENTED_EDGE('',*,*,#6593,.F.);
#9265=ORIENTED_EDGE('',*,*,#6691,.F.);
#9266=ORIENTED_EDGE('',*,*,#6692,.F.);
#9267=ORIENTED_EDGE('',*,*,#6687,.F.);
#9268=ORIENTED_EDGE('',*,*,#6595,.F.);
#9269=ORIENTED_EDGE('',*,*,#6693,.F.);
#9270=ORIENTED_EDGE('',*,*,#6694,.F.);
#9271=ORIENTED_EDGE('',*,*,#6693,.T.);
#9272=ORIENTED_EDGE('',*,*,#6594,.F.);
#9273=ORIENTED_EDGE('',*,*,#6690,.F.);
#9274=ORIENTED_EDGE('',*,*,#6691,.T.);
#9275=ORIENTED_EDGE('',*,*,#6592,.F.);
#9276=ORIENTED_EDGE('',*,*,#6695,.T.);
#9277=ORIENTED_EDGE('',*,*,#6696,.T.);
#9278=ORIENTED_EDGE('',*,*,#6697,.F.);
#9279=ORIENTED_EDGE('',*,*,#6698,.T.);
#9280=ORIENTED_EDGE('',*,*,#6589,.F.);
#9281=ORIENTED_EDGE('',*,*,#6699,.F.);
#9282=ORIENTED_EDGE('',*,*,#6700,.F.);
#9283=ORIENTED_EDGE('',*,*,#6695,.F.);
#9284=ORIENTED_EDGE('',*,*,#6591,.F.);
#9285=ORIENTED_EDGE('',*,*,#6701,.F.);
#9286=ORIENTED_EDGE('',*,*,#6702,.F.);
#9287=ORIENTED_EDGE('',*,*,#6701,.T.);
#9288=ORIENTED_EDGE('',*,*,#6590,.F.);
#9289=ORIENTED_EDGE('',*,*,#6698,.F.);
#9290=ORIENTED_EDGE('',*,*,#6699,.T.);
#9291=ORIENTED_EDGE('',*,*,#6588,.F.);
#9292=ORIENTED_EDGE('',*,*,#6703,.T.);
#9293=ORIENTED_EDGE('',*,*,#6704,.T.);
#9294=ORIENTED_EDGE('',*,*,#6705,.F.);
#9295=ORIENTED_EDGE('',*,*,#6706,.T.);
#9296=ORIENTED_EDGE('',*,*,#6585,.F.);
#9297=ORIENTED_EDGE('',*,*,#6707,.F.);
#9298=ORIENTED_EDGE('',*,*,#6708,.F.);
#9299=ORIENTED_EDGE('',*,*,#6703,.F.);
#9300=ORIENTED_EDGE('',*,*,#6587,.F.);
#9301=ORIENTED_EDGE('',*,*,#6709,.F.);
#9302=ORIENTED_EDGE('',*,*,#6710,.F.);
#9303=ORIENTED_EDGE('',*,*,#6709,.T.);
#9304=ORIENTED_EDGE('',*,*,#6586,.F.);
#9305=ORIENTED_EDGE('',*,*,#6706,.F.);
#9306=ORIENTED_EDGE('',*,*,#6707,.T.);
#9307=ORIENTED_EDGE('',*,*,#6584,.F.);
#9308=ORIENTED_EDGE('',*,*,#6711,.T.);
#9309=ORIENTED_EDGE('',*,*,#6712,.T.);
#9310=ORIENTED_EDGE('',*,*,#6713,.F.);
#9311=ORIENTED_EDGE('',*,*,#6714,.T.);
#9312=ORIENTED_EDGE('',*,*,#6581,.F.);
#9313=ORIENTED_EDGE('',*,*,#6715,.F.);
#9314=ORIENTED_EDGE('',*,*,#6716,.F.);
#9315=ORIENTED_EDGE('',*,*,#6711,.F.);
#9316=ORIENTED_EDGE('',*,*,#6583,.F.);
#9317=ORIENTED_EDGE('',*,*,#6717,.F.);
#9318=ORIENTED_EDGE('',*,*,#6718,.F.);
#9319=ORIENTED_EDGE('',*,*,#6717,.T.);
#9320=ORIENTED_EDGE('',*,*,#6582,.F.);
#9321=ORIENTED_EDGE('',*,*,#6714,.F.);
#9322=ORIENTED_EDGE('',*,*,#6715,.T.);
#9323=ORIENTED_EDGE('',*,*,#6580,.F.);
#9324=ORIENTED_EDGE('',*,*,#6719,.T.);
#9325=ORIENTED_EDGE('',*,*,#6720,.T.);
#9326=ORIENTED_EDGE('',*,*,#6721,.F.);
#9327=ORIENTED_EDGE('',*,*,#6722,.T.);
#9328=ORIENTED_EDGE('',*,*,#6577,.F.);
#9329=ORIENTED_EDGE('',*,*,#6723,.F.);
#9330=ORIENTED_EDGE('',*,*,#6724,.F.);
#9331=ORIENTED_EDGE('',*,*,#6719,.F.);
#9332=ORIENTED_EDGE('',*,*,#6579,.F.);
#9333=ORIENTED_EDGE('',*,*,#6725,.F.);
#9334=ORIENTED_EDGE('',*,*,#6726,.F.);
#9335=ORIENTED_EDGE('',*,*,#6727,.F.);
#9336=ORIENTED_EDGE('',*,*,#6725,.T.);
#9337=ORIENTED_EDGE('',*,*,#6578,.F.);
#9338=ORIENTED_EDGE('',*,*,#6722,.F.);
#9339=ORIENTED_EDGE('',*,*,#6723,.T.);
#9340=ORIENTED_EDGE('',*,*,#6576,.F.);
#9341=ORIENTED_EDGE('',*,*,#6728,.T.);
#9342=ORIENTED_EDGE('',*,*,#6729,.T.);
#9343=ORIENTED_EDGE('',*,*,#6730,.F.);
#9344=ORIENTED_EDGE('',*,*,#6731,.T.);
#9345=ORIENTED_EDGE('',*,*,#6650,.F.);
#9346=ORIENTED_EDGE('',*,*,#6732,.F.);
#9347=ORIENTED_EDGE('',*,*,#6733,.F.);
#9348=ORIENTED_EDGE('',*,*,#6728,.F.);
#9349=ORIENTED_EDGE('',*,*,#6575,.F.);
#9350=ORIENTED_EDGE('',*,*,#6652,.F.);
#9351=ORIENTED_EDGE('',*,*,#6734,.F.);
#9352=ORIENTED_EDGE('',*,*,#6735,.F.);
#9353=ORIENTED_EDGE('',*,*,#6734,.T.);
#9354=ORIENTED_EDGE('',*,*,#6651,.F.);
#9355=ORIENTED_EDGE('',*,*,#6731,.F.);
#9356=ORIENTED_EDGE('',*,*,#6732,.T.);
#9357=ORIENTED_EDGE('',*,*,#6649,.F.);
#9358=ORIENTED_EDGE('',*,*,#6736,.T.);
#9359=ORIENTED_EDGE('',*,*,#6737,.T.);
#9360=ORIENTED_EDGE('',*,*,#6738,.F.);
#9361=ORIENTED_EDGE('',*,*,#6739,.T.);
#9362=ORIENTED_EDGE('',*,*,#6646,.F.);
#9363=ORIENTED_EDGE('',*,*,#6740,.F.);
#9364=ORIENTED_EDGE('',*,*,#6741,.F.);
#9365=ORIENTED_EDGE('',*,*,#6736,.F.);
#9366=ORIENTED_EDGE('',*,*,#6648,.F.);
#9367=ORIENTED_EDGE('',*,*,#6742,.F.);
#9368=ORIENTED_EDGE('',*,*,#6743,.F.);
#9369=ORIENTED_EDGE('',*,*,#6742,.T.);
#9370=ORIENTED_EDGE('',*,*,#6647,.F.);
#9371=ORIENTED_EDGE('',*,*,#6739,.F.);
#9372=ORIENTED_EDGE('',*,*,#6740,.T.);
#9373=ORIENTED_EDGE('',*,*,#6645,.F.);
#9374=ORIENTED_EDGE('',*,*,#6744,.T.);
#9375=ORIENTED_EDGE('',*,*,#6745,.T.);
#9376=ORIENTED_EDGE('',*,*,#6746,.F.);
#9377=ORIENTED_EDGE('',*,*,#6747,.T.);
#9378=ORIENTED_EDGE('',*,*,#6642,.F.);
#9379=ORIENTED_EDGE('',*,*,#6748,.F.);
#9380=ORIENTED_EDGE('',*,*,#6749,.F.);
#9381=ORIENTED_EDGE('',*,*,#6744,.F.);
#9382=ORIENTED_EDGE('',*,*,#6644,.F.);
#9383=ORIENTED_EDGE('',*,*,#6750,.F.);
#9384=ORIENTED_EDGE('',*,*,#6751,.F.);
#9385=ORIENTED_EDGE('',*,*,#6750,.T.);
#9386=ORIENTED_EDGE('',*,*,#6643,.F.);
#9387=ORIENTED_EDGE('',*,*,#6747,.F.);
#9388=ORIENTED_EDGE('',*,*,#6748,.T.);
#9389=ORIENTED_EDGE('',*,*,#6641,.F.);
#9390=ORIENTED_EDGE('',*,*,#6752,.T.);
#9391=ORIENTED_EDGE('',*,*,#6753,.T.);
#9392=ORIENTED_EDGE('',*,*,#6754,.F.);
#9393=ORIENTED_EDGE('',*,*,#6755,.T.);
#9394=ORIENTED_EDGE('',*,*,#6638,.F.);
#9395=ORIENTED_EDGE('',*,*,#6756,.F.);
#9396=ORIENTED_EDGE('',*,*,#6757,.F.);
#9397=ORIENTED_EDGE('',*,*,#6752,.F.);
#9398=ORIENTED_EDGE('',*,*,#6640,.F.);
#9399=ORIENTED_EDGE('',*,*,#6758,.F.);
#9400=ORIENTED_EDGE('',*,*,#6759,.F.);
#9401=ORIENTED_EDGE('',*,*,#6758,.T.);
#9402=ORIENTED_EDGE('',*,*,#6639,.F.);
#9403=ORIENTED_EDGE('',*,*,#6755,.F.);
#9404=ORIENTED_EDGE('',*,*,#6756,.T.);
#9405=ORIENTED_EDGE('',*,*,#6637,.F.);
#9406=ORIENTED_EDGE('',*,*,#6760,.T.);
#9407=ORIENTED_EDGE('',*,*,#6761,.T.);
#9408=ORIENTED_EDGE('',*,*,#6762,.F.);
#9409=ORIENTED_EDGE('',*,*,#6763,.T.);
#9410=ORIENTED_EDGE('',*,*,#6634,.F.);
#9411=ORIENTED_EDGE('',*,*,#6764,.F.);
#9412=ORIENTED_EDGE('',*,*,#6765,.F.);
#9413=ORIENTED_EDGE('',*,*,#6760,.F.);
#9414=ORIENTED_EDGE('',*,*,#6636,.F.);
#9415=ORIENTED_EDGE('',*,*,#6766,.F.);
#9416=ORIENTED_EDGE('',*,*,#6767,.F.);
#9417=ORIENTED_EDGE('',*,*,#6766,.T.);
#9418=ORIENTED_EDGE('',*,*,#6635,.F.);
#9419=ORIENTED_EDGE('',*,*,#6763,.F.);
#9420=ORIENTED_EDGE('',*,*,#6764,.T.);
#9421=ORIENTED_EDGE('',*,*,#6633,.F.);
#9422=ORIENTED_EDGE('',*,*,#6768,.T.);
#9423=ORIENTED_EDGE('',*,*,#6769,.T.);
#9424=ORIENTED_EDGE('',*,*,#6770,.F.);
#9425=ORIENTED_EDGE('',*,*,#6771,.T.);
#9426=ORIENTED_EDGE('',*,*,#6630,.F.);
#9427=ORIENTED_EDGE('',*,*,#6772,.F.);
#9428=ORIENTED_EDGE('',*,*,#6773,.F.);
#9429=ORIENTED_EDGE('',*,*,#6768,.F.);
#9430=ORIENTED_EDGE('',*,*,#6632,.F.);
#9431=ORIENTED_EDGE('',*,*,#6774,.F.);
#9432=ORIENTED_EDGE('',*,*,#6775,.F.);
#9433=ORIENTED_EDGE('',*,*,#6774,.T.);
#9434=ORIENTED_EDGE('',*,*,#6631,.F.);
#9435=ORIENTED_EDGE('',*,*,#6771,.F.);
#9436=ORIENTED_EDGE('',*,*,#6772,.T.);
#9437=ORIENTED_EDGE('',*,*,#6629,.F.);
#9438=ORIENTED_EDGE('',*,*,#6776,.T.);
#9439=ORIENTED_EDGE('',*,*,#6777,.T.);
#9440=ORIENTED_EDGE('',*,*,#6778,.F.);
#9441=ORIENTED_EDGE('',*,*,#6779,.T.);
#9442=ORIENTED_EDGE('',*,*,#6626,.F.);
#9443=ORIENTED_EDGE('',*,*,#6780,.F.);
#9444=ORIENTED_EDGE('',*,*,#6781,.F.);
#9445=ORIENTED_EDGE('',*,*,#6776,.F.);
#9446=ORIENTED_EDGE('',*,*,#6628,.F.);
#9447=ORIENTED_EDGE('',*,*,#6782,.F.);
#9448=ORIENTED_EDGE('',*,*,#6783,.F.);
#9449=ORIENTED_EDGE('',*,*,#6782,.T.);
#9450=ORIENTED_EDGE('',*,*,#6627,.F.);
#9451=ORIENTED_EDGE('',*,*,#6779,.F.);
#9452=ORIENTED_EDGE('',*,*,#6780,.T.);
#9453=ORIENTED_EDGE('',*,*,#6625,.F.);
#9454=ORIENTED_EDGE('',*,*,#6784,.T.);
#9455=ORIENTED_EDGE('',*,*,#6785,.T.);
#9456=ORIENTED_EDGE('',*,*,#6786,.F.);
#9457=ORIENTED_EDGE('',*,*,#6787,.T.);
#9458=ORIENTED_EDGE('',*,*,#6622,.F.);
#9459=ORIENTED_EDGE('',*,*,#6788,.F.);
#9460=ORIENTED_EDGE('',*,*,#6789,.F.);
#9461=ORIENTED_EDGE('',*,*,#6784,.F.);
#9462=ORIENTED_EDGE('',*,*,#6624,.F.);
#9463=ORIENTED_EDGE('',*,*,#6790,.F.);
#9464=ORIENTED_EDGE('',*,*,#6791,.F.);
#9465=ORIENTED_EDGE('',*,*,#6790,.T.);
#9466=ORIENTED_EDGE('',*,*,#6623,.F.);
#9467=ORIENTED_EDGE('',*,*,#6787,.F.);
#9468=ORIENTED_EDGE('',*,*,#6788,.T.);
#9469=ORIENTED_EDGE('',*,*,#6621,.F.);
#9470=ORIENTED_EDGE('',*,*,#6792,.T.);
#9471=ORIENTED_EDGE('',*,*,#6793,.T.);
#9472=ORIENTED_EDGE('',*,*,#6620,.F.);
#9473=ORIENTED_EDGE('',*,*,#6794,.F.);
#9474=ORIENTED_EDGE('',*,*,#6795,.F.);
#9475=ORIENTED_EDGE('',*,*,#6792,.F.);
#9476=ORIENTED_EDGE('',*,*,#6619,.F.);
#9477=ORIENTED_EDGE('',*,*,#6796,.F.);
#9478=ORIENTED_EDGE('',*,*,#6797,.F.);
#9479=ORIENTED_EDGE('',*,*,#6794,.T.);
#9480=ORIENTED_EDGE('',*,*,#6618,.F.);
#9481=ORIENTED_EDGE('',*,*,#6798,.F.);
#9482=ORIENTED_EDGE('',*,*,#6799,.F.);
#9483=ORIENTED_EDGE('',*,*,#6796,.T.);
#9484=ORIENTED_EDGE('',*,*,#6616,.F.);
#9485=ORIENTED_EDGE('',*,*,#6800,.F.);
#9486=ORIENTED_EDGE('',*,*,#6801,.F.);
#9487=ORIENTED_EDGE('',*,*,#6802,.F.);
#9488=ORIENTED_EDGE('',*,*,#6615,.F.);
#9489=ORIENTED_EDGE('',*,*,#6803,.F.);
#9490=ORIENTED_EDGE('',*,*,#6804,.F.);
#9491=ORIENTED_EDGE('',*,*,#6800,.T.);
#9492=ORIENTED_EDGE('',*,*,#6614,.F.);
#9493=ORIENTED_EDGE('',*,*,#6654,.F.);
#9494=ORIENTED_EDGE('',*,*,#6805,.F.);
#9495=ORIENTED_EDGE('',*,*,#6803,.T.);
#9496=ORIENTED_EDGE('',*,*,#6806,.T.);
#9497=ORIENTED_EDGE('',*,*,#6807,.T.);
#9498=ORIENTED_EDGE('',*,*,#6726,.T.);
#9499=ORIENTED_EDGE('',*,*,#6727,.T.);
#9500=ORIENTED_EDGE('',*,*,#6721,.T.);
#9501=ORIENTED_EDGE('',*,*,#6729,.F.);
#9502=ORIENTED_EDGE('',*,*,#6733,.T.);
#9503=ORIENTED_EDGE('',*,*,#6735,.T.);
#9504=ORIENTED_EDGE('',*,*,#6730,.T.);
#9505=ORIENTED_EDGE('',*,*,#6737,.F.);
#9506=ORIENTED_EDGE('',*,*,#6741,.T.);
#9507=ORIENTED_EDGE('',*,*,#6743,.T.);
#9508=ORIENTED_EDGE('',*,*,#6738,.T.);
#9509=ORIENTED_EDGE('',*,*,#6745,.F.);
#9510=ORIENTED_EDGE('',*,*,#6749,.T.);
#9511=ORIENTED_EDGE('',*,*,#6751,.T.);
#9512=ORIENTED_EDGE('',*,*,#6746,.T.);
#9513=ORIENTED_EDGE('',*,*,#6753,.F.);
#9514=ORIENTED_EDGE('',*,*,#6757,.T.);
#9515=ORIENTED_EDGE('',*,*,#6759,.T.);
#9516=ORIENTED_EDGE('',*,*,#6754,.T.);
#9517=ORIENTED_EDGE('',*,*,#6761,.F.);
#9518=ORIENTED_EDGE('',*,*,#6765,.T.);
#9519=ORIENTED_EDGE('',*,*,#6767,.T.);
#9520=ORIENTED_EDGE('',*,*,#6762,.T.);
#9521=ORIENTED_EDGE('',*,*,#6769,.F.);
#9522=ORIENTED_EDGE('',*,*,#6773,.T.);
#9523=ORIENTED_EDGE('',*,*,#6775,.T.);
#9524=ORIENTED_EDGE('',*,*,#6770,.T.);
#9525=ORIENTED_EDGE('',*,*,#6777,.F.);
#9526=ORIENTED_EDGE('',*,*,#6781,.T.);
#9527=ORIENTED_EDGE('',*,*,#6783,.T.);
#9528=ORIENTED_EDGE('',*,*,#6778,.T.);
#9529=ORIENTED_EDGE('',*,*,#6785,.F.);
#9530=ORIENTED_EDGE('',*,*,#6789,.T.);
#9531=ORIENTED_EDGE('',*,*,#6791,.T.);
#9532=ORIENTED_EDGE('',*,*,#6786,.T.);
#9533=ORIENTED_EDGE('',*,*,#6793,.F.);
#9534=ORIENTED_EDGE('',*,*,#6795,.T.);
#9535=ORIENTED_EDGE('',*,*,#6797,.T.);
#9536=ORIENTED_EDGE('',*,*,#6799,.T.);
#9537=ORIENTED_EDGE('',*,*,#6808,.F.);
#9538=ORIENTED_EDGE('',*,*,#6801,.T.);
#9539=ORIENTED_EDGE('',*,*,#6804,.T.);
#9540=ORIENTED_EDGE('',*,*,#6805,.T.);
#9541=ORIENTED_EDGE('',*,*,#6653,.F.);
#9542=ORIENTED_EDGE('',*,*,#6567,.T.);
#9543=ORIENTED_EDGE('',*,*,#6571,.T.);
#9544=ORIENTED_EDGE('',*,*,#6563,.T.);
#9545=ORIENTED_EDGE('',*,*,#6656,.F.);
#9546=ORIENTED_EDGE('',*,*,#6660,.T.);
#9547=ORIENTED_EDGE('',*,*,#6662,.T.);
#9548=ORIENTED_EDGE('',*,*,#6657,.T.);
#9549=ORIENTED_EDGE('',*,*,#6664,.F.);
#9550=ORIENTED_EDGE('',*,*,#6668,.T.);
#9551=ORIENTED_EDGE('',*,*,#6670,.T.);
#9552=ORIENTED_EDGE('',*,*,#6665,.T.);
#9553=ORIENTED_EDGE('',*,*,#6672,.F.);
#9554=ORIENTED_EDGE('',*,*,#6676,.T.);
#9555=ORIENTED_EDGE('',*,*,#6678,.T.);
#9556=ORIENTED_EDGE('',*,*,#6673,.T.);
#9557=ORIENTED_EDGE('',*,*,#6680,.F.);
#9558=ORIENTED_EDGE('',*,*,#6684,.T.);
#9559=ORIENTED_EDGE('',*,*,#6686,.T.);
#9560=ORIENTED_EDGE('',*,*,#6681,.T.);
#9561=ORIENTED_EDGE('',*,*,#6688,.F.);
#9562=ORIENTED_EDGE('',*,*,#6692,.T.);
#9563=ORIENTED_EDGE('',*,*,#6694,.T.);
#9564=ORIENTED_EDGE('',*,*,#6689,.T.);
#9565=ORIENTED_EDGE('',*,*,#6696,.F.);
#9566=ORIENTED_EDGE('',*,*,#6700,.T.);
#9567=ORIENTED_EDGE('',*,*,#6702,.T.);
#9568=ORIENTED_EDGE('',*,*,#6697,.T.);
#9569=ORIENTED_EDGE('',*,*,#6704,.F.);
#9570=ORIENTED_EDGE('',*,*,#6708,.T.);
#9571=ORIENTED_EDGE('',*,*,#6710,.T.);
#9572=ORIENTED_EDGE('',*,*,#6705,.T.);
#9573=ORIENTED_EDGE('',*,*,#6712,.F.);
#9574=ORIENTED_EDGE('',*,*,#6716,.T.);
#9575=ORIENTED_EDGE('',*,*,#6718,.T.);
#9576=ORIENTED_EDGE('',*,*,#6713,.T.);
#9577=ORIENTED_EDGE('',*,*,#6720,.F.);
#9578=ORIENTED_EDGE('',*,*,#6724,.T.);
#9579=ORIENTED_EDGE('',*,*,#6807,.F.);
#9580=ORIENTED_EDGE('',*,*,#6798,.T.);
#9581=ORIENTED_EDGE('',*,*,#6617,.F.);
#9582=ORIENTED_EDGE('',*,*,#6802,.T.);
#9583=ORIENTED_EDGE('',*,*,#6808,.T.);
#9584=ORIENTED_EDGE('',*,*,#6573,.T.);
#9585=ORIENTED_EDGE('',*,*,#6545,.F.);
#9586=ORIENTED_EDGE('',*,*,#6552,.T.);
#9587=ORIENTED_EDGE('',*,*,#6546,.F.);
#9588=ORIENTED_EDGE('',*,*,#6534,.T.);
#9589=ORIENTED_EDGE('',*,*,#6561,.T.);
#9590=ORIENTED_EDGE('',*,*,#6809,.F.);
#9591=ORIENTED_EDGE('',*,*,#6809,.T.);
#9592=ORIENTED_EDGE('',*,*,#6810,.T.);
#9593=ORIENTED_EDGE('',*,*,#6811,.F.);
#9594=ORIENTED_EDGE('',*,*,#6810,.F.);
#9595=ORIENTED_EDGE('',*,*,#6811,.T.);
#9596=ORIENTED_EDGE('',*,*,#6812,.T.);
#9597=ORIENTED_EDGE('',*,*,#6813,.F.);
#9598=ORIENTED_EDGE('',*,*,#6812,.F.);
#9599=ORIENTED_EDGE('',*,*,#6558,.T.);
#9600=ORIENTED_EDGE('',*,*,#6559,.T.);
#9601=ORIENTED_EDGE('',*,*,#6550,.T.);
#9602=ORIENTED_EDGE('',*,*,#6551,.T.);
#9603=ORIENTED_EDGE('',*,*,#6813,.T.);
#9604=ORIENTED_EDGE('',*,*,#6814,.T.);
#9605=ORIENTED_EDGE('',*,*,#6815,.F.);
#9606=ORIENTED_EDGE('',*,*,#6814,.F.);
#9607=ORIENTED_EDGE('',*,*,#6806,.F.);
#9608=ORIENTED_EDGE('',*,*,#6815,.T.);
#11570=PLANE('',#12976);
#11571=PLANE('',#12977);
#11572=PLANE('',#12985);
#12029=ADVANCED_FACE('',(#2062),#1268,.T.);
#12030=ADVANCED_FACE('',(#2063),#272,.T.);
#12031=ADVANCED_FACE('',(#2064),#273,.T.);
#12032=ADVANCED_FACE('',(#2065),#274,.F.);
#12033=ADVANCED_FACE('',(#2066),#1269,.T.);
#12034=ADVANCED_FACE('',(#2067),#275,.F.);
#12035=ADVANCED_FACE('',(#2068),#406,.T.);
#12036=ADVANCED_FACE('',(#2069),#1270,.F.);
#12037=ADVANCED_FACE('',(#2070),#1271,.F.);
#12038=ADVANCED_FACE('',(#2071),#1272,.F.);
#12039=ADVANCED_FACE('',(#2072),#407,.T.);
#12040=ADVANCED_FACE('',(#2073),#408,.T.);
#12041=ADVANCED_FACE('',(#2074),#409,.T.);
#12042=ADVANCED_FACE('',(#2075),#1273,.F.);
#12043=ADVANCED_FACE('',(#2076),#1274,.F.);
#12044=ADVANCED_FACE('',(#2077),#1275,.F.);
#12045=ADVANCED_FACE('',(#2078),#410,.T.);
#12046=ADVANCED_FACE('',(#2079),#1276,.F.);
#12047=ADVANCED_FACE('',(#2080),#1277,.F.);
#12048=ADVANCED_FACE('',(#2081),#1278,.F.);
#12049=ADVANCED_FACE('',(#2082),#411,.T.);
#12050=ADVANCED_FACE('',(#2083),#1279,.F.);
#12051=ADVANCED_FACE('',(#2084),#1280,.F.);
#12052=ADVANCED_FACE('',(#2085),#1281,.F.);
#12053=ADVANCED_FACE('',(#2086),#412,.T.);
#12054=ADVANCED_FACE('',(#2087),#1282,.F.);
#12055=ADVANCED_FACE('',(#2088),#1283,.F.);
#12056=ADVANCED_FACE('',(#2089),#1284,.F.);
#12057=ADVANCED_FACE('',(#2090),#413,.T.);
#12058=ADVANCED_FACE('',(#2091),#1285,.F.);
#12059=ADVANCED_FACE('',(#2092),#1286,.F.);
#12060=ADVANCED_FACE('',(#2093),#1287,.F.);
#12061=ADVANCED_FACE('',(#2094),#414,.T.);
#12062=ADVANCED_FACE('',(#2095),#1288,.F.);
#12063=ADVANCED_FACE('',(#2096),#1289,.F.);
#12064=ADVANCED_FACE('',(#2097),#1290,.F.);
#12065=ADVANCED_FACE('',(#2098),#415,.T.);
#12066=ADVANCED_FACE('',(#2099),#1291,.F.);
#12067=ADVANCED_FACE('',(#2100),#1292,.F.);
#12068=ADVANCED_FACE('',(#2101),#1293,.F.);
#12069=ADVANCED_FACE('',(#2102),#416,.T.);
#12070=ADVANCED_FACE('',(#2103),#1294,.F.);
#12071=ADVANCED_FACE('',(#2104),#1295,.F.);
#12072=ADVANCED_FACE('',(#2105),#1296,.F.);
#12073=ADVANCED_FACE('',(#2106),#417,.T.);
#12074=ADVANCED_FACE('',(#2107),#1297,.F.);
#12075=ADVANCED_FACE('',(#2108),#1298,.F.);
#12076=ADVANCED_FACE('',(#2109),#1299,.F.);
#12077=ADVANCED_FACE('',(#2110),#418,.T.);
#12078=ADVANCED_FACE('',(#2111),#1300,.F.);
#12079=ADVANCED_FACE('',(#2112),#1301,.F.);
#12080=ADVANCED_FACE('',(#2113),#1302,.F.);
#12081=ADVANCED_FACE('',(#2114),#419,.T.);
#12082=ADVANCED_FACE('',(#2115),#1303,.F.);
#12083=ADVANCED_FACE('',(#2116),#1304,.F.);
#12084=ADVANCED_FACE('',(#2117),#1305,.F.);
#12085=ADVANCED_FACE('',(#2118),#420,.T.);
#12086=ADVANCED_FACE('',(#2119),#1306,.F.);
#12087=ADVANCED_FACE('',(#2120),#1307,.F.);
#12088=ADVANCED_FACE('',(#2121),#1308,.F.);
#12089=ADVANCED_FACE('',(#2122),#421,.T.);
#12090=ADVANCED_FACE('',(#2123),#1309,.F.);
#12091=ADVANCED_FACE('',(#2124),#1310,.F.);
#12092=ADVANCED_FACE('',(#2125),#1311,.F.);
#12093=ADVANCED_FACE('',(#2126),#422,.T.);
#12094=ADVANCED_FACE('',(#2127),#1312,.F.);
#12095=ADVANCED_FACE('',(#2128),#1313,.F.);
#12096=ADVANCED_FACE('',(#2129),#1314,.F.);
#12097=ADVANCED_FACE('',(#2130),#423,.T.);
#12098=ADVANCED_FACE('',(#2131),#1315,.F.);
#12099=ADVANCED_FACE('',(#2132),#1316,.F.);
#12100=ADVANCED_FACE('',(#2133),#1317,.F.);
#12101=ADVANCED_FACE('',(#2134),#424,.T.);
#12102=ADVANCED_FACE('',(#2135),#1318,.F.);
#12103=ADVANCED_FACE('',(#2136),#1319,.F.);
#12104=ADVANCED_FACE('',(#2137),#1320,.F.);
#12105=ADVANCED_FACE('',(#2138),#425,.T.);
#12106=ADVANCED_FACE('',(#2139),#1321,.F.);
#12107=ADVANCED_FACE('',(#2140),#1322,.F.);
#12108=ADVANCED_FACE('',(#2141),#1323,.F.);
#12109=ADVANCED_FACE('',(#2142),#426,.T.);
#12110=ADVANCED_FACE('',(#2143),#1324,.F.);
#12111=ADVANCED_FACE('',(#2144),#1325,.F.);
#12112=ADVANCED_FACE('',(#2145),#1326,.F.);
#12113=ADVANCED_FACE('',(#2146),#1327,.F.);
#12114=ADVANCED_FACE('',(#2147),#1328,.F.);
#12115=ADVANCED_FACE('',(#2148),#1329,.F.);
#12116=ADVANCED_FACE('',(#2149),#427,.F.);
#12117=ADVANCED_FACE('',(#2150),#428,.T.);
#12118=ADVANCED_FACE('',(#2151,#1370),#11570,.T.);
#12119=ADVANCED_FACE('',(#2152,#1371),#11571,.T.);
#12120=ADVANCED_FACE('',(#2153),#429,.F.);
#12121=ADVANCED_FACE('',(#2154,#1372,#1373),#276,.F.);
#12122=ADVANCED_FACE('',(#2155),#430,.F.);
#12123=ADVANCED_FACE('',(#2156,#1374),#11572,.T.);
#12483=CLOSED_SHELL('',(#12029,#12030,#12031,#12032,#12033,#12034,#12035,
#12036,#12037,#12038,#12039,#12040,#12041,#12042,#12043,#12044,#12045,#12046,
#12047,#12048,#12049,#12050,#12051,#12052,#12053,#12054,#12055,#12056,#12057,
#12058,#12059,#12060,#12061,#12062,#12063,#12064,#12065,#12066,#12067,#12068,
#12069,#12070,#12071,#12072,#12073,#12074,#12075,#12076,#12077,#12078,#12079,
#12080,#12081,#12082,#12083,#12084,#12085,#12086,#12087,#12088,#12089,#12090,
#12091,#12092,#12093,#12094,#12095,#12096,#12097,#12098,#12099,#12100,#12101,
#12102,#12103,#12104,#12105,#12106,#12107,#12108,#12109,#12110,#12111,#12112,
#12113,#12114,#12115,#12116,#12117,#12118,#12119,#12120,#12121,#12122,#12123));
#12900=AXIS2_PLACEMENT_3D('',#21151,#14452,#14453);
#12901=AXIS2_PLACEMENT_3D('',#21400,#14454,#14455);
#12902=AXIS2_PLACEMENT_3D('',#21402,#14456,#14457);
#12903=AXIS2_PLACEMENT_3D('',#21404,#14458,#14459);
#12904=AXIS2_PLACEMENT_3D('',#21418,#14460,#14461);
#12905=AXIS2_PLACEMENT_3D('',#21419,#14462,#14463);
#12906=AXIS2_PLACEMENT_3D('',#21421,#14464,#14465);
#12907=AXIS2_PLACEMENT_3D('',#21437,#14466,#14467);
#12908=AXIS2_PLACEMENT_3D('',#21438,#14468,#14469);
#12909=AXIS2_PLACEMENT_3D('',#21692,#14471,#14472);
#12910=AXIS2_PLACEMENT_3D('',#21732,#14474,#14475);
#12911=AXIS2_PLACEMENT_3D('',#21734,#14476,#14477);
#12912=AXIS2_PLACEMENT_3D('',#21878,#14479,#14480);
#12913=AXIS2_PLACEMENT_3D('',#21880,#14481,#14482);
#12914=AXIS2_PLACEMENT_3D('',#21889,#14484,#14485);
#12915=AXIS2_PLACEMENT_3D('',#21915,#14486,#14487);
#12916=AXIS2_PLACEMENT_3D('',#21941,#14488,#14489);
#12917=AXIS2_PLACEMENT_3D('',#21967,#14490,#14491);
#12918=AXIS2_PLACEMENT_3D('',#21993,#14492,#14493);
#12919=AXIS2_PLACEMENT_3D('',#22019,#14494,#14495);
#12920=AXIS2_PLACEMENT_3D('',#22045,#14496,#14497);
#12921=AXIS2_PLACEMENT_3D('',#22071,#14498,#14499);
#12922=AXIS2_PLACEMENT_3D('',#22097,#14500,#14501);
#12923=AXIS2_PLACEMENT_3D('',#22122,#14502,#14503);
#12924=AXIS2_PLACEMENT_3D('',#22124,#14504,#14505);
#12925=AXIS2_PLACEMENT_3D('',#22150,#14506,#14507);
#12926=AXIS2_PLACEMENT_3D('',#22176,#14508,#14509);
#12927=AXIS2_PLACEMENT_3D('',#22202,#14510,#14511);
#12928=AXIS2_PLACEMENT_3D('',#22228,#14512,#14513);
#12929=AXIS2_PLACEMENT_3D('',#22254,#14514,#14515);
#12930=AXIS2_PLACEMENT_3D('',#22280,#14516,#14517);
#12931=AXIS2_PLACEMENT_3D('',#22306,#14518,#14519);
#12932=AXIS2_PLACEMENT_3D('',#22332,#14520,#14521);
#12933=AXIS2_PLACEMENT_3D('',#22358,#14522,#14523);
#12934=AXIS2_PLACEMENT_3D('',#22382,#14524,#14525);
#12935=AXIS2_PLACEMENT_3D('',#22384,#14526,#14527);
#12936=AXIS2_PLACEMENT_3D('',#22393,#14528,#14529);
#12937=AXIS2_PLACEMENT_3D('',#22403,#14530,#14531);
#12938=AXIS2_PLACEMENT_3D('',#22512,#14532,#14533);
#12939=AXIS2_PLACEMENT_3D('',#22522,#14534,#14535);
#12940=AXIS2_PLACEMENT_3D('',#22631,#14536,#14537);
#12941=AXIS2_PLACEMENT_3D('',#22641,#14538,#14539);
#12942=AXIS2_PLACEMENT_3D('',#22750,#14540,#14541);
#12943=AXIS2_PLACEMENT_3D('',#22760,#14542,#14543);
#12944=AXIS2_PLACEMENT_3D('',#22869,#14544,#14545);
#12945=AXIS2_PLACEMENT_3D('',#22879,#14546,#14547);
#12946=AXIS2_PLACEMENT_3D('',#22988,#14548,#14549);
#12947=AXIS2_PLACEMENT_3D('',#22998,#14550,#14551);
#12948=AXIS2_PLACEMENT_3D('',#23107,#14552,#14553);
#12949=AXIS2_PLACEMENT_3D('',#23117,#14554,#14555);
#12950=AXIS2_PLACEMENT_3D('',#23226,#14556,#14557);
#12951=AXIS2_PLACEMENT_3D('',#23236,#14558,#14559);
#12952=AXIS2_PLACEMENT_3D('',#23345,#14560,#14561);
#12953=AXIS2_PLACEMENT_3D('',#23355,#14562,#14563);
#12954=AXIS2_PLACEMENT_3D('',#23469,#14564,#14565);
#12955=AXIS2_PLACEMENT_3D('',#23479,#14566,#14567);
#12956=AXIS2_PLACEMENT_3D('',#23588,#14568,#14569);
#12957=AXIS2_PLACEMENT_3D('',#23598,#14570,#14571);
#12958=AXIS2_PLACEMENT_3D('',#23707,#14572,#14573);
#12959=AXIS2_PLACEMENT_3D('',#23717,#14574,#14575);
#12960=AXIS2_PLACEMENT_3D('',#23826,#14576,#14577);
#12961=AXIS2_PLACEMENT_3D('',#23836,#14578,#14579);
#12962=AXIS2_PLACEMENT_3D('',#23945,#14580,#14581);
#12963=AXIS2_PLACEMENT_3D('',#23955,#14582,#14583);
#12964=AXIS2_PLACEMENT_3D('',#24064,#14584,#14585);
#12965=AXIS2_PLACEMENT_3D('',#24074,#14586,#14587);
#12966=AXIS2_PLACEMENT_3D('',#24183,#14588,#14589);
#12967=AXIS2_PLACEMENT_3D('',#24193,#14590,#14591);
#12968=AXIS2_PLACEMENT_3D('',#24302,#14592,#14593);
#12969=AXIS2_PLACEMENT_3D('',#24312,#14594,#14595);
#12970=AXIS2_PLACEMENT_3D('',#24421,#14596,#14597);
#12971=AXIS2_PLACEMENT_3D('',#24431,#14598,#14599);
#12972=AXIS2_PLACEMENT_3D('',#24648,#14600,#14601);
#12973=AXIS2_PLACEMENT_3D('',#24650,#14602,#14603);
#12974=AXIS2_PLACEMENT_3D('',#24652,#14605,#14606);
#12975=AXIS2_PLACEMENT_3D('',#24653,#14607,#14608);
#12976=AXIS2_PLACEMENT_3D('',#24654,#14609,#14610);
#12977=AXIS2_PLACEMENT_3D('',#24655,#14611,#14612);
#12978=AXIS2_PLACEMENT_3D('',#24657,#14613,#14614);
#12979=AXIS2_PLACEMENT_3D('',#24658,#14615,#14616);
#12980=AXIS2_PLACEMENT_3D('',#24661,#14618,#14619);
#12981=AXIS2_PLACEMENT_3D('',#24662,#14620,#14621);
#12982=AXIS2_PLACEMENT_3D('',#24665,#14623,#14624);
#12983=AXIS2_PLACEMENT_3D('',#24666,#14625,#14626);
#12984=AXIS2_PLACEMENT_3D('',#24669,#14628,#14629);
#12985=AXIS2_PLACEMENT_3D('',#24670,#14630,#14631);
#14452=DIRECTION('axis',(0.,0.,1.));
#14453=DIRECTION('refdir',(1.,0.,0.));
#14454=DIRECTION('center_axis',(0.,0.,1.));
#14455=DIRECTION('ref_axis',(-0.707106781186547,-0.707106781186548,0.));
#14456=DIRECTION('center_axis',(0.,0.,1.));
#14457=DIRECTION('ref_axis',(1.,0.,0.));
#14458=DIRECTION('center_axis',(0.,0.,1.));
#14459=DIRECTION('ref_axis',(1.,0.,0.));
#14460=DIRECTION('center_axis',(0.,0.,1.));
#14461=DIRECTION('ref_axis',(1.,0.,0.));
#14462=DIRECTION('center_axis',(0.,0.,1.));
#14463=DIRECTION('ref_axis',(1.,0.,0.));
#14464=DIRECTION('center_axis',(0.,0.,1.));
#14465=DIRECTION('ref_axis',(1.,0.,0.));
#14466=DIRECTION('center_axis',(0.,0.,1.));
#14467=DIRECTION('ref_axis',(1.,0.,0.));
#14468=DIRECTION('center_axis',(-1.,0.,0.));
#14469=DIRECTION('ref_axis',(0.,0.,1.));
#14470=DIRECTION('',(-1.,0.,0.));
#14471=DIRECTION('center_axis',(6.12323399573677E-17,1.,0.));
#14472=DIRECTION('ref_axis',(1.7303891563162E-32,0.,1.));
#14473=DIRECTION('',(6.12323399573677E-17,1.,0.));
#14474=DIRECTION('center_axis',(0.,0.,-1.));
#14475=DIRECTION('ref_axis',(1.,0.,0.));
#14476=DIRECTION('center_axis',(0.,0.,1.));
#14477=DIRECTION('ref_axis',(1.,0.,0.));
#14478=DIRECTION('',(-0.707106781186546,-8.65956056235491E-17,-0.707106781186549));
#14479=DIRECTION('center_axis',(0.,0.,-1.));
#14480=DIRECTION('ref_axis',(1.,0.,0.));
#14481=DIRECTION('center_axis',(0.,0.,1.));
#14482=DIRECTION('ref_axis',(1.,0.,0.));
#14483=DIRECTION('',(-0.707106781186548,-8.65956056235493E-17,-0.707106781186548));
#14484=DIRECTION('center_axis',(0.,0.,1.));
#14485=DIRECTION('ref_axis',(1.,0.,0.));
#14486=DIRECTION('center_axis',(0.,0.,1.));
#14487=DIRECTION('ref_axis',(1.,0.,0.));
#14488=DIRECTION('center_axis',(0.,0.,1.));
#14489=DIRECTION('ref_axis',(1.,0.,0.));
#14490=DIRECTION('center_axis',(0.,0.,1.));
#14491=DIRECTION('ref_axis',(1.,0.,0.));
#14492=DIRECTION('center_axis',(0.,0.,1.));
#14493=DIRECTION('ref_axis',(1.,0.,0.));
#14494=DIRECTION('center_axis',(0.,0.,1.));
#14495=DIRECTION('ref_axis',(1.,0.,0.));
#14496=DIRECTION('center_axis',(0.,0.,1.));
#14497=DIRECTION('ref_axis',(1.,0.,0.));
#14498=DIRECTION('center_axis',(0.,0.,1.));
#14499=DIRECTION('ref_axis',(1.,0.,0.));
#14500=DIRECTION('center_axis',(0.,0.,1.));
#14501=DIRECTION('ref_axis',(1.,0.,0.));
#14502=DIRECTION('center_axis',(0.,0.,1.));
#14503=DIRECTION('ref_axis',(1.,0.,0.));
#14504=DIRECTION('center_axis',(0.,0.,1.));
#14505=DIRECTION('ref_axis',(1.,0.,0.));
#14506=DIRECTION('center_axis',(0.,0.,1.));
#14507=DIRECTION('ref_axis',(1.,0.,0.));
#14508=DIRECTION('center_axis',(0.,0.,1.));
#14509=DIRECTION('ref_axis',(1.,0.,0.));
#14510=DIRECTION('center_axis',(0.,0.,1.));
#14511=DIRECTION('ref_axis',(1.,0.,0.));
#14512=DIRECTION('center_axis',(0.,0.,1.));
#14513=DIRECTION('ref_axis',(1.,0.,0.));
#14514=DIRECTION('center_axis',(0.,0.,1.));
#14515=DIRECTION('ref_axis',(1.,0.,0.));
#14516=DIRECTION('center_axis',(0.,0.,1.));
#14517=DIRECTION('ref_axis',(1.,0.,0.));
#14518=DIRECTION('center_axis',(0.,0.,1.));
#14519=DIRECTION('ref_axis',(1.,0.,0.));
#14520=DIRECTION('center_axis',(0.,0.,1.));
#14521=DIRECTION('ref_axis',(1.,0.,0.));
#14522=DIRECTION('center_axis',(0.,0.,1.));
#14523=DIRECTION('ref_axis',(1.,0.,0.));
#14524=DIRECTION('center_axis',(0.,0.,1.));
#14525=DIRECTION('ref_axis',(1.,0.,0.));
#14526=DIRECTION('center_axis',(0.,0.,1.));
#14527=DIRECTION('ref_axis',(1.,0.,0.));
#14528=DIRECTION('center_axis',(0.,0.,1.));
#14529=DIRECTION('ref_axis',(1.,0.,0.));
#14530=DIRECTION('center_axis',(0.,0.,1.));
#14531=DIRECTION('ref_axis',(1.,0.,0.));
#14532=DIRECTION('center_axis',(0.,0.,1.));
#14533=DIRECTION('ref_axis',(1.,0.,0.));
#14534=DIRECTION('center_axis',(0.,0.,1.));
#14535=DIRECTION('ref_axis',(1.,0.,0.));
#14536=DIRECTION('center_axis',(0.,0.,1.));
#14537=DIRECTION('ref_axis',(1.,0.,0.));
#14538=DIRECTION('center_axis',(0.,0.,1.));
#14539=DIRECTION('ref_axis',(1.,0.,0.));
#14540=DIRECTION('center_axis',(0.,0.,1.));
#14541=DIRECTION('ref_axis',(1.,0.,0.));
#14542=DIRECTION('center_axis',(0.,0.,1.));
#14543=DIRECTION('ref_axis',(1.,0.,0.));
#14544=DIRECTION('center_axis',(0.,0.,1.));
#14545=DIRECTION('ref_axis',(1.,0.,0.));
#14546=DIRECTION('center_axis',(0.,0.,1.));
#14547=DIRECTION('ref_axis',(1.,0.,0.));
#14548=DIRECTION('center_axis',(0.,0.,1.));
#14549=DIRECTION('ref_axis',(1.,0.,0.));
#14550=DIRECTION('center_axis',(0.,0.,1.));
#14551=DIRECTION('ref_axis',(1.,0.,0.));
#14552=DIRECTION('center_axis',(0.,0.,1.));
#14553=DIRECTION('ref_axis',(1.,0.,0.));
#14554=DIRECTION('center_axis',(0.,0.,1.));
#14555=DIRECTION('ref_axis',(1.,0.,0.));
#14556=DIRECTION('center_axis',(0.,0.,1.));
#14557=DIRECTION('ref_axis',(1.,0.,0.));
#14558=DIRECTION('center_axis',(0.,0.,1.));
#14559=DIRECTION('ref_axis',(1.,0.,0.));
#14560=DIRECTION('center_axis',(0.,0.,1.));
#14561=DIRECTION('ref_axis',(1.,0.,0.));
#14562=DIRECTION('center_axis',(0.,0.,1.));
#14563=DIRECTION('ref_axis',(1.,0.,0.));
#14564=DIRECTION('center_axis',(0.,0.,1.));
#14565=DIRECTION('ref_axis',(-0.994427391317185,0.105423732613192,0.));
#14566=DIRECTION('center_axis',(0.,0.,1.));
#14567=DIRECTION('ref_axis',(1.,0.,0.));
#14568=DIRECTION('center_axis',(0.,0.,1.));
#14569=DIRECTION('ref_axis',(1.,0.,0.));
#14570=DIRECTION('center_axis',(0.,0.,1.));
#14571=DIRECTION('ref_axis',(1.,0.,0.));
#14572=DIRECTION('center_axis',(0.,0.,1.));
#14573=DIRECTION('ref_axis',(1.,0.,0.));
#14574=DIRECTION('center_axis',(0.,0.,1.));
#14575=DIRECTION('ref_axis',(1.,0.,0.));
#14576=DIRECTION('center_axis',(0.,0.,1.));
#14577=DIRECTION('ref_axis',(1.,0.,0.));
#14578=DIRECTION('center_axis',(0.,0.,1.));
#14579=DIRECTION('ref_axis',(1.,0.,0.));
#14580=DIRECTION('center_axis',(0.,0.,1.));
#14581=DIRECTION('ref_axis',(1.,0.,0.));
#14582=DIRECTION('center_axis',(0.,0.,1.));
#14583=DIRECTION('ref_axis',(1.,0.,0.));
#14584=DIRECTION('center_axis',(0.,0.,1.));
#14585=DIRECTION('ref_axis',(1.,0.,0.));
#14586=DIRECTION('center_axis',(0.,0.,1.));
#14587=DIRECTION('ref_axis',(1.,0.,0.));
#14588=DIRECTION('center_axis',(0.,0.,1.));
#14589=DIRECTION('ref_axis',(1.,0.,0.));
#14590=DIRECTION('center_axis',(0.,0.,1.));
#14591=DIRECTION('ref_axis',(1.,0.,0.));
#14592=DIRECTION('center_axis',(0.,0.,1.));
#14593=DIRECTION('ref_axis',(1.,0.,0.));
#14594=DIRECTION('center_axis',(0.,0.,1.));
#14595=DIRECTION('ref_axis',(1.,0.,0.));
#14596=DIRECTION('center_axis',(0.,0.,1.));
#14597=DIRECTION('ref_axis',(1.,0.,0.));
#14598=DIRECTION('center_axis',(0.,0.,1.));
#14599=DIRECTION('ref_axis',(1.,0.,0.));
#14600=DIRECTION('center_axis',(0.,0.,-1.));
#14601=DIRECTION('ref_axis',(1.,0.,0.));
#14602=DIRECTION('center_axis',(0.,0.,1.));
#14603=DIRECTION('ref_axis',(1.,0.,0.));
#14604=DIRECTION('',(-0.707106781186548,-8.65956056235493E-17,-0.707106781186548));
#14605=DIRECTION('center_axis',(0.,0.,1.));
#14606=DIRECTION('ref_axis',(1.,0.,0.));
#14607=DIRECTION('center_axis',(0.,0.,1.));
#14608=DIRECTION('ref_axis',(1.,0.,0.));
#14609=DIRECTION('center_axis',(0.,0.,1.));
#14610=DIRECTION('ref_axis',(1.,0.,0.));
#14611=DIRECTION('center_axis',(0.,0.,1.));
#14612=DIRECTION('ref_axis',(1.,0.,0.));
#14613=DIRECTION('center_axis',(0.,0.,1.));
#14614=DIRECTION('ref_axis',(1.,0.,0.));
#14615=DIRECTION('center_axis',(0.,0.,1.));
#14616=DIRECTION('ref_axis',(1.,0.,0.));
#14617=DIRECTION('',(0.707106781186547,8.65956056235493E-17,-0.707106781186547));
#14618=DIRECTION('center_axis',(0.,0.,1.));
#14619=DIRECTION('ref_axis',(1.,0.,0.));
#14620=DIRECTION('center_axis',(0.,0.,1.));
#14621=DIRECTION('ref_axis',(1.,0.,0.));
#14622=DIRECTION('',(0.,0.,-1.));
#14623=DIRECTION('center_axis',(0.,0.,1.));
#14624=DIRECTION('ref_axis',(1.,0.,0.));
#14625=DIRECTION('center_axis',(0.,0.,-1.));
#14626=DIRECTION('ref_axis',(1.,0.,0.));
#14627=DIRECTION('',(-0.70710678118655,-8.65956056235496E-17,-0.707106781186545));
#14628=DIRECTION('center_axis',(0.,0.,1.));
#14629=DIRECTION('ref_axis',(1.,0.,0.));
#14630=DIRECTION('center_axis',(0.,0.,-1.));
#14631=DIRECTION('ref_axis',(-1.,0.,0.));
#21151=CARTESIAN_POINT('',(0.,0.,0.));
#21152=CARTESIAN_POINT('Ctrl Pts',(0.999999999998244,-1.87406103457374E-6,
2.60499999999311));
#21153=CARTESIAN_POINT('Ctrl Pts',(1.00000006288704,0.033555619638003,2.60500024661583));
#21154=CARTESIAN_POINT('Ctrl Pts',(0.996432788538549,0.100793877077062,
2.59172126532562));
#21155=CARTESIAN_POINT('Ctrl Pts',(0.987779661769916,0.157562252712982,
2.55296011060328));
#21156=CARTESIAN_POINT('Ctrl Pts',(0.977968286593196,0.211192459212548,
2.49909481560466));
#21157=CARTESIAN_POINT('Ctrl Pts',(0.970281147530057,0.242238373929747,
2.44471009644067));
#21158=CARTESIAN_POINT('Ctrl Pts',(0.967388261055284,0.253317392831602,
2.37452193295668));
#21159=CARTESIAN_POINT('Ctrl Pts',(0.967116369990459,0.254356366300813,
2.34056467313598));
#21160=CARTESIAN_POINT('Ctrl Pts',(0.968060909182331,0.250746912814477,
2.30584393595531));
#21161=CARTESIAN_POINT('Ctrl Pts',(0.971275486994325,0.238235555290696,
2.25382796860057));
#21162=CARTESIAN_POINT('Ctrl Pts',(0.978160761261309,0.209370469448592,
2.20003517000389));
#21163=CARTESIAN_POINT('Ctrl Pts',(0.986928061083623,0.163194558725017,
2.1514224394046));
#21164=CARTESIAN_POINT('Ctrl Pts',(0.994800163464163,0.109016749833536,
2.11560611365411));
#21165=CARTESIAN_POINT('Ctrl Pts',(1.00003726905853,0.0393234864952561,
2.09484257852823));
#21166=CARTESIAN_POINT('Ctrl Pts',(1.00039359739908,-0.0285679116079913,
2.09347899005165));
#21167=CARTESIAN_POINT('Ctrl Pts',(0.995946129986918,-0.098499816085455,
2.11089539860567));
#21168=CARTESIAN_POINT('Ctrl Pts',(0.987595534630939,-0.160108842507484,
2.14787016428115));
#21169=CARTESIAN_POINT('Ctrl Pts',(0.978767296657426,-0.20640426202618,
2.19598850651528));
#21170=CARTESIAN_POINT('Ctrl Pts',(0.97062172581105,-0.241091125419321,
2.25963518301816));
#21171=CARTESIAN_POINT('Ctrl Pts',(0.967038345237899,-0.254607790735269,
2.32400532558939));
#21172=CARTESIAN_POINT('Ctrl Pts',(0.967372392238064,-0.253367892292085,
2.39214155711082));
#21173=CARTESIAN_POINT('Ctrl Pts',(0.971848592631414,-0.236216524025834,
2.45101723423612));
#21174=CARTESIAN_POINT('Ctrl Pts',(0.977999994055034,-0.208938409888944,
2.49656599568729));
#21175=CARTESIAN_POINT('Ctrl Pts',(0.982365078241419,-0.187417224408925,
2.52354132496555));
#21176=CARTESIAN_POINT('Ctrl Pts',(0.986694720178997,-0.163267539196543,
2.54663242388917));
#21177=CARTESIAN_POINT('Ctrl Pts',(0.99244571253526,-0.125541882265517,
2.57418619605903));
#21178=CARTESIAN_POINT('Ctrl Pts',(0.998300344088637,-0.0706101566680352,
2.59849422048893));
#21179=CARTESIAN_POINT('Ctrl Pts',(0.999999955756101,-0.0236095057558304,
2.60499982649452));
#21180=CARTESIAN_POINT('Ctrl Pts',(0.999999999998244,-1.87406103457374E-6,
2.60499999999311));
#21181=CARTESIAN_POINT('Ctrl Pts',(0.983333333331803,-1.72646341714646E-6,
2.58833333332708));
#21182=CARTESIAN_POINT('Ctrl Pts',(0.983325070408895,0.0309254949332375,
2.58831701644367));
#21183=CARTESIAN_POINT('Ctrl Pts',(0.980235431771385,0.0928701985922922,
2.5763334457126));
#21184=CARTESIAN_POINT('Ctrl Pts',(0.97262951086769,0.146010496479255,2.54070549738907));
#21185=CARTESIAN_POINT('Ctrl Pts',(0.963966193226361,0.196619990384259,
2.49071684326285));
#21186=CARTESIAN_POINT('Ctrl Pts',(0.957121635980358,0.226408216243534,
2.43967803502293));
#21187=CARTESIAN_POINT('Ctrl Pts',(0.954530758590317,0.237116103160976,
2.37322988185745));
#21188=CARTESIAN_POINT('Ctrl Pts',(0.954292056495262,0.238108034056394,
2.34106055897148));
#21189=CARTESIAN_POINT('Ctrl Pts',(0.955131698824161,0.234634460337268,
2.30818704053657));
#21190=CARTESIAN_POINT('Ctrl Pts',(0.958005717805603,0.222572733944937,
2.2590085409333));
#21191=CARTESIAN_POINT('Ctrl Pts',(0.964133168526514,0.194921019608955,
2.20849850875947));
#21192=CARTESIAN_POINT('Ctrl Pts',(0.971886775166395,0.151277899039362,
2.16333241887712));
#21193=CARTESIAN_POINT('Ctrl Pts',(0.978798486508062,0.100613721566294,
2.13040797264567));
#21194=CARTESIAN_POINT('Ctrl Pts',(0.983369400970407,0.0361963313628681,
2.11151394416968));
#21195=CARTESIAN_POINT('Ctrl Pts',(0.983676824334791,-0.0262950908417384,
2.11028422573118));
#21196=CARTESIAN_POINT('Ctrl Pts',(0.979801092832465,-0.0908603189323969,
2.12610656815928));
#21197=CARTESIAN_POINT('Ctrl Pts',(0.972473802924845,-0.148358154753562,
2.16004581981554));
#21198=CARTESIAN_POINT('Ctrl Pts',(0.964672149439096,-0.192110727398231,
2.20471275196644));
#21199=CARTESIAN_POINT('Ctrl Pts',(0.957427193110245,-0.225297504050057,
2.26446164543395));
#21200=CARTESIAN_POINT('Ctrl Pts',(0.954222830159563,-0.238355411074918,
2.32536038420973));
#21201=CARTESIAN_POINT('Ctrl Pts',(0.954522079095343,-0.2371523061421,2.3899277120541));
#21202=CARTESIAN_POINT('Ctrl Pts',(0.958517953243843,-0.220614507903057,
2.4455635357429));
#21203=CARTESIAN_POINT('Ctrl Pts',(0.963982071416956,-0.194581079725971,
2.48825477624319));
#21204=CARTESIAN_POINT('Ctrl Pts',(0.967849868185066,-0.174169675975904,
2.51340938027297));
#21205=CARTESIAN_POINT('Ctrl Pts',(0.97167321111088,-0.151401045973518,
2.53482806141593));
#21206=CARTESIAN_POINT('Ctrl Pts',(0.976733295652627,-0.116052309467583,
2.56023494607926));
#21207=CARTESIAN_POINT('Ctrl Pts',(0.981853837292877,-0.0650450913579237,
2.58243716495324));
#21208=CARTESIAN_POINT('Ctrl Pts',(0.983332905880957,-0.0217501188318965,
2.58833203941799));
#21209=CARTESIAN_POINT('Ctrl Pts',(0.983333333331803,-1.72646341714646E-6,
2.58833333332708));
#21210=CARTESIAN_POINT('Ctrl Pts',(0.966666666665363,-1.57886579971917E-6,
2.57166666666104));
#21211=CARTESIAN_POINT('Ctrl Pts',(0.966675031089233,0.0282574067618839,
2.57168340910161));
#21212=CARTESIAN_POINT('Ctrl Pts',(0.964030995123869,0.0849671350523733,
2.56092437077672));
#21213=CARTESIAN_POINT('Ctrl Pts',(0.957496079669552,0.134432741424285,
2.52848314020048));
#21214=CARTESIAN_POINT('Ctrl Pts',(0.949965488618089,0.18202293386404,2.48231761863255));
#21215=CARTESIAN_POINT('Ctrl Pts',(0.943960096058651,0.210589600813346,
2.4346289274524));
#21216=CARTESIAN_POINT('Ctrl Pts',(0.941686431722323,0.220882428486858,
2.3719223211333));
#21217=CARTESIAN_POINT('Ctrl Pts',(0.94146963989202,0.221854615130021,2.34155719007975));
#21218=CARTESIAN_POINT('Ctrl Pts',(0.942215861234142,0.218493014540143,
2.31051805593517));
#21219=CARTESIAN_POINT('Ctrl Pts',(0.944737453851974,0.206900615314252,
2.26419080172698));
#21220=CARTESIAN_POINT('Ctrl Pts',(0.950105713610565,0.180489574889026,
2.21697132240232));
#21221=CARTESIAN_POINT('Ctrl Pts',(0.956837948144641,0.139371349739201,
2.17526823220057));
#21222=CARTESIAN_POINT('Ctrl Pts',(0.962797300252717,0.0922406494407946,
2.14521214199563));
#21223=CARTESIAN_POINT('Ctrl Pts',(0.966692768725039,0.0330593334366949,
2.12821013824094));
#21224=CARTESIAN_POINT('Ctrl Pts',(0.966958180635997,-0.0240006511464648,
2.12709572724774));
#21225=CARTESIAN_POINT('Ctrl Pts',(0.963654605188848,-0.08321040561347,
2.1413234011611));
#21226=CARTESIAN_POINT('Ctrl Pts',(0.957353720921044,-0.136587098613656,
2.17220985324203));
#21227=CARTESIAN_POINT('Ctrl Pts',(0.950573235959199,-0.177820331414012,
2.21345060010943));
#21228=CARTESIAN_POINT('Ctrl Pts',(0.944223169736954,-0.209514123317684,
2.26930212368042));
#21229=CARTESIAN_POINT('Ctrl Pts',(0.941403959395846,-0.222103494504004,
2.32673583609555));
#21230=CARTESIAN_POINT('Ctrl Pts',(0.941667556372663,-0.220946133881027,
2.38772812706794));
#21231=CARTESIAN_POINT('Ctrl Pts',(0.945187704752525,-0.205008502652309,
2.44011245850097));
#21232=CARTESIAN_POINT('Ctrl Pts',(0.94997031235299,-0.180221173921234,
2.47994404421443));
#21233=CARTESIAN_POINT('Ctrl Pts',(0.953336718390379,-0.160920110206714,
2.5032802399603));
#21234=CARTESIAN_POINT('Ctrl Pts',(0.956651963018509,-0.139538170190601,
2.5230099883211));
#21235=CARTESIAN_POINT('Ctrl Pts',(0.961021973375283,-0.10656485199273,
2.54628159282629));
#21236=CARTESIAN_POINT('Ctrl Pts',(0.965409168116845,-0.0594989402485911,
2.56637680898634));
#21237=CARTESIAN_POINT('Ctrl Pts',(0.966667022710479,-0.0198905682807695,
2.57166766119149));
#21238=CARTESIAN_POINT('Ctrl Pts',(0.966666666665363,-1.57886579971917E-6,
2.57166666666104));
#21239=CARTESIAN_POINT('Ctrl Pts',(0.949999999998922,-1.43126818229188E-6,
2.554999999995));
#21240=CARTESIAN_POINT('Ctrl Pts',(0.950000038611092,0.0256272820571184,
2.55500017892945));
#21241=CARTESIAN_POINT('Ctrl Pts',(0.947833638356706,0.077043456567603,
2.5455365511637));
#21242=CARTESIAN_POINT('Ctrl Pts',(0.942345928767326,0.122880985190557,
2.51622852698627));
#21243=CARTESIAN_POINT('Ctrl Pts',(0.935963395251255,0.167450465035751,
2.47393964629074));
#21244=CARTESIAN_POINT('Ctrl Pts',(0.930800584508952,0.194759443127133,
2.42959686603466));
#21245=CARTESIAN_POINT('Ctrl Pts',(0.928828929257356,0.204681138816232,
2.37063027003408));
#21246=CARTESIAN_POINT('Ctrl Pts',(0.928645326396822,0.205606282885602,
2.34205307591525));
#21247=CARTESIAN_POINT('Ctrl Pts',(0.929286650875972,0.202380562062934,
2.31286116051643));
#21248=CARTESIAN_POINT('Ctrl Pts',(0.931467684663253,0.191237793968494,
2.26937137405972));
#21249=CARTESIAN_POINT('Ctrl Pts',(0.93607812087577,0.166040125049389,2.2254346611579));
#21250=CARTESIAN_POINT('Ctrl Pts',(0.941796662227414,0.127454690053546,
2.18717821167308));
#21251=CARTESIAN_POINT('Ctrl Pts',(0.946795623296616,0.0838376211735529,
2.16001400098719));
#21252=CARTESIAN_POINT('Ctrl Pts',(0.950024900636915,0.0299321783043069,
2.14488150388239));
#21253=CARTESIAN_POINT('Ctrl Pts',(0.950241407571709,-0.0217278303802119,
2.14390096292727));
#21254=CARTESIAN_POINT('Ctrl Pts',(0.947509568034395,-0.0755709084604119,
2.15653457071471));
#21255=CARTESIAN_POINT('Ctrl Pts',(0.942231989214949,-0.124836410859733,
2.18438550877642));
#21256=CARTESIAN_POINT('Ctrl Pts',(0.936478088740869,-0.163526796786063,
2.22217484556059));
#21257=CARTESIAN_POINT('Ctrl Pts',(0.931028637036149,-0.19372050194842,
2.27412858609622));
#21258=CARTESIAN_POINT('Ctrl Pts',(0.92858844431751,-0.205851114843653,
2.32809089471589));
#21259=CARTESIAN_POINT('Ctrl Pts',(0.928817243229942,-0.204730547731042,
2.38551428201123));
#21260=CARTESIAN_POINT('Ctrl Pts',(0.931857065364954,-0.189406486529532,
2.43465876000775));
#21261=CARTESIAN_POINT('Ctrl Pts',(0.935952389714912,-0.165863843758261,
2.47163282477033));
#21262=CARTESIAN_POINT('Ctrl Pts',(0.938821508334025,-0.147672561773693,
2.49314829526772));
#21263=CARTESIAN_POINT('Ctrl Pts',(0.941630453950392,-0.127671676967576,
2.51120562584786));
#21264=CARTESIAN_POINT('Ctrl Pts',(0.945309556492649,-0.0970752791947962,
2.53233034284651));
#21265=CARTESIAN_POINT('Ctrl Pts',(0.948962661321086,-0.0539338749384796,
2.55031975345065));
#21266=CARTESIAN_POINT('Ctrl Pts',(0.949999972835335,-0.0180311813568356,
2.55499987411497));
#21267=CARTESIAN_POINT('Ctrl Pts',(0.949999999998922,-1.43126818229188E-6,
2.554999999995));
#21268=CARTESIAN_POINT('',(0.998737211088938,0.0502392594122345,2.10000000017302));
#21269=CARTESIAN_POINT('',(0.998737211088938,-0.0502392594122345,2.10000000017302));
#21270=CARTESIAN_POINT('Ctrl Pts',(0.998741489349531,0.0501276226578845,
2.09998790761528));
#21271=CARTESIAN_POINT('Ctrl Pts',(0.998209106442774,0.0465065804968853,
2.0999823604152));
#21272=CARTESIAN_POINT('Ctrl Pts',(0.997731917482903,0.0428858888083561,
2.09997532142456));
#21273=CARTESIAN_POINT('Ctrl Pts',(0.99731100353809,0.0392650986878338,
2.09996763820277));
#21274=CARTESIAN_POINT('Ctrl Pts',(0.996973673612343,0.0363633158470504,
2.0999614806956));
#21275=CARTESIAN_POINT('Ctrl Pts',(0.996672480569791,0.0334615115052595,
2.09995491761494));
#21276=CARTESIAN_POINT('Ctrl Pts',(0.996408345014525,0.0305539602702526,
2.09994817558028));
#21277=CARTESIAN_POINT('Ctrl Pts',(0.995823734577335,0.0241186857880212,
2.09993325345505));
#21278=CARTESIAN_POINT('Ctrl Pts',(0.995422878237189,0.0176782325627147,
2.09991691990568));
#21279=CARTESIAN_POINT('Ctrl Pts',(0.995209369745946,0.0111608079949593,
2.0999080411453));
#21280=CARTESIAN_POINT('Ctrl Pts',(0.99514171218205,0.00909553618039141,
2.09990522760241));
#21281=CARTESIAN_POINT('Ctrl Pts',(0.995092895768509,0.00702412914613266,
2.09990323613576));
#21282=CARTESIAN_POINT('Ctrl Pts',(0.99506286554661,0.00494410069252508,
2.0999025509242));
#21283=CARTESIAN_POINT('Ctrl Pts',(0.99504459933955,0.00367890090298719,
2.09990213413686));
#21284=CARTESIAN_POINT('Ctrl Pts',(0.995033286585864,0.00241076308799952,
2.09990220272711));
#21285=CARTESIAN_POINT('Ctrl Pts',(0.995028899524127,0.00113911783449072,
2.09990288388685));
#21286=CARTESIAN_POINT('Ctrl Pts',(0.995024963884268,-1.67708640180092E-6,
2.09990349495629));
#21287=CARTESIAN_POINT('Ctrl Pts',(0.995026593989671,-0.00114513314823198,
2.09990463268876));
#21288=CARTESIAN_POINT('Ctrl Pts',(0.995033805529301,-0.00228459200009584,
2.09990622411078));
#21289=CARTESIAN_POINT('Ctrl Pts',(0.995042806799174,-0.00370683706316931,
2.09990821048536));
#21290=CARTESIAN_POINT('Ctrl Pts',(0.995060508292759,-0.00512536873273449,
2.09991087886862));
#21291=CARTESIAN_POINT('Ctrl Pts',(0.99508694937675,-0.00654097371496716,
2.0999140064208));
#21292=CARTESIAN_POINT('Ctrl Pts',(0.995138761674284,-0.00931490486528927,
2.09992013497682));
#21293=CARTESIAN_POINT('Ctrl Pts',(0.995224111395307,-0.0120760964135134,
2.09992800145899));
#21294=CARTESIAN_POINT('Ctrl Pts',(0.995343089287915,-0.0148303143798948,
2.09993619328405));
#21295=CARTESIAN_POINT('Ctrl Pts',(0.995539967164857,-0.0193878382523947,
2.09994974865211));
#21296=CARTESIAN_POINT('Ctrl Pts',(0.995828617967945,-0.0239182715715797,
2.09996404004403));
#21297=CARTESIAN_POINT('Ctrl Pts',(0.996207735735797,-0.0284458173699921,
2.09997472302851));
#21298=CARTESIAN_POINT('Ctrl Pts',(0.99631850279087,-0.0297686330154764,
2.09997784428219));
#21299=CARTESIAN_POINT('Ctrl Pts',(0.996436986832906,-0.0310911807891784,
2.09998067371155));
#21300=CARTESIAN_POINT('Ctrl Pts',(0.996563166797704,-0.0324135784390754,
2.09998318511707));
#21301=CARTESIAN_POINT('Ctrl Pts',(0.997133221361869,-0.0383878931186965,
2.09999453111945));
#21302=CARTESIAN_POINT('Ctrl Pts',(0.997858925779834,-0.0443424598651534,
2.09999902027607));
#21303=CARTESIAN_POINT('Ctrl Pts',(0.998734041876947,-0.0502864563072932,
2.0999972397247));
#21304=CARTESIAN_POINT('',(0.987458837468112,0.157876674357314,2.54999999999916));
#21305=CARTESIAN_POINT('Ctrl Pts',(0.998741489263531,0.0501276243402692,
2.09998790795724));
#21306=CARTESIAN_POINT('Ctrl Pts',(0.997746174412029,0.0695985876399753,
2.10394554683626));
#21307=CARTESIAN_POINT('Ctrl Pts',(0.994363645806935,0.112020975270126,
2.11759217250489));
#21308=CARTESIAN_POINT('Ctrl Pts',(0.986928061083623,0.163194558725017,
2.1514224394046));
#21309=CARTESIAN_POINT('Ctrl Pts',(0.978160761261309,0.209370469448592,
2.20003517000389));
#21310=CARTESIAN_POINT('Ctrl Pts',(0.971275486994325,0.238235555290696,
2.25382796860057));
#21311=CARTESIAN_POINT('Ctrl Pts',(0.968060909182331,0.250746912814477,
2.30584393595531));
#21312=CARTESIAN_POINT('Ctrl Pts',(0.967116369990459,0.254356366300813,
2.34056467313598));
#21313=CARTESIAN_POINT('Ctrl Pts',(0.967388261055284,0.253317392831602,
2.37452193295668));
#21314=CARTESIAN_POINT('Ctrl Pts',(0.970281147530057,0.242238373929747,
2.44471009644067));
#21315=CARTESIAN_POINT('Ctrl Pts',(0.977968286593196,0.211192459212548,
2.49909481560466));
#21316=CARTESIAN_POINT('Ctrl Pts',(0.98494013308223,0.173083472433883,2.53737085347425));
#21317=CARTESIAN_POINT('Ctrl Pts',(0.986199840262143,0.165761961406214,
2.54388428246999));
#21318=CARTESIAN_POINT('Ctrl Pts',(0.987440095705288,0.157976027584706,
2.55002758371622));
#21319=CARTESIAN_POINT('',(0.972500000001548,-1.63052496584468E-6,2.57749999999709));
#21320=CARTESIAN_POINT('Ctrl Pts',(0.987458837468451,0.157876674355192,
2.55));
#21321=CARTESIAN_POINT('Ctrl Pts',(0.985294697406766,0.146794280964263,
2.55388665064189));
#21322=CARTESIAN_POINT('Ctrl Pts',(0.983354421647032,0.135549889588831,
2.55740912752908));
#21323=CARTESIAN_POINT('Ctrl Pts',(0.977055328631449,0.0935709003424381,
2.56892572544489));
#21324=CARTESIAN_POINT('Ctrl Pts',(0.974161715360584,0.0622013742464855,
2.57437596695135));
#21325=CARTESIAN_POINT('Ctrl Pts',(0.972834706545006,0.0246194032981655,
2.57687004873351));
#21326=CARTESIAN_POINT('Ctrl Pts',(0.972691422895011,0.0189840464089377,
2.57713968402705));
#21327=CARTESIAN_POINT('Ctrl Pts',(0.972559701868467,0.0105124985263587,
2.57738760007473));
#21328=CARTESIAN_POINT('Ctrl Pts',(0.972529696233088,0.0076814295447408,
2.5774440907214));
#21329=CARTESIAN_POINT('Ctrl Pts',(0.972504563213093,0.00323267114025078,
2.57749140831944));
#21330=CARTESIAN_POINT('Ctrl Pts',(0.972499996930093,0.00161553516506767,
2.57750000577993));
#21331=CARTESIAN_POINT('Ctrl Pts',(0.972500000001548,-1.63052496584468E-6,
2.57749999999708));
#21332=CARTESIAN_POINT('',(0.949999999998922,-1.43126818229188E-6,2.554999999995));
#21333=CARTESIAN_POINT('Ctrl Pts',(0.972500000001548,-1.63052496584468E-6,
2.57749999999709));
#21334=CARTESIAN_POINT('Ctrl Pts',(0.965000000000673,-1.56410603799375E-6,
2.56999999999639));
#21335=CARTESIAN_POINT('Ctrl Pts',(0.957499999999797,-1.49768711014282E-6,
2.5624999999957));
#21336=CARTESIAN_POINT('Ctrl Pts',(0.949999999998922,-1.43126818229188E-6,
2.554999999995));
#21337=CARTESIAN_POINT('',(0.950017413548361,2.77722566314428E-6,2.14493017758226));
#21338=CARTESIAN_POINT('Ctrl Pts',(0.949999999998922,-1.43126818229188E-6,
2.554999999995));
#21339=CARTESIAN_POINT('Ctrl Pts',(0.950000038611092,0.0256272820571184,
2.55500017892945));
#21340=CARTESIAN_POINT('Ctrl Pts',(0.947833638356706,0.077043456567603,
2.5455365511637));
#21341=CARTESIAN_POINT('Ctrl Pts',(0.942345928767326,0.122880985190557,
2.51622852698627));
#21342=CARTESIAN_POINT('Ctrl Pts',(0.935963395251255,0.167450465035751,
2.47393964629074));
#21343=CARTESIAN_POINT('Ctrl Pts',(0.930800584508952,0.194759443127133,
2.42959686603466));
#21344=CARTESIAN_POINT('Ctrl Pts',(0.928828929257356,0.204681138816232,
2.37063027003408));
#21345=CARTESIAN_POINT('Ctrl Pts',(0.928645326396822,0.205606282885602,
2.34205307591525));
#21346=CARTESIAN_POINT('Ctrl Pts',(0.929286650875972,0.202380562062934,
2.31286116051643));
#21347=CARTESIAN_POINT('Ctrl Pts',(0.931467684663253,0.191237793968494,
2.26937137405972));
#21348=CARTESIAN_POINT('Ctrl Pts',(0.93607812087577,0.166040125049389,2.2254346611579));
#21349=CARTESIAN_POINT('Ctrl Pts',(0.941796662227414,0.127454690053546,
2.18717821167308));
#21350=CARTESIAN_POINT('Ctrl Pts',(0.946795623296616,0.0838376211735529,
2.16001400098719));
#21351=CARTESIAN_POINT('Ctrl Pts',(0.949571221584807,0.0375053185605399,
2.14700745845955));
#21352=CARTESIAN_POINT('Ctrl Pts',(0.950019209030419,0.0100740119424525,
2.1449223021834));
#21353=CARTESIAN_POINT('Ctrl Pts',(0.950017413548361,2.77722566314337E-6,
2.14493017758226));
#21354=CARTESIAN_POINT('Ctrl Pts',(0.950017413548361,2.77722566314337E-6,
2.14493017758226));
#21355=CARTESIAN_POINT('Ctrl Pts',(0.950016105516441,-0.0073342476264757,
2.14493591491227));
#21356=CARTESIAN_POINT('Ctrl Pts',(0.949714588734556,-0.0321111444056223,
2.14633727826451));
#21357=CARTESIAN_POINT('Ctrl Pts',(0.947509568034395,-0.0755709084604119,
2.15653457071471));
#21358=CARTESIAN_POINT('Ctrl Pts',(0.942231989214949,-0.124836410859733,
2.18438550877642));
#21359=CARTESIAN_POINT('Ctrl Pts',(0.936478088740869,-0.163526796786063,
2.22217484556059));
#21360=CARTESIAN_POINT('Ctrl Pts',(0.931028637036149,-0.19372050194842,
2.27412858609622));
#21361=CARTESIAN_POINT('Ctrl Pts',(0.92858844431751,-0.205851114843653,
2.32809089471589));
#21362=CARTESIAN_POINT('Ctrl Pts',(0.928817243229942,-0.204730547731042,
2.38551428201123));
#21363=CARTESIAN_POINT('Ctrl Pts',(0.931857065364954,-0.189406486529532,
2.43465876000775));
#21364=CARTESIAN_POINT('Ctrl Pts',(0.935952389714912,-0.165863843758261,
2.47163282477033));
#21365=CARTESIAN_POINT('Ctrl Pts',(0.938821508334025,-0.147672561773693,
2.49314829526772));
#21366=CARTESIAN_POINT('Ctrl Pts',(0.941630453950392,-0.127671676967576,
2.51120562584786));
#21367=CARTESIAN_POINT('Ctrl Pts',(0.945309556492649,-0.0970752791947962,
2.53233034284651));
#21368=CARTESIAN_POINT('Ctrl Pts',(0.948962661321086,-0.0539338749384796,
2.55031975345065));
#21369=CARTESIAN_POINT('Ctrl Pts',(0.949999972835335,-0.0180311813568356,
2.55499987411497));
#21370=CARTESIAN_POINT('Ctrl Pts',(0.949999999998922,-1.43126818229188E-6,
2.554999999995));
#21371=CARTESIAN_POINT('',(0.987458837468112,-0.157876674357314,2.54999999999916));
#21372=CARTESIAN_POINT('Ctrl Pts',(0.972500000001548,-1.63052496584468E-6,
2.57749999999708));
#21373=CARTESIAN_POINT('Ctrl Pts',(0.972500001100936,-0.00058047386256792,
2.57749999792719));
#21374=CARTESIAN_POINT('Ctrl Pts',(0.972500587629742,-0.00115932100720252,
2.5774988936244));
#21375=CARTESIAN_POINT('Ctrl Pts',(0.972506627935273,-0.00414265020170195,
2.57748752117621));
#21376=CARTESIAN_POINT('Ctrl Pts',(0.972521597304209,-0.00654688441944551,
2.57745933671442));
#21377=CARTESIAN_POINT('Ctrl Pts',(0.972586968658232,-0.0128156465435284,
2.57733627628346));
#21378=CARTESIAN_POINT('Ctrl Pts',(0.972653363288269,-0.016678636176991,
2.57721129835072));
#21379=CARTESIAN_POINT('Ctrl Pts',(0.972929256482295,-0.0281987946478753,
2.57669227394828));
#21380=CARTESIAN_POINT('Ctrl Pts',(0.973215079278776,-0.0358422720486581,
2.57615478699383));
#21381=CARTESIAN_POINT('Ctrl Pts',(0.974562717145952,-0.0623401377173552,
2.57362665221117));
#21382=CARTESIAN_POINT('Ctrl Pts',(0.976141626745025,-0.0810078079633483,
2.57067014303824));
#21383=CARTESIAN_POINT('Ctrl Pts',(0.980686505593143,-0.119336271682647,
2.56227318576719));
#21384=CARTESIAN_POINT('Ctrl Pts',(0.98374047439577,-0.138835225480723,
2.55667793110024));
#21385=CARTESIAN_POINT('Ctrl Pts',(0.987458837468451,-0.157876674355193,
2.55));
#21386=CARTESIAN_POINT('Ctrl Pts',(0.987454582400007,-0.157881308716372,
2.55005328965836));
#21387=CARTESIAN_POINT('Ctrl Pts',(0.987200786017512,-0.159467384180762,
2.5487918471679));
#21388=CARTESIAN_POINT('Ctrl Pts',(0.985506430965119,-0.169895526191808,
2.54029497054242));
#21389=CARTESIAN_POINT('Ctrl Pts',(0.982365078241419,-0.187417224408925,
2.52354132496555));
#21390=CARTESIAN_POINT('Ctrl Pts',(0.977999994055034,-0.208938409888944,
2.49656599568729));
#21391=CARTESIAN_POINT('Ctrl Pts',(0.971848592631414,-0.236216524025834,
2.45101723423612));
#21392=CARTESIAN_POINT('Ctrl Pts',(0.967372392238064,-0.253367892292085,
2.39214155711082));
#21393=CARTESIAN_POINT('Ctrl Pts',(0.967038345237899,-0.254607790735269,
2.32400532558939));
#21394=CARTESIAN_POINT('Ctrl Pts',(0.97062172581105,-0.241091125419321,
2.25963518301816));
#21395=CARTESIAN_POINT('Ctrl Pts',(0.978767296657426,-0.20640426202618,
2.19598850651528));
#21396=CARTESIAN_POINT('Ctrl Pts',(0.987595534630939,-0.160108842507484,
2.14787016428115));
#21397=CARTESIAN_POINT('Ctrl Pts',(0.995084474394307,-0.104856939129847,
2.11471063719305));
#21398=CARTESIAN_POINT('Ctrl Pts',(0.997930949375477,-0.066177461549665,
2.10319104189167));
#21399=CARTESIAN_POINT('Ctrl Pts',(0.998734041791771,-0.0502864579926989,
2.09999724006344));
#21400=CARTESIAN_POINT('Origin',(0.,0.,2.325));
#21401=CARTESIAN_POINT('',(-1.,-1.22464679914735E-16,2.55));
#21402=CARTESIAN_POINT('Origin',(0.,0.,2.55));
#21403=CARTESIAN_POINT('',(-0.157876674357314,0.987458837468112,2.54999999999916));
#21404=CARTESIAN_POINT('Origin',(0.,0.,2.55));
#21405=CARTESIAN_POINT('',(-0.0502392594122347,0.998737211088938,2.10000000017302));
#21406=CARTESIAN_POINT('Ctrl Pts',(-0.0501579437468834,0.998754980083996,
2.09996629680899));
#21407=CARTESIAN_POINT('Ctrl Pts',(-0.0826028085300709,0.997060472227549,
2.10669206239688));
#21408=CARTESIAN_POINT('Ctrl Pts',(-0.13333014615059,0.991871170579173,
2.12768221339602));
#21409=CARTESIAN_POINT('Ctrl Pts',(-0.184987608046235,0.98297944306662,
2.17252130019332));
#21410=CARTESIAN_POINT('Ctrl Pts',(-0.230530876255093,0.973454395083889,
2.2311541204646));
#21411=CARTESIAN_POINT('Ctrl Pts',(-0.255122284839583,0.966868905933786,
2.30756601931672));
#21412=CARTESIAN_POINT('Ctrl Pts',(-0.253875658998481,0.967246420818866,
2.38036927332879));
#21413=CARTESIAN_POINT('Ctrl Pts',(-0.237007380156922,0.971620587810882,
2.45580858562862));
#21414=CARTESIAN_POINT('Ctrl Pts',(-0.204967295321157,0.979117858283225,
2.50518732075992));
#21415=CARTESIAN_POINT('Ctrl Pts',(-0.173082478875929,0.984944804714717,
2.53735038518041));
#21416=CARTESIAN_POINT('Ctrl Pts',(-0.165770169783921,0.986201917446944,
2.54386940226406));
#21417=CARTESIAN_POINT('Ctrl Pts',(-0.157987843541269,0.987440871532657,
2.55001521460453));
#21418=CARTESIAN_POINT('Origin',(0.,0.,2.1));
#21419=CARTESIAN_POINT('Origin',(0.,0.,2.325));
#21420=CARTESIAN_POINT('',(0.0502392594122347,0.998737211088938,2.10000000017302));
#21421=CARTESIAN_POINT('Origin',(0.,0.,2.1));
#21422=CARTESIAN_POINT('',(0.157876674357314,0.987458837468112,2.54999999999916));
#21423=CARTESIAN_POINT('Ctrl Pts',(0.15787361447241,0.987459601094589,2.55002190145526));
#21424=CARTESIAN_POINT('Ctrl Pts',(0.159367603381274,0.987220783300611,
2.54883298459783));
#21425=CARTESIAN_POINT('Ctrl Pts',(0.16716148070395,0.985957317693993,2.54248953138653));
#21426=CARTESIAN_POINT('Ctrl Pts',(0.197782154055467,0.980628932028831,
2.51447081618292));
#21427=CARTESIAN_POINT('Ctrl Pts',(0.240862072091396,0.970821978192215,
2.45070211099161));
#21428=CARTESIAN_POINT('Ctrl Pts',(0.253753920072381,0.967257584978194,
2.38208598978509));
#21429=CARTESIAN_POINT('Ctrl Pts',(0.25377137321269,0.967257227319747,2.31770963275004));
#21430=CARTESIAN_POINT('Ctrl Pts',(0.247407872853293,0.96898626609141,2.28335835196792));
#21431=CARTESIAN_POINT('Ctrl Pts',(0.223542473616943,0.974765351154506,
2.22546113156583));
#21432=CARTESIAN_POINT('Ctrl Pts',(0.202625228604316,0.979486896662666,
2.19281789751093));
#21433=CARTESIAN_POINT('Ctrl Pts',(0.152664347670934,0.988739671565028,
2.14180432402534));
#21434=CARTESIAN_POINT('Ctrl Pts',(0.102949265500905,0.995581814195147,
2.11270476782457));
#21435=CARTESIAN_POINT('Ctrl Pts',(0.0581205001812461,0.998362457461274,
2.10152203482183));
#21436=CARTESIAN_POINT('Ctrl Pts',(0.0502611231985831,0.998755291180234,
2.09995263652274));
#21437=CARTESIAN_POINT('Origin',(0.,0.,2.55));
#21438=CARTESIAN_POINT('Origin',(0.705,0.,2.35));
#21439=CARTESIAN_POINT('',(0.501,-1.25526296912604E-17,2.145));
#21440=CARTESIAN_POINT('',(0.705,-2.51052593825207E-17,2.145));
#21441=CARTESIAN_POINT('',(0.457138928554548,-0.205,2.35));
#21442=CARTESIAN_POINT('Ctrl Pts',(0.457138928554548,-0.205,2.35));
#21443=CARTESIAN_POINT('Ctrl Pts',(0.457138928554548,-0.205,2.32390927987453));
#21444=CARTESIAN_POINT('Ctrl Pts',(0.459609069157102,-0.199722778787908,
2.29632432035936));
#21445=CARTESIAN_POINT('Ctrl Pts',(0.468177727272261,-0.178715671123715,
2.24592797085052));
#21446=CARTESIAN_POINT('Ctrl Pts',(0.474117890962221,-0.162998335554875,
2.22308455526839));
#21447=CARTESIAN_POINT('Ctrl Pts',(0.485018345626291,-0.126935588134045,
2.18702180784756));
#21448=CARTESIAN_POINT('Ctrl Pts',(0.490733376060334,-0.104084611878653,
2.17128923329376));
#21449=CARTESIAN_POINT('Ctrl Pts',(0.498772107838147,-0.0536585253249439,
2.1502704112139));
#21450=CARTESIAN_POINT('Ctrl Pts',(0.501,-0.0260615896504235,2.145));
#21451=CARTESIAN_POINT('Ctrl Pts',(0.501,-6.24500451351651E-17,2.145));
#21452=CARTESIAN_POINT('Ctrl Pts',(0.501,0.,2.145));
#21453=CARTESIAN_POINT('Ctrl Pts',(0.501,0.0260615896504235,2.145));
#21454=CARTESIAN_POINT('Ctrl Pts',(0.498772107838147,0.0536585253249438,
2.1502704112139));
#21455=CARTESIAN_POINT('Ctrl Pts',(0.490733376060334,0.104084611878653,
2.17128923329376));
#21456=CARTESIAN_POINT('Ctrl Pts',(0.485018345626291,0.126935588134045,
2.18702180784756));
#21457=CARTESIAN_POINT('Ctrl Pts',(0.474117890962221,0.162998335554875,
2.22308455526839));
#21458=CARTESIAN_POINT('Ctrl Pts',(0.468177727272261,0.178715671123715,
2.24592797085052));
#21459=CARTESIAN_POINT('Ctrl Pts',(0.459609069157102,0.199722778787908,
2.29632432035936));
#21460=CARTESIAN_POINT('Ctrl Pts',(0.457138928554548,0.205,2.32390927987453));
#21461=CARTESIAN_POINT('Ctrl Pts',(0.457138928554548,0.205,2.37609072012547));
#21462=CARTESIAN_POINT('Ctrl Pts',(0.459609069157102,0.199722778787908,
2.40367567964064));
#21463=CARTESIAN_POINT('Ctrl Pts',(0.468177727272261,0.178715671123715,
2.45407202914948));
#21464=CARTESIAN_POINT('Ctrl Pts',(0.474117890962221,0.162998335554875,
2.47691544473161));
#21465=CARTESIAN_POINT('Ctrl Pts',(0.485018345626291,0.126935588134045,
2.51297819215244));
#21466=CARTESIAN_POINT('Ctrl Pts',(0.490733376060334,0.104084611878653,
2.52871076670624));
#21467=CARTESIAN_POINT('Ctrl Pts',(0.498772107838147,0.0536585253249439,
2.5497295887861));
#21468=CARTESIAN_POINT('Ctrl Pts',(0.501,0.0260615896504235,2.555));
#21469=CARTESIAN_POINT('Ctrl Pts',(0.501,-0.0260615896504234,2.555));
#21470=CARTESIAN_POINT('Ctrl Pts',(0.498772107838147,-0.0536585253249438,
2.5497295887861));
#21471=CARTESIAN_POINT('Ctrl Pts',(0.490733376060334,-0.104084611878653,
2.52871076670624));
#21472=CARTESIAN_POINT('Ctrl Pts',(0.485018345626291,-0.126935588134045,
2.51297819215244));
#21473=CARTESIAN_POINT('Ctrl Pts',(0.474117890962222,-0.162998335554875,
2.47691544473161));
#21474=CARTESIAN_POINT('Ctrl Pts',(0.468177727272261,-0.178715671123715,
2.45407202914948));
#21475=CARTESIAN_POINT('Ctrl Pts',(0.459609069157102,-0.199722778787908,
2.40367567964064));
#21476=CARTESIAN_POINT('Ctrl Pts',(0.457138928554548,-0.205,2.37609072012547));
#21477=CARTESIAN_POINT('Ctrl Pts',(0.457138928554548,-0.205,2.35));
#21478=CARTESIAN_POINT('Ctrl Pts',(1.8740610339731E-6,0.999999999998244,
2.60499999999311));
#21479=CARTESIAN_POINT('Ctrl Pts',(-0.0335556196380034,1.00000006288704,
2.60500024661583));
#21480=CARTESIAN_POINT('Ctrl Pts',(-0.100756673071006,0.996441174833638,
2.59168345968582));
#21481=CARTESIAN_POINT('Ctrl Pts',(-0.157603488695687,0.98777358833807,
2.55296445525625));
#21482=CARTESIAN_POINT('Ctrl Pts',(-0.204967295321157,0.979117858283225,
2.50518732075992));
#21483=CARTESIAN_POINT('Ctrl Pts',(-0.237007380156922,0.971620587810882,
2.45580858562862));
#21484=CARTESIAN_POINT('Ctrl Pts',(-0.253875658998481,0.967246420818866,
2.38036927332879));
#21485=CARTESIAN_POINT('Ctrl Pts',(-0.255122284839583,0.966868905933786,
2.30756601931672));
#21486=CARTESIAN_POINT('Ctrl Pts',(-0.230530876255093,0.973454395083889,
2.2311541204646));
#21487=CARTESIAN_POINT('Ctrl Pts',(-0.184987608046235,0.98297944306662,
2.17252130019332));
#21488=CARTESIAN_POINT('Ctrl Pts',(-0.130000247114384,0.992444341497521,
2.12479183461179));
#21489=CARTESIAN_POINT('Ctrl Pts',(-0.0547900546441262,0.999800917250482,
2.09586490599377));
#21490=CARTESIAN_POINT('Ctrl Pts',(0.00901292386013043,1.00025490450459,
2.09401178448709));
#21491=CARTESIAN_POINT('Ctrl Pts',(0.0460479466138129,0.999088187246804,
2.09861314679373));
#21492=CARTESIAN_POINT('Ctrl Pts',(0.101662133244068,0.995758958476132,
2.11195137517568));
#21493=CARTESIAN_POINT('Ctrl Pts',(0.152664347670934,0.988739671565028,
2.14180432402534));
#21494=CARTESIAN_POINT('Ctrl Pts',(0.202625228604316,0.979486896662666,
2.19281789751093));
#21495=CARTESIAN_POINT('Ctrl Pts',(0.223542473616943,0.974765351154506,
2.22546113156583));
#21496=CARTESIAN_POINT('Ctrl Pts',(0.247407872853293,0.96898626609141,2.28335835196792));
#21497=CARTESIAN_POINT('Ctrl Pts',(0.25377137321269,0.967257227319747,2.31770963275004));
#21498=CARTESIAN_POINT('Ctrl Pts',(0.253753920072381,0.967257584978194,
2.38208598978509));
#21499=CARTESIAN_POINT('Ctrl Pts',(0.240862072091396,0.970821978192215,
2.45070211099161));
#21500=CARTESIAN_POINT('Ctrl Pts',(0.197782154055467,0.980628932028831,
2.51447081618292));
#21501=CARTESIAN_POINT('Ctrl Pts',(0.16267570908935,0.986737898868484,2.54659412947604));
#21502=CARTESIAN_POINT('Ctrl Pts',(0.136234199434897,0.990851168416345,
2.56664374352278));
#21503=CARTESIAN_POINT('Ctrl Pts',(0.0840473157184407,0.997329420352096,
2.59494454511583));
#21504=CARTESIAN_POINT('Ctrl Pts',(0.03365753814838,0.999999936925475,2.60499975264892));
#21505=CARTESIAN_POINT('Ctrl Pts',(1.8740610339731E-6,0.999999999998244,
2.60499999999311));
#21506=CARTESIAN_POINT('Ctrl Pts',(1.72646341657069E-6,0.983333333331803,
2.58833333332708));
#21507=CARTESIAN_POINT('Ctrl Pts',(-0.0309211194933883,0.983327802047045,
2.58831966882739));
#21508=CARTESIAN_POINT('Ctrl Pts',(-0.0928377960476621,0.98023976768212,
2.57629404074584));
#21509=CARTESIAN_POINT('Ctrl Pts',(-0.146048423576797,0.972626976944164,
2.54070953195264));
#21510=CARTESIAN_POINT('Ctrl Pts',(-0.190747496194426,0.964977664234015,
2.49636747507197));
#21511=CARTESIAN_POINT('Ctrl Pts',(-0.221374849129247,0.95831490086092,
2.45011538765543));
#21512=CARTESIAN_POINT('Ctrl Pts',(-0.237650481571607,0.954402200933291,
2.37878285196974));
#21513=CARTESIAN_POINT('Ctrl Pts',(-0.238858199349336,0.954071300725052,
2.30977107620483));
#21514=CARTESIAN_POINT('Ctrl Pts',(-0.215099921034606,0.959955138122488,
2.23759648199501));
#21515=CARTESIAN_POINT('Ctrl Pts',(-0.17183883952112,0.968399947196108,
2.18290355895676));
#21516=CARTESIAN_POINT('Ctrl Pts',(-0.120099054224975,0.976743248230922,
2.13876052168788));
#21517=CARTESIAN_POINT('Ctrl Pts',(-0.0504163434655785,0.983158893045571,
2.11245900795287));
#21518=CARTESIAN_POINT('Ctrl Pts',(0.00827833993718029,0.983561344274991,
2.1107555539468));
#21519=CARTESIAN_POINT('Ctrl Pts',(0.0424518621317906,0.982538668939213,
2.11495120932668));
#21520=CARTESIAN_POINT('Ctrl Pts',(0.0937720299455498,0.979640570051344,
2.12707976132422));
#21521=CARTESIAN_POINT('Ctrl Pts',(0.141360481904814,0.973477223378796,
2.15443787690997));
#21522=CARTESIAN_POINT('Ctrl Pts',(0.188538345234594,0.965310317630362,
2.20179163355866));
#21523=CARTESIAN_POINT('Ctrl Pts',(0.208490757001602,0.961105657569896,
2.23236164151278));
#21524=CARTESIAN_POINT('Ctrl Pts',(0.231400254955185,0.955964354544338,
2.28688145033855));
#21525=CARTESIAN_POINT('Ctrl Pts',(0.237544330067899,0.954413219989739,
2.31941255684048));
#21526=CARTESIAN_POINT('Ctrl Pts',(0.237537755869605,0.954418441564086,
2.38038851320367));
#21527=CARTESIAN_POINT('Ctrl Pts',(0.225032695661137,0.957606932779055,
2.44537253850971));
#21528=CARTESIAN_POINT('Ctrl Pts',(0.183910350012796,0.966318757498156,
2.50501316984723));
#21529=CARTESIAN_POINT('Ctrl Pts',(0.150857782836235,0.971711641804196,
2.53478061849988));
#21530=CARTESIAN_POINT('Ctrl Pts',(0.126062259734711,0.975331110231934,
2.55328561568025));
#21531=CARTESIAN_POINT('Ctrl Pts',(0.0774389729843563,0.981016367853088,
2.57924416260037));
#21532=CARTESIAN_POINT('Ctrl Pts',(0.0310095625324942,0.983324489370319,
2.58831441049439));
#21533=CARTESIAN_POINT('Ctrl Pts',(1.72646341657069E-6,0.983333333331803,
2.58833333332708));
#21534=CARTESIAN_POINT('Ctrl Pts',(1.57886579916828E-6,0.966666666665363,
2.57166666666104));
#21535=CARTESIAN_POINT('Ctrl Pts',(-0.028261782201734,0.966672299451083,
2.57168075671789));
#21536=CARTESIAN_POINT('Ctrl Pts',(-0.0849369725180309,0.964038061600584,
2.56088137505698));
#21537=CARTESIAN_POINT('Ctrl Pts',(-0.134467081311291,0.957489301980934,
2.52849464185));
#21538=CARTESIAN_POINT('Ctrl Pts',(-0.176493077367449,0.950850885491106,
2.48751717131812));
#21539=CARTESIAN_POINT('Ctrl Pts',(-0.205749279945383,0.945011607194673,
2.44443170330968));
#21540=CARTESIAN_POINT('Ctrl Pts',(-0.221405615759076,0.941576404880082,
2.37718285612148));
#21541=CARTESIAN_POINT('Ctrl Pts',(-0.222592256095046,0.941273043800734,
2.31198020634687));
#21542=CARTESIAN_POINT('Ctrl Pts',(-0.19967059846768,0.946452066132863,
2.24404982314633));
#21543=CARTESIAN_POINT('Ctrl Pts',(-0.158679713896286,0.953815819341673,
2.19329233666131));
#21544=CARTESIAN_POINT('Ctrl Pts',(-0.110198993644362,0.961036297799555,
2.15273846356872));
#21545=CARTESIAN_POINT('Ctrl Pts',(-0.046075343884759,0.966525769606431,
2.12903238312702));
#21546=CARTESIAN_POINT('Ctrl Pts',(0.00757919676247354,0.966850980745995,
2.12753983018364));
#21547=CARTESIAN_POINT('Ctrl Pts',(0.0388114474174279,0.965990205488828,
2.13128917659776));
#21548=CARTESIAN_POINT('Ctrl Pts',(0.0859427838572395,0.963505820548163,
2.14224095850635));
#21549=CARTESIAN_POINT('Ctrl Pts',(0.130095057847622,0.958228990545236,
2.16703937038342));
#21550=CARTESIAN_POINT('Ctrl Pts',(0.17448083867517,0.95111834103327,2.21079555546396));
#21551=CARTESIAN_POINT('Ctrl Pts',(0.193473476747956,0.947464227672504,
2.23924962741081));
#21552=CARTESIAN_POINT('Ctrl Pts',(0.215362766008526,0.942940862740997,
2.29040473546289));
#21553=CARTESIAN_POINT('Ctrl Pts',(0.221328116324425,0.941582271034106,
2.32111335094323));
#21554=CARTESIAN_POINT('Ctrl Pts',(0.221307475198179,0.941576462552143,
2.37869131092512));
#21555=CARTESIAN_POINT('Ctrl Pts',(0.209212867982546,0.944395419867102,
2.44004063866257));
#21556=CARTESIAN_POINT('Ctrl Pts',(0.170035598298793,0.952016482602868,
2.49557168347949));
#21557=CARTESIAN_POINT('Ctrl Pts',(0.139037988014577,0.956682144907831,
2.52295666497662));
#21558=CARTESIAN_POINT('Ctrl Pts',(0.115891644338605,0.959813980610051,
2.53993061096407));
#21559=CARTESIAN_POINT('Ctrl Pts',(0.0708540967431303,0.964686661475804,
2.56350215110508));
#21560=CARTESIAN_POINT('Ctrl Pts',(0.0283530954373026,0.96667540882895,
2.57168516269162));
#21561=CARTESIAN_POINT('Ctrl Pts',(1.57886579916828E-6,0.966666666665363,
2.57166666666104));
#21562=CARTESIAN_POINT('Ctrl Pts',(1.43126818176587E-6,0.949999999998922,
2.554999999995));
#21563=CARTESIAN_POINT('Ctrl Pts',(-0.0256272820571188,0.950000038611092,
2.55500017892945));
#21564=CARTESIAN_POINT('Ctrl Pts',(-0.0770180954946874,0.947836654449066,
2.545491956117));
#21565=CARTESIAN_POINT('Ctrl Pts',(-0.122912016192401,0.942342690587028,
2.51623971854639));
#21566=CARTESIAN_POINT('Ctrl Pts',(-0.162273278240718,0.936710691441896,
2.47869732563017));
#21567=CARTESIAN_POINT('Ctrl Pts',(-0.190116748917708,0.931705920244711,
2.43873850533649));
#21568=CARTESIAN_POINT('Ctrl Pts',(-0.205180438332203,0.928732184994508,
2.37559643476243));
#21569=CARTESIAN_POINT('Ctrl Pts',(-0.2063281706048,0.928475438592001,2.31418526323498));
#21570=CARTESIAN_POINT('Ctrl Pts',(-0.184239643247193,0.932952809171462,
2.25049218467674));
#21571=CARTESIAN_POINT('Ctrl Pts',(-0.14553094537117,0.939236323471161,
2.20367459542476));
#21572=CARTESIAN_POINT('Ctrl Pts',(-0.100297800754953,0.945335204532955,
2.16670715064481));
#21573=CARTESIAN_POINT('Ctrl Pts',(-0.0417016327062113,0.94988374540152,
2.14562648508612));
#21574=CARTESIAN_POINT('Ctrl Pts',(0.0068446128395234,0.950157420516395,
2.14428359964335));
#21575=CARTESIAN_POINT('Ctrl Pts',(0.0352153629354055,0.949440687181237,
2.14762723913071));
#21576=CARTESIAN_POINT('Ctrl Pts',(0.0780526805587212,0.947387432123376,
2.15736934465489));
#21577=CARTESIAN_POINT('Ctrl Pts',(0.118791192081503,0.942966542359005,
2.17967292326805));
#21578=CARTESIAN_POINT('Ctrl Pts',(0.160393955305448,0.936941762000965,
2.2197692915117));
#21579=CARTESIAN_POINT('Ctrl Pts',(0.178421760132616,0.933804534087895,
2.24615013735776));
#21580=CARTESIAN_POINT('Ctrl Pts',(0.199355148110418,0.929918951193924,
2.29392783383353));
#21581=CARTESIAN_POINT('Ctrl Pts',(0.205101073179634,0.928738263704097,
2.32281627503367));
#21582=CARTESIAN_POINT('Ctrl Pts',(0.205091310995403,0.928737319138035,
2.3769938343437));
#21583=CARTESIAN_POINT('Ctrl Pts',(0.193383491552286,0.931180374453942,
2.43471106618067));
#21584=CARTESIAN_POINT('Ctrl Pts',(0.156163794256122,0.937706308072193,
2.4861140371438));
#21585=CARTESIAN_POINT('Ctrl Pts',(0.127220061761462,0.941655887843543,
2.51114315400046));
#21586=CARTESIAN_POINT('Ctrl Pts',(0.105719704638418,0.944293922425639,
2.52657248312153));
#21587=CARTESIAN_POINT('Ctrl Pts',(0.0642457540090459,0.948373608976796,
2.54780176858962));
#21588=CARTESIAN_POINT('Ctrl Pts',(0.0257051198214169,0.949999961273794,
2.55499982053709));
#21589=CARTESIAN_POINT('Ctrl Pts',(1.43126818176587E-6,0.949999999998922,
2.554999999995));
#21590=CARTESIAN_POINT('Ctrl Pts',(-0.0501579420662037,0.998754980171774,
2.09996629646059));
#21591=CARTESIAN_POINT('Ctrl Pts',(-0.0455541516249309,0.998081971740583,
2.09994285225375));
#21592=CARTESIAN_POINT('Ctrl Pts',(-0.0409493960495382,0.997497248478843,
2.09992115702739));
#21593=CARTESIAN_POINT('Ctrl Pts',(-0.0363408599228962,0.997001962981805,
2.0999069394429));
#21594=CARTESIAN_POINT('Ctrl Pts',(-0.0344254769968775,0.996796114235378,
2.09990103038244));
#21595=CARTESIAN_POINT('Ctrl Pts',(-0.0325094393882293,0.996605701141417,
2.09989644467646));
#21596=CARTESIAN_POINT('Ctrl Pts',(-0.030591027199469,0.996431064903213,
2.0998929904383));
#21597=CARTESIAN_POINT('Ctrl Pts',(-0.0241570348712139,0.995845367927649,
2.09988140557563));
#21598=CARTESIAN_POINT('Ctrl Pts',(-0.0177195435991528,0.995439341015549,
2.09988208911745));
#21599=CARTESIAN_POINT('Ctrl Pts',(-0.0112042061332443,0.99522006377236,
2.09989207709953));
#21600=CARTESIAN_POINT('Ctrl Pts',(-0.0091395956891891,0.995150578179511,
2.09989524213775));
#21601=CARTESIAN_POINT('Ctrl Pts',(-0.00706875291999245,0.995099879623312,
2.09989939288935));
#21602=CARTESIAN_POINT('Ctrl Pts',(-0.00498909077113959,0.995068038205673,
2.09990458544879));
#21603=CARTESIAN_POINT('Ctrl Pts',(-0.00372411379059672,0.995048670319229,
2.09990774387919));
#21604=CARTESIAN_POINT('Ctrl Pts',(-0.00245612535390708,0.995036282497343,
2.09991128863539));
#21605=CARTESIAN_POINT('Ctrl Pts',(-0.00118453247084987,0.995030876493846,
2.09991524595687));
#21606=CARTESIAN_POINT('Ctrl Pts',(-4.37845315938809E-5,0.995026026759759,
2.09991879607608));
#21607=CARTESIAN_POINT('Ctrl Pts',(0.00109970303547405,0.995026788370882,
2.09992271042795));
#21608=CARTESIAN_POINT('Ctrl Pts',(0.00223928716687367,0.995033203141033,
2.09992682811702));
#21609=CARTESIAN_POINT('Ctrl Pts',(0.0036616886009847,0.995041209902455,
2.09993196771721));
#21610=CARTESIAN_POINT('Ctrl Pts',(0.00508052255109117,0.995058026539435,
2.09993740601942));
#21611=CARTESIAN_POINT('Ctrl Pts',(0.00649660255618722,0.99508373088496,
2.09994278957186));
#21612=CARTESIAN_POINT('Ctrl Pts',(0.00927146453168093,0.99513409951579,
2.09995333884513));
#21613=CARTESIAN_POINT('Ctrl Pts',(0.0120342525028786,0.995218575771198,
2.09996364717532));
#21614=CARTESIAN_POINT('Ctrl Pts',(0.0147909036437984,0.995337528356299,
2.0999713663429));
#21615=CARTESIAN_POINT('Ctrl Pts',(0.0158423647792016,0.995382900082279,
2.09997431064172));
#21616=CARTESIAN_POINT('Ctrl Pts',(0.0168924947237524,0.995433267490783,
2.09997688114622));
#21617=CARTESIAN_POINT('Ctrl Pts',(0.0179416114429507,0.995488633595717,
2.09997896362948));
#21618=CARTESIAN_POINT('Ctrl Pts',(0.0227736532195703,0.995743639856846,
2.09998855517054));
#21619=CARTESIAN_POINT('Ctrl Pts',(0.027584328345019,0.996104743818564,
2.09998770209067));
#21620=CARTESIAN_POINT('Ctrl Pts',(0.0323893668042188,0.996568206430001,
2.09998210436156));
#21621=CARTESIAN_POINT('Ctrl Pts',(0.0368950513274315,0.997002795316889,
2.09997685537102));
#21622=CARTESIAN_POINT('Ctrl Pts',(0.0413861399780065,0.997526459114176,
2.09996745668706));
#21623=CARTESIAN_POINT('Ctrl Pts',(0.0458741854723339,0.99813430097851,
2.09995967180744));
#21624=CARTESIAN_POINT('Ctrl Pts',(0.0473368418337277,0.998332396958311,
2.09995713471112));
#21625=CARTESIAN_POINT('Ctrl Pts',(0.0487991635875438,0.99853942952464,
2.09995477525694));
#21626=CARTESIAN_POINT('Ctrl Pts',(0.0502611215119263,0.998755291264538,
2.09995263618594));
#21627=CARTESIAN_POINT('',(1.63052496528509E-6,0.972500000001548,2.57749999999709));
#21628=CARTESIAN_POINT('Ctrl Pts',(-0.157876674355192,0.987458837468451,
2.55));
#21629=CARTESIAN_POINT('Ctrl Pts',(-0.14679428096426,0.985294697406766,
2.55388665064189));
#21630=CARTESIAN_POINT('Ctrl Pts',(-0.135549889588828,0.983354421647031,
2.55740912752908));
#21631=CARTESIAN_POINT('Ctrl Pts',(-0.0935709003424397,0.977055328631449,
2.56892572544489));
#21632=CARTESIAN_POINT('Ctrl Pts',(-0.062201374246487,0.974161715360584,
2.57437596695135));
#21633=CARTESIAN_POINT('Ctrl Pts',(-0.024619403298166,0.972834706545006,
2.57687004873351));
#21634=CARTESIAN_POINT('Ctrl Pts',(-0.0189840464089389,0.972691422895011,
2.57713968402705));
#21635=CARTESIAN_POINT('Ctrl Pts',(-0.0105124985263454,0.972559701868467,
2.57738760007473));
#21636=CARTESIAN_POINT('Ctrl Pts',(-0.00768142954473445,0.972529696233088,
2.5774440907214));
#21637=CARTESIAN_POINT('Ctrl Pts',(-0.0032326711402507,0.972504563213093,
2.57749140831944));
#21638=CARTESIAN_POINT('Ctrl Pts',(-0.0016155351650678,0.972499996930093,
2.57750000577993));
#21639=CARTESIAN_POINT('Ctrl Pts',(1.63052496528509E-6,0.972500000001548,
2.57749999999708));
#21640=CARTESIAN_POINT('',(1.43126818176587E-6,0.949999999998922,2.554999999995));
#21641=CARTESIAN_POINT('Ctrl Pts',(1.63052496528509E-6,0.972500000001548,
2.57749999999709));
#21642=CARTESIAN_POINT('Ctrl Pts',(1.56410603744535E-6,0.965000000000673,
2.56999999999639));
#21643=CARTESIAN_POINT('Ctrl Pts',(1.49768710960561E-6,0.957499999999797,
2.5624999999957));
#21644=CARTESIAN_POINT('Ctrl Pts',(1.43126818176587E-6,0.949999999998922,
2.554999999995));
#21645=CARTESIAN_POINT('',(-3.4869210388678E-5,0.950019014087066,2.14494180214374));
#21646=CARTESIAN_POINT('Ctrl Pts',(1.43126818176587E-6,0.949999999998922,
2.554999999995));
#21647=CARTESIAN_POINT('Ctrl Pts',(-0.0256272820571188,0.950000038611092,
2.55500017892945));
#21648=CARTESIAN_POINT('Ctrl Pts',(-0.0770180954946874,0.947836654449066,
2.545491956117));
#21649=CARTESIAN_POINT('Ctrl Pts',(-0.122912016192401,0.942342690587028,
2.51623971854639));
#21650=CARTESIAN_POINT('Ctrl Pts',(-0.162273278240718,0.936710691441896,
2.47869732563017));
#21651=CARTESIAN_POINT('Ctrl Pts',(-0.190116748917708,0.931705920244711,
2.43873850533649));
#21652=CARTESIAN_POINT('Ctrl Pts',(-0.205180438332203,0.928732184994508,
2.37559643476243));
#21653=CARTESIAN_POINT('Ctrl Pts',(-0.2063281706048,0.928475438592001,2.31418526323498));
#21654=CARTESIAN_POINT('Ctrl Pts',(-0.184239643247193,0.932952809171462,
2.25049218467674));
#21655=CARTESIAN_POINT('Ctrl Pts',(-0.14553094537117,0.939236323471161,
2.20367459542476));
#21656=CARTESIAN_POINT('Ctrl Pts',(-0.100297800754953,0.945335204532955,
2.16670715064481));
#21657=CARTESIAN_POINT('Ctrl Pts',(-0.0465835707283805,0.949504783852479,
2.14738282011878));
#21658=CARTESIAN_POINT('Ctrl Pts',(-0.00936425895417839,0.950027004161095,
2.14491207293051));
#21659=CARTESIAN_POINT('Ctrl Pts',(-3.48692103886768E-5,0.950019014087066,
2.14494180214374));
#21660=CARTESIAN_POINT('Ctrl Pts',(-3.48692103886768E-5,0.950019014087066,
2.14494180214374));
#21661=CARTESIAN_POINT('Ctrl Pts',(0.00462828401910463,0.950015020370377,
2.14495666183772));
#21662=CARTESIAN_POINT('Ctrl Pts',(0.0163025714633961,0.949918483082405,
2.14539826893541));
#21663=CARTESIAN_POINT('Ctrl Pts',(0.0352153629354055,0.949440687181237,
2.14762723913071));
#21664=CARTESIAN_POINT('Ctrl Pts',(0.0780526805587212,0.947387432123376,
2.15736934465489));
#21665=CARTESIAN_POINT('Ctrl Pts',(0.118791192081503,0.942966542359005,
2.17967292326805));
#21666=CARTESIAN_POINT('Ctrl Pts',(0.160393955305448,0.936941762000965,
2.2197692915117));
#21667=CARTESIAN_POINT('Ctrl Pts',(0.178421760132616,0.933804534087895,
2.24615013735776));
#21668=CARTESIAN_POINT('Ctrl Pts',(0.199355148110418,0.929918951193924,
2.29392783383353));
#21669=CARTESIAN_POINT('Ctrl Pts',(0.205101073179634,0.928738263704097,
2.32281627503367));
#21670=CARTESIAN_POINT('Ctrl Pts',(0.205091310995403,0.928737319138035,
2.3769938343437));
#21671=CARTESIAN_POINT('Ctrl Pts',(0.193383491552286,0.931180374453942,
2.43471106618067));
#21672=CARTESIAN_POINT('Ctrl Pts',(0.156163794256122,0.937706308072193,
2.4861140371438));
#21673=CARTESIAN_POINT('Ctrl Pts',(0.127220061761462,0.941655887843543,
2.51114315400046));
#21674=CARTESIAN_POINT('Ctrl Pts',(0.105719704638418,0.944293922425639,
2.52657248312153));
#21675=CARTESIAN_POINT('Ctrl Pts',(0.0642457540090459,0.948373608976796,
2.54780176858962));
#21676=CARTESIAN_POINT('Ctrl Pts',(0.0257051198214169,0.949999961273794,
2.55499982053709));
#21677=CARTESIAN_POINT('Ctrl Pts',(1.43126818176587E-6,0.949999999998922,
2.554999999995));
#21678=CARTESIAN_POINT('Ctrl Pts',(1.63052496528509E-6,0.972500000001548,
2.57749999999708));
#21679=CARTESIAN_POINT('Ctrl Pts',(0.000580473862567526,0.972500001100936,
2.57749999792719));
#21680=CARTESIAN_POINT('Ctrl Pts',(0.00115932100720228,0.972500587629742,
2.5774988936244));
#21681=CARTESIAN_POINT('Ctrl Pts',(0.00414265020169645,0.972506627935274,
2.57748752117621));
#21682=CARTESIAN_POINT('Ctrl Pts',(0.00654688441943462,0.972521597304209,
2.57745933671442));
#21683=CARTESIAN_POINT('Ctrl Pts',(0.0128156465435042,0.972586968658231,
2.57733627628346));
#21684=CARTESIAN_POINT('Ctrl Pts',(0.0166786361769429,0.972653363288268,
2.57721129835072));
#21685=CARTESIAN_POINT('Ctrl Pts',(0.0281987946478794,0.972929256482295,
2.57669227394828));
#21686=CARTESIAN_POINT('Ctrl Pts',(0.0358422720486675,0.973215079278776,
2.57615478699383));
#21687=CARTESIAN_POINT('Ctrl Pts',(0.0623401377173534,0.974562717145952,
2.57362665221117));
#21688=CARTESIAN_POINT('Ctrl Pts',(0.0810078079633459,0.976141626745025,
2.57067014303824));
#21689=CARTESIAN_POINT('Ctrl Pts',(0.119336271682641,0.980686505593142,
2.56227318576719));
#21690=CARTESIAN_POINT('Ctrl Pts',(0.138835225480719,0.983740474395769,
2.55667793110024));
#21691=CARTESIAN_POINT('Ctrl Pts',(0.157876674355193,0.987458837468451,
2.55));
#21692=CARTESIAN_POINT('Origin',(4.31687996699442E-17,0.705,2.35));
#21693=CARTESIAN_POINT('',(-0.205,0.457138928554548,2.35));
#21694=CARTESIAN_POINT('',(-1.45611632917078E-17,0.501,2.145));
#21695=CARTESIAN_POINT('Ctrl Pts',(-0.205,0.457138928554548,2.35));
#21696=CARTESIAN_POINT('Ctrl Pts',(-0.205,0.457138928554548,2.37609072012547));
#21697=CARTESIAN_POINT('Ctrl Pts',(-0.199722778787908,0.459609069157102,
2.40367567964064));
#21698=CARTESIAN_POINT('Ctrl Pts',(-0.178715671123715,0.468177727272261,
2.45407202914948));
#21699=CARTESIAN_POINT('Ctrl Pts',(-0.162998335554875,0.474117890962222,
2.47691544473161));
#21700=CARTESIAN_POINT('Ctrl Pts',(-0.126935588134045,0.485018345626291,
2.51297819215244));
#21701=CARTESIAN_POINT('Ctrl Pts',(-0.104084611878653,0.490733376060334,
2.52871076670624));
#21702=CARTESIAN_POINT('Ctrl Pts',(-0.0536585253249438,0.498772107838147,
2.5497295887861));
#21703=CARTESIAN_POINT('Ctrl Pts',(-0.0260615896504234,0.501,2.555));
#21704=CARTESIAN_POINT('Ctrl Pts',(0.0260615896504235,0.501,2.555));
#21705=CARTESIAN_POINT('Ctrl Pts',(0.0536585253249439,0.498772107838147,
2.5497295887861));
#21706=CARTESIAN_POINT('Ctrl Pts',(0.104084611878653,0.490733376060334,
2.52871076670624));
#21707=CARTESIAN_POINT('Ctrl Pts',(0.126935588134046,0.485018345626291,
2.51297819215244));
#21708=CARTESIAN_POINT('Ctrl Pts',(0.162998335554875,0.474117890962221,
2.47691544473161));
#21709=CARTESIAN_POINT('Ctrl Pts',(0.178715671123715,0.468177727272261,
2.45407202914948));
#21710=CARTESIAN_POINT('Ctrl Pts',(0.199722778787908,0.459609069157102,
2.40367567964064));
#21711=CARTESIAN_POINT('Ctrl Pts',(0.205,0.457138928554548,2.37609072012547));
#21712=CARTESIAN_POINT('Ctrl Pts',(0.205,0.457138928554548,2.32390927987453));
#21713=CARTESIAN_POINT('Ctrl Pts',(0.199722778787908,0.459609069157102,
2.29632432035936));
#21714=CARTESIAN_POINT('Ctrl Pts',(0.178715671123715,0.468177727272261,
2.24592797085052));
#21715=CARTESIAN_POINT('Ctrl Pts',(0.162998335554875,0.474117890962221,
2.22308455526839));
#21716=CARTESIAN_POINT('Ctrl Pts',(0.126935588134045,0.485018345626291,
2.18702180784756));
#21717=CARTESIAN_POINT('Ctrl Pts',(0.104084611878653,0.490733376060334,
2.17128923329376));
#21718=CARTESIAN_POINT('Ctrl Pts',(0.0536585253249439,0.498772107838147,
2.1502704112139));
#21719=CARTESIAN_POINT('Ctrl Pts',(0.0260615896504234,0.501,2.145));
#21720=CARTESIAN_POINT('Ctrl Pts',(-3.46944695195361E-17,0.501,2.145));
#21721=CARTESIAN_POINT('Ctrl Pts',(-3.46944695195361E-17,0.501,2.145));
#21722=CARTESIAN_POINT('Ctrl Pts',(-0.0260615896504235,0.501,2.145));
#21723=CARTESIAN_POINT('Ctrl Pts',(-0.0536585253249439,0.498772107838147,
2.1502704112139));
#21724=CARTESIAN_POINT('Ctrl Pts',(-0.104084611878653,0.490733376060334,
2.17128923329376));
#21725=CARTESIAN_POINT('Ctrl Pts',(-0.126935588134045,0.485018345626291,
2.18702180784756));
#21726=CARTESIAN_POINT('Ctrl Pts',(-0.162998335554875,0.474117890962221,
2.22308455526839));
#21727=CARTESIAN_POINT('Ctrl Pts',(-0.178715671123715,0.468177727272261,
2.24592797085052));
#21728=CARTESIAN_POINT('Ctrl Pts',(-0.199722778787908,0.459609069157102,
2.29632432035936));
#21729=CARTESIAN_POINT('Ctrl Pts',(-0.205,0.457138928554548,2.32390927987453));
#21730=CARTESIAN_POINT('Ctrl Pts',(-0.205,0.457138928554548,2.35));
#21731=CARTESIAN_POINT('',(1.80635402874235E-17,0.705,2.145));
#21732=CARTESIAN_POINT('Origin',(0.,0.,2.575));
#21733=CARTESIAN_POINT('',(-0.95,-1.16341445918999E-16,2.6));
#21734=CARTESIAN_POINT('Origin',(0.,0.,2.6));
#21735=CARTESIAN_POINT('',(-0.975,-1.19403062916867E-16,2.575));
#21736=CARTESIAN_POINT('Ctrl Pts',(0.958722904333223,-0.492368803403902,
1.28318567027397));
#21737=CARTESIAN_POINT('Ctrl Pts',(1.17966054547972,-0.551909716442828,
1.53751096017971));
#21738=CARTESIAN_POINT('Ctrl Pts',(1.38346957888851,-0.474301142999537,
1.74607168007007));
#21739=CARTESIAN_POINT('Ctrl Pts',(1.57015000455958,-0.25954308307403,1.90886782994505));
#21740=CARTESIAN_POINT('Ctrl Pts',(0.977056147031499,-0.499517476440598,
1.26357731004417));
#21741=CARTESIAN_POINT('Ctrl Pts',(1.20215092434677,-0.559685710444569,
1.51399891879435));
#21742=CARTESIAN_POINT('Ctrl Pts',(1.40943351079342,-0.480379041610332,
1.71946418982835));
#21743=CARTESIAN_POINT('Ctrl Pts',(1.59908490462109,-0.261294297877456,
1.87976839865854));
#21744=CARTESIAN_POINT('Ctrl Pts',(1.00746303394202,-0.518620069692388,
1.22814769645102));
#21745=CARTESIAN_POINT('Ctrl Pts',(1.23972845750293,-0.581473014736936,
1.47151503544581));
#21746=CARTESIAN_POINT('Ctrl Pts',(1.45412237507391,-0.500093997069209,
1.67108761359797));
#21747=CARTESIAN_POINT('Ctrl Pts',(1.65065338225238,-0.274488870722725,
1.82686083829874));
#21748=CARTESIAN_POINT('Ctrl Pts',(1.04993028655864,-0.572066424422519,
1.16792151434878));
#21749=CARTESIAN_POINT('Ctrl Pts',(1.2934389287759,-0.644190775510559,1.39927831144435));
#21750=CARTESIAN_POINT('Ctrl Pts',(1.52163836885008,-0.563757672145161,
1.58904291706244));
#21751=CARTESIAN_POINT('Ctrl Pts',(1.73461532684231,-0.33063289130358,1.73712011416644));
#21752=CARTESIAN_POINT('Ctrl Pts',(1.07500617197391,-0.618955132624418,
1.12620659350916));
#21753=CARTESIAN_POINT('Ctrl Pts',(1.32576077930413,-0.699668038277416,
1.34934531900258));
#21754=CARTESIAN_POINT('Ctrl Pts',(1.5644313526713,-0.621802268592357,1.53232296148774));
#21755=CARTESIAN_POINT('Ctrl Pts',(1.79095608809519,-0.385229355344034,
1.67514376227794));
#21756=CARTESIAN_POINT('Ctrl Pts',(1.08812946536139,-0.649605006049397,
1.10192284729582));
#21757=CARTESIAN_POINT('Ctrl Pts',(1.34295142581462,-0.736085457637468,
1.32027771712106));
#21758=CARTESIAN_POINT('Ctrl Pts',(1.58796351671871,-0.660325994321481,
1.4993370241196));
#21759=CARTESIAN_POINT('Ctrl Pts',(1.82316573807368,-0.422326616101437,
1.63910076829143));
#21760=CARTESIAN_POINT('',(0.962275025729455,-0.493314642657339,1.28727233489076));
#21761=CARTESIAN_POINT('',(1.08521613661244,-0.642908916934723,1.10727038327973));
#21762=CARTESIAN_POINT('Ctrl Pts',(0.962275025729455,-0.493314642657339,
1.28727233489076));
#21763=CARTESIAN_POINT('Ctrl Pts',(0.992714976574291,-0.505155444616777,
1.25478273943474));
#21764=CARTESIAN_POINT('Ctrl Pts',(1.01347020049701,-0.522900410113937,
1.22829923781273));
#21765=CARTESIAN_POINT('Ctrl Pts',(1.05095536138695,-0.572202237706898,
1.17205963503468));
#21766=CARTESIAN_POINT('Ctrl Pts',(1.0691927306699,-0.603178396559865,1.14130666672664));
#21767=CARTESIAN_POINT('Ctrl Pts',(1.08521613661244,-0.642908916934723,
1.10727038327973));
#21768=CARTESIAN_POINT('',(1.5699559447672,-0.259766273896474,1.90869858745619));
#21769=CARTESIAN_POINT('Ctrl Pts',(0.962275025729455,-0.493314642657339,
1.28727233489076));
#21770=CARTESIAN_POINT('Ctrl Pts',(1.06019965524839,-0.519074140629025,
1.39987124007464));
#21771=CARTESIAN_POINT('Ctrl Pts',(1.15475382712427,-0.517846241724568,
1.50346488650363));
#21772=CARTESIAN_POINT('Ctrl Pts',(1.35913828497575,-0.454602843714802,
1.715480776583));
#21773=CARTESIAN_POINT('Ctrl Pts',(1.46714441944577,-0.377981286365637,
1.81902921434248));
#21774=CARTESIAN_POINT('Ctrl Pts',(1.5699559447672,-0.259766273896474,1.90869858745619));
#21775=CARTESIAN_POINT('',(1.81394816223928,-0.428377445609995,1.63615580822897));
#21776=CARTESIAN_POINT('Ctrl Pts',(1.81394816223928,-0.428377445609995,
1.63615580822897));
#21777=CARTESIAN_POINT('Ctrl Pts',(1.79068402602087,-0.396788109812435,
1.66605750085059));
#21778=CARTESIAN_POINT('Ctrl Pts',(1.76065343036505,-0.361451075078504,
1.70278841264342));
#21779=CARTESIAN_POINT('Ctrl Pts',(1.70449155357827,-0.313194031324451,
1.76702045133065));
#21780=CARTESIAN_POINT('Ctrl Pts',(1.67910176739992,-0.293827753703524,
1.79540516147607));
#21781=CARTESIAN_POINT('Ctrl Pts',(1.63136425547036,-0.270592580621385,
1.84635863460718));
#21782=CARTESIAN_POINT('Ctrl Pts',(1.60535049511978,-0.261679155446849,
1.87346655258888));
#21783=CARTESIAN_POINT('Ctrl Pts',(1.5699559447672,-0.259766273896474,1.90869858745619));
#21784=CARTESIAN_POINT('Ctrl Pts',(1.08521613661244,-0.642908916934723,
1.10727038327973));
#21785=CARTESIAN_POINT('Ctrl Pts',(1.16760035714813,-0.668710261798003,
1.18103565901042));
#21786=CARTESIAN_POINT('Ctrl Pts',(1.25518160519556,-0.681355585835302,
1.25302429310885));
#21787=CARTESIAN_POINT('Ctrl Pts',(1.44098614169382,-0.665371573463992,
1.39260788389872));
#21788=CARTESIAN_POINT('Ctrl Pts',(1.53389259595497,-0.635301149560131,
1.45574709063856));
#21789=CARTESIAN_POINT('Ctrl Pts',(1.69239761845937,-0.541698310562567,
1.55895701082587));
#21790=CARTESIAN_POINT('Ctrl Pts',(1.75616935678546,-0.489122861296313,
1.59904902099409));
#21791=CARTESIAN_POINT('Ctrl Pts',(1.81394816223928,-0.428377445609995,
1.63615580822897));
#21792=CARTESIAN_POINT('Ctrl Pts',(1.21487793679797,-0.362330138275323,
1.10149705943221));
#21793=CARTESIAN_POINT('Ctrl Pts',(1.48329895916361,-0.383459937582893,
1.31979778023781));
#21794=CARTESIAN_POINT('Ctrl Pts',(1.70227260218966,-0.249644960941914,
1.49880741124996));
#21795=CARTESIAN_POINT('Ctrl Pts',(1.87179886587611,0.0391147916476142,
1.63852595246867));
#21796=CARTESIAN_POINT('Ctrl Pts',(1.18333690797345,-0.373447482460584,
1.12583385309083));
#21797=CARTESIAN_POINT('Ctrl Pts',(1.44573672483852,-0.398305182537799,
1.34892944774501));
#21798=CARTESIAN_POINT('Ctrl Pts',(1.66212671668267,-0.270675994878902,
1.5318660237053));
#21799=CARTESIAN_POINT('Ctrl Pts',(1.83255854794259,0.00930365130125684,
1.67464838892921));
#21800=CARTESIAN_POINT('Ctrl Pts',(1.13169790455625,-0.386758017000778,
1.16764044916318));
#21801=CARTESIAN_POINT('Ctrl Pts',(1.38402127269754,-0.416680587119745,
1.39897336709085));
#21802=CARTESIAN_POINT('Ctrl Pts',(1.59542335194445,-0.298670375694656,
1.58871211231351));
#21803=CARTESIAN_POINT('Ctrl Pts',(1.76604232095017,-0.0327265383253196,
1.73676275687621));
#21804=CARTESIAN_POINT('Ctrl Pts',(1.06341115236232,-0.39167174183756,1.22801607619329));
#21805=CARTESIAN_POINT('Ctrl Pts',(1.30168216224369,-0.425665904909547,
1.47139032317727));
#21806=CARTESIAN_POINT('Ctrl Pts',(1.50457544636212,-0.318647566754319,
1.67096220367118));
#21807=CARTESIAN_POINT('Ctrl Pts',(1.67209124376879,-0.0706042875438403,
1.82672793765153));
#21808=CARTESIAN_POINT('Ctrl Pts',(1.0286884268729,-0.38218165487343,1.263527751515));
#21809=CARTESIAN_POINT('Ctrl Pts',(1.25929056133869,-0.415770412604396,
1.51397381108002));
#21810=CARTESIAN_POINT('Ctrl Pts',(1.45588630034146,-0.312692596804321,
1.71945276482244));
#21811=CARTESIAN_POINT('Ctrl Pts',(1.61878272768802,-0.0729619965738721,
1.87976043671971));
#21812=CARTESIAN_POINT('Ctrl Pts',(1.01098164381094,-0.373486051297297,
1.28318517919159));
#21813=CARTESIAN_POINT('Ctrl Pts',(1.23750736860246,-0.406026489679721,
1.53754499301511));
#21814=CARTESIAN_POINT('Ctrl Pts',(1.43052436008973,-0.304436793685253,
1.74612783237316));
#21815=CARTESIAN_POINT('Ctrl Pts',(1.59003261827274,-0.0687169633138944,
1.90893369726573));
#21816=CARTESIAN_POINT('',(1.20742290720348,-0.364905277844141,1.10727038327973));
#21817=CARTESIAN_POINT('',(1.01462217612883,-0.373997862975654,1.28727233489076));
#21818=CARTESIAN_POINT('Ctrl Pts',(1.20742290720348,-0.364905277844141,
1.10727038327973));
#21819=CARTESIAN_POINT('Ctrl Pts',(1.18311862080933,-0.373615945090665,
1.12801545944046));
#21820=CARTESIAN_POINT('Ctrl Pts',(1.15609247800026,-0.381365818655255,
1.15133239961427));
#21821=CARTESIAN_POINT('Ctrl Pts',(1.10715678825458,-0.389206856698246,
1.19509600545485));
#21822=CARTESIAN_POINT('Ctrl Pts',(1.08733497046196,-0.390682503085345,
1.2132474061745));
#21823=CARTESIAN_POINT('Ctrl Pts',(1.05408067239119,-0.388091095569738,
1.24538218411127));
#21824=CARTESIAN_POINT('Ctrl Pts',(1.03595219175474,-0.384447468688916,
1.26364457695044));
#21825=CARTESIAN_POINT('Ctrl Pts',(1.01462217612883,-0.373997862975654,
1.28727233489076));
#21826=CARTESIAN_POINT('',(1.86363850813291,0.0276890267571665,1.63615580822897));
#21827=CARTESIAN_POINT('Ctrl Pts',(1.86363850813291,0.0276890267571664,
1.63615580822897));
#21828=CARTESIAN_POINT('Ctrl Pts',(1.80655480211395,-0.0698239366990066,
1.58477934055781));
#21829=CARTESIAN_POINT('Ctrl Pts',(1.74187241700953,-0.148691945288574,
1.53343685544651));
#21830=CARTESIAN_POINT('Ctrl Pts',(1.59669345888589,-0.274785130849277,
1.42076782591239));
#21831=CARTESIAN_POINT('Ctrl Pts',(1.51444831269985,-0.320436333138584,
1.35830292226017));
#21832=CARTESIAN_POINT('Ctrl Pts',(1.35321270714141,-0.366271065016131,
1.23020598103184));
#21833=CARTESIAN_POINT('Ctrl Pts',(1.2795761902763,-0.371649422530894,1.1696137009149));
#21834=CARTESIAN_POINT('Ctrl Pts',(1.20742290720348,-0.364905277844141,
1.10727038327973));
#21835=CARTESIAN_POINT('',(1.58980227845634,-0.0690572297370891,1.90869858745619));
#21836=CARTESIAN_POINT('Ctrl Pts',(1.58980227845634,-0.0690572297370894,
1.90869858745619));
#21837=CARTESIAN_POINT('Ctrl Pts',(1.63853765425277,-0.0758898445998981,
1.85971261137246));
#21838=CARTESIAN_POINT('Ctrl Pts',(1.67950604280849,-0.0682369940313469,
1.81924683990323));
#21839=CARTESIAN_POINT('Ctrl Pts',(1.7703562129981,-0.0309159708914552,
1.7294679192124));
#21840=CARTESIAN_POINT('Ctrl Pts',(1.81575345115033,-0.00571744860871286,
1.68453186312949));
#21841=CARTESIAN_POINT('Ctrl Pts',(1.86363850813291,0.0276890267571661,
1.63615580822897));
#21842=CARTESIAN_POINT('Ctrl Pts',(1.01462217612883,-0.373997862975654,
1.28727233489076));
#21843=CARTESIAN_POINT('Ctrl Pts',(1.11493412912611,-0.387792676785359,
1.39987124007464));
#21844=CARTESIAN_POINT('Ctrl Pts',(1.20865423507634,-0.375201374409042,
1.50346488650363));
#21845=CARTESIAN_POINT('Ctrl Pts',(1.40394856048621,-0.287835131123856,
1.715480776583));
#21846=CARTESIAN_POINT('Ctrl Pts',(1.50195515531182,-0.198779555753985,
1.81902921434248));
#21847=CARTESIAN_POINT('Ctrl Pts',(1.58980227845634,-0.0690572297370891,
1.90869858745619));
#21848=CARTESIAN_POINT('Ctrl Pts',(1.01462217612883,-0.373997862975654,
1.28727233489076));
#21849=CARTESIAN_POINT('Ctrl Pts',(1.24016643693111,-0.405014516431692,
1.54044292999952));
#21850=CARTESIAN_POINT('Ctrl Pts',(1.43238606966553,-0.302637979515068,
1.74808806061869));
#21851=CARTESIAN_POINT('Ctrl Pts',(1.59128107433209,-0.0668682522257824,
1.91020772674828));
#21852=CARTESIAN_POINT('Ctrl Pts',(0.997173125995706,-0.413770122869549,
1.28727233489076));
#21853=CARTESIAN_POINT('Ctrl Pts',(1.22092814469495,-0.453754022216744,
1.54044292999952));
#21854=CARTESIAN_POINT('Ctrl Pts',(1.41678703930426,-0.359331486839601,
1.74808806061869));
#21855=CARTESIAN_POINT('Ctrl Pts',(1.58474980982363,-0.130502516738118,
1.91020772674828));
#21856=CARTESIAN_POINT('Ctrl Pts',(0.979724075862581,-0.453542382763444,
1.28727233489076));
#21857=CARTESIAN_POINT('Ctrl Pts',(1.2016898524588,-0.502493528001797,1.54044292999952));
#21858=CARTESIAN_POINT('Ctrl Pts',(1.40118800894299,-0.416024994164134,
1.74808806061869));
#21859=CARTESIAN_POINT('Ctrl Pts',(1.57821854531517,-0.194136781250453,
1.91020772674828));
#21860=CARTESIAN_POINT('Ctrl Pts',(0.962275025729455,-0.493314642657339,
1.28727233489076));
#21861=CARTESIAN_POINT('Ctrl Pts',(1.18245156022264,-0.55123303378685,1.54044292999952));
#21862=CARTESIAN_POINT('Ctrl Pts',(1.38558897858172,-0.472718501488667,
1.74808806061869));
#21863=CARTESIAN_POINT('Ctrl Pts',(1.5716872808067,-0.257771045762789,1.91020772674828));
#21864=CARTESIAN_POINT('Ctrl Pts',(1.01462217612883,-0.373997862975654,
1.28727233489076));
#21865=CARTESIAN_POINT('Ctrl Pts',(1.00648281422349,-0.394056488869181,
1.28797191329047));
#21866=CARTESIAN_POINT('Ctrl Pts',(0.998068152324092,-0.414003503730721,
1.28831907556383));
#21867=CARTESIAN_POINT('Ctrl Pts',(0.989370462098315,-0.433838594404394,
1.288319084765));
#21868=CARTESIAN_POINT('Ctrl Pts',(0.98061834720741,-0.453797800577661,
1.28831909402374));
#21869=CARTESIAN_POINT('Ctrl Pts',(0.97158845574471,-0.473623504353524,
1.28796761487395));
#21870=CARTESIAN_POINT('Ctrl Pts',(0.962275025729455,-0.493314642657339,
1.28727233489076));
#21871=CARTESIAN_POINT('Ctrl Pts',(1.5699559447672,-0.259766273896474,1.90869858745619));
#21872=CARTESIAN_POINT('Ctrl Pts',(1.57432246394088,-0.227349477989724,
1.90968240330487));
#21873=CARTESIAN_POINT('Ctrl Pts',(1.57814313696878,-0.194870259405019,
1.91020759224355));
#21874=CARTESIAN_POINT('Ctrl Pts',(1.58148345331813,-0.162326115709102,
1.91020766105751));
#21875=CARTESIAN_POINT('Ctrl Pts',(1.5846721664331,-0.131259016977809,1.91020772674828));
#21876=CARTESIAN_POINT('Ctrl Pts',(1.58741938775354,-0.100166338107427,
1.90972920064616));
#21877=CARTESIAN_POINT('Ctrl Pts',(1.58980227845634,-0.0690572297370893,
1.90869858745619));
#21878=CARTESIAN_POINT('Origin',(0.,0.,1.86807790411448));
#21879=CARTESIAN_POINT('',(-1.4,-1.71450551880629E-16,2.1));
#21880=CARTESIAN_POINT('Origin',(0.,0.,2.1));
#21881=CARTESIAN_POINT('',(-1.82153560297087,-2.51062254834063E-10,1.67846439702913));
#21882=CARTESIAN_POINT('',(-1.63192209588552,-1.99852817118404E-16,1.86807790411448));
#21883=CARTESIAN_POINT('',(-1.86363850813291,-0.0276890267571664,1.63615580822897));
#21884=CARTESIAN_POINT('Ctrl Pts',(-1.82153560297087,-5.02124314349928E-10,
1.67846439702913));
#21885=CARTESIAN_POINT('Ctrl Pts',(-1.835325320101,-0.00850724271337055,
1.66467467989666));
#21886=CARTESIAN_POINT('Ctrl Pts',(-1.84937147874757,-0.017735792998272,
1.65056912712851));
#21887=CARTESIAN_POINT('Ctrl Pts',(-1.86363850813291,-0.027689026757167,
1.63615580822897));
#21888=CARTESIAN_POINT('',(-1.85754313061971,-0.153129647965885,1.63615580822897));
#21889=CARTESIAN_POINT('Origin',(0.,0.,1.63615580822897));
#21890=CARTESIAN_POINT('',(-1.57338902476662,-0.238090659850088,1.90869858745619));
#21891=CARTESIAN_POINT('Ctrl Pts',(-1.85754313061971,-0.153129647965885,
1.63615580822897));
#21892=CARTESIAN_POINT('Ctrl Pts',(-1.8208638312973,-0.179418518304102,
1.67055126645182));
#21893=CARTESIAN_POINT('Ctrl Pts',(-1.77686224462366,-0.205674380666754,
1.71144473817108));
#21894=CARTESIAN_POINT('Ctrl Pts',(-1.68888826787379,-0.239335933327674,
1.79435460643495));
#21895=CARTESIAN_POINT('Ctrl Pts',(-1.6630238425637,-0.243149658729552,
1.81929762514764));
#21896=CARTESIAN_POINT('Ctrl Pts',(-1.63091267750169,-0.246644834768741,
1.85055034165243));
#21897=CARTESIAN_POINT('Ctrl Pts',(-1.60540976577649,-0.246614602123327,
1.87576293296796));
#21898=CARTESIAN_POINT('Ctrl Pts',(-1.57338902476662,-0.238090659850087,
1.90869858745619));
#21899=CARTESIAN_POINT('',(-1.53333167412,-0.425598593400271,1.90869858745619));
#21900=CARTESIAN_POINT('Ctrl Pts',(-1.57338902476662,-0.238090659850087,
1.90869858745619));
#21901=CARTESIAN_POINT('Ctrl Pts',(-1.56752449044192,-0.270270193465538,
1.90968240330487));
#21902=CARTESIAN_POINT('Ctrl Pts',(-1.56112153591504,-0.30234041884027,
1.91020759224355));
#21903=CARTESIAN_POINT('Ctrl Pts',(-1.55424167207615,-0.334323953288057,
1.91020766105751));
#21904=CARTESIAN_POINT('Ctrl Pts',(-1.54767405698886,-0.364855886521523,
1.91020772674828));
#21905=CARTESIAN_POINT('Ctrl Pts',(-1.54067865355577,-0.395275719445611,
1.90972920064616));
#21906=CARTESIAN_POINT('Ctrl Pts',(-1.53333167412,-0.425598593400271,1.90869858745619));
#21907=CARTESIAN_POINT('',(-1.76386916735272,-0.602229799711917,1.63615580822897));
#21908=CARTESIAN_POINT('Ctrl Pts',(-1.53333167412,-0.425598593400271,1.90869858745619));
#21909=CARTESIAN_POINT('Ctrl Pts',(-1.58179316495641,-0.434160449860449,
1.85971261136993));
#21910=CARTESIAN_POINT('Ctrl Pts',(-1.61839155697287,-0.454098671559182,
1.81924683990076));
#21911=CARTESIAN_POINT('Ctrl Pts',(-1.69326237295061,-0.517667320349936,
1.72946791919794));
#21912=CARTESIAN_POINT('Ctrl Pts',(-1.72865094049847,-0.55566105726035,
1.68453186311304));
#21913=CARTESIAN_POINT('Ctrl Pts',(-1.76386916735272,-0.602229799711918,
1.63615580822897));
#21914=CARTESIAN_POINT('',(-1.71930883511106,-0.71964734468187,1.63615580822897));
#21915=CARTESIAN_POINT('Origin',(0.,0.,1.63615580822897));
#21916=CARTESIAN_POINT('',(-1.42280782457595,-0.71264162093535,1.90869858745619));
#21917=CARTESIAN_POINT('Ctrl Pts',(-1.71930883511106,-0.71964734468187,
1.63615580822897));
#21918=CARTESIAN_POINT('Ctrl Pts',(-1.68192000782792,-0.731529338010255,
1.66605750085977));
#21919=CARTESIAN_POINT('Ctrl Pts',(-1.6368541577183,-0.742466058393773,
1.70278841265036));
#21920=CARTESIAN_POINT('Ctrl Pts',(-1.56305346633165,-0.748495703972133,
1.76702045133087));
#21921=CARTESIAN_POINT('Ctrl Pts',(-1.53112948545226,-0.749239609810652,
1.7954051614765));
#21922=CARTESIAN_POINT('Ctrl Pts',(-1.47885173495873,-0.739977854207805,
1.84635863460877));
#21923=CARTESIAN_POINT('Ctrl Pts',(-1.45256698088295,-0.73189846196087,
1.87346655259029));
#21924=CARTESIAN_POINT('Ctrl Pts',(-1.42280782457595,-0.71264162093535,
1.90869858745619));
#21925=CARTESIAN_POINT('',(-1.32676788217082,-0.878593860895847,1.90869858745619));
#21926=CARTESIAN_POINT('Ctrl Pts',(-1.42280782457595,-0.71264162093535,
1.90869858745619));
#21927=CARTESIAN_POINT('Ctrl Pts',(-1.40728629823317,-0.741433935301229,
1.90968240330487));
#21928=CARTESIAN_POINT('Ctrl Pts',(-1.39128648195262,-0.769955910359912,
1.91020759224355));
#21929=CARTESIAN_POINT('Ctrl Pts',(-1.37485988693288,-0.79824806436543,
1.91020766105751));
#21930=CARTESIAN_POINT('Ctrl Pts',(-1.3591788275673,-0.825256153747753,
1.91020772674828));
#21931=CARTESIAN_POINT('Ctrl Pts',(-1.34312555820857,-0.852025435531464,
1.90972920064616));
#21932=CARTESIAN_POINT('Ctrl Pts',(-1.32676788217082,-0.878593860895846,
1.90869858745619));
#21933=CARTESIAN_POINT('',(-1.4914400228729,-1.11782012388912,1.63615580822897));
#21934=CARTESIAN_POINT('Ctrl Pts',(-1.32676788217082,-0.878593860895847,
1.90869858745619));
#21935=CARTESIAN_POINT('Ctrl Pts',(-1.37021173966974,-0.901712094514641,
1.85971261137088));
#21936=CARTESIAN_POINT('Ctrl Pts',(-1.39885762954068,-0.931983995284014,
1.81924683990171));
#21937=CARTESIAN_POINT('Ctrl Pts',(-1.45042021416875,-1.01557772746493,
1.72946791920256));
#21938=CARTESIAN_POINT('Ctrl Pts',(-1.47233603155308,-1.06264758730959,
1.68453186311793));
#21939=CARTESIAN_POINT('Ctrl Pts',(-1.4914400228729,-1.11782012388912,1.63615580822897));
#21940=CARTESIAN_POINT('',(-1.4127766116927,-1.21572094522251,1.63615580822897));
#21941=CARTESIAN_POINT('Origin',(0.,0.,1.63615580822897));
#21942=CARTESIAN_POINT('',(-1.13295228123076,-1.11743425489732,1.90869858745619));
#21943=CARTESIAN_POINT('Ctrl Pts',(-1.4127766116927,-1.21572094522251,1.63615580822897));
#21944=CARTESIAN_POINT('Ctrl Pts',(-1.3735459860182,-1.2154676093739,1.66605750084812));
#21945=CARTESIAN_POINT('Ctrl Pts',(-1.32730618314253,-1.21194293501399,
1.70278841264146));
#21946=CARTESIAN_POINT('Ctrl Pts',(-1.25525429172787,-1.19487180089464,
1.76702045133136));
#21947=CARTESIAN_POINT('Ctrl Pts',(-1.2246629021408,-1.18571424477025,1.79540516147636));
#21948=CARTESIAN_POINT('Ctrl Pts',(-1.17780584675887,-1.16075107842331,
1.84635863460519));
#21949=CARTESIAN_POINT('Ctrl Pts',(-1.15530422962322,-1.14494468407762,
1.87346655258698));
#21950=CARTESIAN_POINT('Ctrl Pts',(-1.13295228123076,-1.11743425489732,
1.90869858745619));
#21951=CARTESIAN_POINT('',(-0.990330805779366,-1.24558623976355,1.90869858745619));
#21952=CARTESIAN_POINT('Ctrl Pts',(-1.13295228123076,-1.11743425489732,
1.90869858745619));
#21953=CARTESIAN_POINT('Ctrl Pts',(-1.10929311801315,-1.14002095767567,
1.90968240330488));
#21954=CARTESIAN_POINT('Ctrl Pts',(-1.08526261347374,-1.16220275277526,
1.91020759224355));
#21955=CARTESIAN_POINT('Ctrl Pts',(-1.0608972368445,-1.18403409318141,1.91020766105751));
#21956=CARTESIAN_POINT('Ctrl Pts',(-1.03763770454778,-1.20487459874735,
1.91020772674828));
#21957=CARTESIAN_POINT('Ctrl Pts',(-1.01409797511791,-1.22537296557718,
1.90972920064616));
#21958=CARTESIAN_POINT('Ctrl Pts',(-0.990330805779366,-1.24558623976355,
1.90869858745619));
#21959=CARTESIAN_POINT('',(-1.07301833748062,-1.52399042602929,1.63615580822897));
#21960=CARTESIAN_POINT('Ctrl Pts',(-0.990330805779367,-1.24558623976355,
1.90869858745619));
#21961=CARTESIAN_POINT('Ctrl Pts',(-1.02450444247791,-1.28099787675963,
1.85971261137182));
#21962=CARTESIAN_POINT('Ctrl Pts',(-1.04239377091547,-1.31864023203577,
1.81924683990262));
#21963=CARTESIAN_POINT('Ctrl Pts',(-1.06560081914983,-1.4140763106475,1.72946791922643));
#21964=CARTESIAN_POINT('Ctrl Pts',(-1.07189861347384,-1.465614767582,1.6845318631466));
#21965=CARTESIAN_POINT('Ctrl Pts',(-1.07301833748062,-1.52399042602929,
1.63615580822897));
#21966=CARTESIAN_POINT('',(-0.967951970128401,-1.59279130921887,1.63615580822897));
#21967=CARTESIAN_POINT('Origin',(0.,0.,1.63615580822897));
#21968=CARTESIAN_POINT('',(-0.732195474855993,-1.41284463836769,1.90869858745619));
#21969=CARTESIAN_POINT('Ctrl Pts',(-0.967951970128401,-1.59279130921887,
1.63615580822897));
#21970=CARTESIAN_POINT('Ctrl Pts',(-0.930719713024342,-1.58042744247569,
1.66605750084852));
#21971=CARTESIAN_POINT('Ctrl Pts',(-0.88783223146424,-1.56278639305271,
1.7027884126418));
#21972=CARTESIAN_POINT('Ctrl Pts',(-0.824582081179338,-1.52428552078414,
1.76702045133143));
#21973=CARTESIAN_POINT('Ctrl Pts',(-0.798317781239416,-1.50612290809472,
1.79540516147644));
#21974=CARTESIAN_POINT('Ctrl Pts',(-0.761468116016933,-1.46790189965195,
1.84635863460764));
#21975=CARTESIAN_POINT('Ctrl Pts',(-0.744952250886494,-1.44591574321431,
1.87346655258914));
#21976=CARTESIAN_POINT('Ctrl Pts',(-0.732195474855993,-1.41284463836769,
1.90869858745619));
#21977=CARTESIAN_POINT('',(-0.55695325007777,-1.49065195897357,1.90869858745619));
#21978=CARTESIAN_POINT('Ctrl Pts',(-0.732195474855993,-1.41284463836769,
1.90869858745619));
#21979=CARTESIAN_POINT('Ctrl Pts',(-0.702714598502394,-1.42701478571972,
1.90968240330488));
#21980=CARTESIAN_POINT('Ctrl Pts',(-0.673005678918811,-1.44068509220623,
1.91020759224355));
#21981=CARTESIAN_POINT('Ctrl Pts',(-0.643086573508102,-1.45391861530618,
1.91020766105751));
#21982=CARTESIAN_POINT('Ctrl Pts',(-0.614525373360046,-1.46655152316666,
1.91020772674828));
#21983=CARTESIAN_POINT('Ctrl Pts',(-0.585803416586614,-1.47877245207676,
1.90972920064616));
#21984=CARTESIAN_POINT('Ctrl Pts',(-0.556953250077771,-1.49065195897357,
1.90869858745619));
#21985=CARTESIAN_POINT('',(-0.549562141057369,-1.78098192700405,1.63615580822897));
#21986=CARTESIAN_POINT('Ctrl Pts',(-0.55695325007777,-1.49065195897357,
1.90869858745619));
#21987=CARTESIAN_POINT('Ctrl Pts',(-0.578511512315346,-1.53489066159152,
1.85971261137103));
#21988=CARTESIAN_POINT('Ctrl Pts',(-0.583893147208912,-1.57621877537089,
1.81924683990186));
#21989=CARTESIAN_POINT('Ctrl Pts',(-0.576472991487369,-1.67415525213672,
1.7294679192084));
#21990=CARTESIAN_POINT('Ctrl Pts',(-0.566536290754651,-1.72511736292283,
1.68453186312477));
#21991=CARTESIAN_POINT('Ctrl Pts',(-0.549562141057369,-1.78098192700405,
1.63615580822897));
#21992=CARTESIAN_POINT('',(-0.428377445609995,-1.81394816223928,1.63615580822897));
#21993=CARTESIAN_POINT('Origin',(0.,0.,1.63615580822897));
#21994=CARTESIAN_POINT('',(-0.259766273896474,-1.5699559447672,1.90869858745619));
#21995=CARTESIAN_POINT('Ctrl Pts',(-0.428377445609995,-1.81394816223928,
1.63615580822897));
#21996=CARTESIAN_POINT('Ctrl Pts',(-0.396788109819453,-1.79068402602605,
1.66605750084394));
#21997=CARTESIAN_POINT('Ctrl Pts',(-0.361451075082306,-1.76065343036948,
1.70278841263835));
#21998=CARTESIAN_POINT('Ctrl Pts',(-0.313194031324859,-1.70449155357874,
1.76702045133011));
#21999=CARTESIAN_POINT('Ctrl Pts',(-0.29382775370378,-1.67910176740044,
1.79540516147552));
#22000=CARTESIAN_POINT('Ctrl Pts',(-0.270592580621278,-1.63136425547015,
1.84635863460741));
#22001=CARTESIAN_POINT('Ctrl Pts',(-0.261679155446836,-1.60535049511953,
1.87346655258912));
#22002=CARTESIAN_POINT('Ctrl Pts',(-0.259766273896474,-1.5699559447672,
1.90869858745619));
#22003=CARTESIAN_POINT('',(-0.0690572297370887,-1.58980227845634,1.90869858745619));
#22004=CARTESIAN_POINT('Ctrl Pts',(-0.259766273896473,-1.5699559447672,
1.90869858745619));
#22005=CARTESIAN_POINT('Ctrl Pts',(-0.227349477989679,-1.57432246394089,
1.90968240330488));
#22006=CARTESIAN_POINT('Ctrl Pts',(-0.194870259404996,-1.57814313696878,
1.91020759224355));
#22007=CARTESIAN_POINT('Ctrl Pts',(-0.162326115709102,-1.58148345331813,
1.91020766105751));
#22008=CARTESIAN_POINT('Ctrl Pts',(-0.131259016977817,-1.5846721664331,
1.91020772674828));
#22009=CARTESIAN_POINT('Ctrl Pts',(-0.100166338107431,-1.58741938775353,
1.90972920064616));
#22010=CARTESIAN_POINT('Ctrl Pts',(-0.0690572297370894,-1.58980227845634,
1.90869858745619));
#22011=CARTESIAN_POINT('',(0.0276890267571667,-1.86363850813291,1.63615580822897));
#22012=CARTESIAN_POINT('Ctrl Pts',(-0.0690572297370892,-1.58980227845634,
1.90869858745619));
#22013=CARTESIAN_POINT('Ctrl Pts',(-0.0758898445996493,-1.63853765425097,
1.85971261137426));
#22014=CARTESIAN_POINT('Ctrl Pts',(-0.0682369940319697,-1.6795060428066,
1.81924683990509));
#22015=CARTESIAN_POINT('Ctrl Pts',(-0.0309159709011246,-1.77035621297488,
1.72946791923535));
#22016=CARTESIAN_POINT('Ctrl Pts',(-0.00571744862659264,-1.8157534511247,
1.68453186315538));
#22017=CARTESIAN_POINT('Ctrl Pts',(0.0276890267571667,-1.86363850813291,
1.63615580822897));
#22018=CARTESIAN_POINT('',(0.153129647965884,-1.85754313061971,1.63615580822897));
#22019=CARTESIAN_POINT('Origin',(0.,0.,1.63615580822897));
#22020=CARTESIAN_POINT('',(0.238090659850087,-1.57338902476662,1.90869858745619));
#22021=CARTESIAN_POINT('Ctrl Pts',(0.153129647965884,-1.85754313061971,
1.63615580822897));
#22022=CARTESIAN_POINT('Ctrl Pts',(0.17941851828628,-1.82086383132218,1.67055126642849));
#22023=CARTESIAN_POINT('Ctrl Pts',(0.205674380657903,-1.77686224464677,
1.7114447381493));
#22024=CARTESIAN_POINT('Ctrl Pts',(0.23933593332684,-1.68888826787598,1.79435460643288));
#22025=CARTESIAN_POINT('Ctrl Pts',(0.243149658729243,-1.66302384256654,
1.81929762514487));
#22026=CARTESIAN_POINT('Ctrl Pts',(0.246644834768774,-1.63091267750138,
1.85055034165273));
#22027=CARTESIAN_POINT('Ctrl Pts',(0.246614602123246,-1.60540976577619,
1.87576293296827));
#22028=CARTESIAN_POINT('Ctrl Pts',(0.238090659850087,-1.57338902476662,
1.90869858745619));
#22029=CARTESIAN_POINT('',(0.425598593400271,-1.53333167412,1.90869858745619));
#22030=CARTESIAN_POINT('Ctrl Pts',(0.238090659850087,-1.57338902476662,
1.90869858745619));
#22031=CARTESIAN_POINT('Ctrl Pts',(0.270270193465529,-1.56752449044192,
1.90968240330487));
#22032=CARTESIAN_POINT('Ctrl Pts',(0.302340418840266,-1.56112153591504,
1.91020759224355));
#22033=CARTESIAN_POINT('Ctrl Pts',(0.334323953288058,-1.55424167207615,
1.91020766105751));
#22034=CARTESIAN_POINT('Ctrl Pts',(0.364855886521546,-1.54767405698885,
1.91020772674828));
#22035=CARTESIAN_POINT('Ctrl Pts',(0.395275719445622,-1.54067865355577,
1.90972920064616));
#22036=CARTESIAN_POINT('Ctrl Pts',(0.425598593400271,-1.53333167412,1.90869858745619));
#22037=CARTESIAN_POINT('',(0.602229799711917,-1.76386916735272,1.63615580822897));
#22038=CARTESIAN_POINT('Ctrl Pts',(0.425598593400271,-1.53333167412,1.90869858745619));
#22039=CARTESIAN_POINT('Ctrl Pts',(0.434160449860198,-1.58179316495496,
1.8597126113714));
#22040=CARTESIAN_POINT('Ctrl Pts',(0.454098671558146,-1.61839155697167,
1.8192468399022));
#22041=CARTESIAN_POINT('Ctrl Pts',(0.517667320342287,-1.69326237294158,
1.72946791920875));
#22042=CARTESIAN_POINT('Ctrl Pts',(0.555661057248714,-1.72865094048965,
1.68453186312515));
#22043=CARTESIAN_POINT('Ctrl Pts',(0.602229799711917,-1.76386916735272,
1.63615580822897));
#22044=CARTESIAN_POINT('',(0.71964734468187,-1.71930883511106,1.63615580822897));
#22045=CARTESIAN_POINT('Origin',(0.,0.,1.63615580822897));
#22046=CARTESIAN_POINT('',(0.71264162093535,-1.42280782457595,1.90869858745619));
#22047=CARTESIAN_POINT('Ctrl Pts',(0.71964734468187,-1.71930883511106,1.63615580822897));
#22048=CARTESIAN_POINT('Ctrl Pts',(0.731529338009191,-1.68192000783126,
1.6660575008571));
#22049=CARTESIAN_POINT('Ctrl Pts',(0.742466058393583,-1.63685415772067,
1.70278841264829));
#22050=CARTESIAN_POINT('Ctrl Pts',(0.7484957039722,-1.56305346633081,1.76702045133161));
#22051=CARTESIAN_POINT('Ctrl Pts',(0.749239609810595,-1.53112948545192,
1.79540516147683));
#22052=CARTESIAN_POINT('Ctrl Pts',(0.739977854208178,-1.47885173496085,
1.84635863460671));
#22053=CARTESIAN_POINT('Ctrl Pts',(0.73189846196194,-1.4525669808846,1.87346655258834));
#22054=CARTESIAN_POINT('Ctrl Pts',(0.71264162093535,-1.42280782457595,1.90869858745619));
#22055=CARTESIAN_POINT('',(0.878593860895847,-1.32676788217082,1.90869858745619));
#22056=CARTESIAN_POINT('Ctrl Pts',(0.712641620935351,-1.42280782457595,
1.90869858745619));
#22057=CARTESIAN_POINT('Ctrl Pts',(0.741433935301239,-1.40728629823317,
1.90968240330488));
#22058=CARTESIAN_POINT('Ctrl Pts',(0.769955910359916,-1.39128648195261,
1.91020759224355));
#22059=CARTESIAN_POINT('Ctrl Pts',(0.798248064365429,-1.37485988693288,
1.91020766105751));
#22060=CARTESIAN_POINT('Ctrl Pts',(0.825256153747754,-1.3591788275673,1.91020772674828));
#22061=CARTESIAN_POINT('Ctrl Pts',(0.852025435531465,-1.34312555820857,
1.90972920064616));
#22062=CARTESIAN_POINT('Ctrl Pts',(0.878593860895846,-1.32676788217082,
1.90869858745619));
#22063=CARTESIAN_POINT('',(1.11782012388912,-1.4914400228729,1.63615580822897));
#22064=CARTESIAN_POINT('Ctrl Pts',(0.878593860895847,-1.32676788217082,
1.90869858745619));
#22065=CARTESIAN_POINT('Ctrl Pts',(0.901712094513363,-1.37021173966734,
1.85971261137359));
#22066=CARTESIAN_POINT('Ctrl Pts',(0.9319839952815,-1.39885762953914,1.8192468399044));
#22067=CARTESIAN_POINT('Ctrl Pts',(1.01557772744379,-1.45042021415571,1.72946791922527));
#22068=CARTESIAN_POINT('Ctrl Pts',(1.06264758728011,-1.47233603154289,1.68453186314377));
#22069=CARTESIAN_POINT('Ctrl Pts',(1.11782012388912,-1.4914400228729,1.63615580822897));
#22070=CARTESIAN_POINT('',(1.21572094522251,-1.4127766116927,1.63615580822897));
#22071=CARTESIAN_POINT('Origin',(0.,0.,1.63615580822897));
#22072=CARTESIAN_POINT('',(1.11743425489732,-1.13295228123076,1.90869858745619));
#22073=CARTESIAN_POINT('Ctrl Pts',(1.21572094522251,-1.4127766116927,1.63615580822897));
#22074=CARTESIAN_POINT('Ctrl Pts',(1.21546760937391,-1.37354598601756,1.6660575008486));
#22075=CARTESIAN_POINT('Ctrl Pts',(1.21194293501389,-1.3273061831421,1.70278841264184));
#22076=CARTESIAN_POINT('Ctrl Pts',(1.19487180089496,-1.25525429172921,1.76702045133017));
#22077=CARTESIAN_POINT('Ctrl Pts',(1.18571424477058,-1.22466290214144,1.79540516147567));
#22078=CARTESIAN_POINT('Ctrl Pts',(1.16075107842279,-1.17780584675786,1.84635863460628));
#22079=CARTESIAN_POINT('Ctrl Pts',(1.14494468407672,-1.15530422962249,1.87346655258813));
#22080=CARTESIAN_POINT('Ctrl Pts',(1.11743425489732,-1.13295228123076,1.90869858745619));
#22081=CARTESIAN_POINT('',(1.24558623976355,-0.990330805779367,1.90869858745619));
#22082=CARTESIAN_POINT('Ctrl Pts',(1.11743425489732,-1.13295228123076,1.90869858745619));
#22083=CARTESIAN_POINT('Ctrl Pts',(1.14002095767566,-1.10929311801316,1.90968240330487));
#22084=CARTESIAN_POINT('Ctrl Pts',(1.16220275277526,-1.08526261347375,1.91020759224355));
#22085=CARTESIAN_POINT('Ctrl Pts',(1.18403409318141,-1.0608972368445,1.91020766105751));
#22086=CARTESIAN_POINT('Ctrl Pts',(1.20487459874738,-1.03763770454774,1.91020772674828));
#22087=CARTESIAN_POINT('Ctrl Pts',(1.2253729655772,-1.01409797511789,1.90972920064616));
#22088=CARTESIAN_POINT('Ctrl Pts',(1.24558623976355,-0.990330805779366,
1.90869858745619));
#22089=CARTESIAN_POINT('',(1.52399042602929,-1.07301833748062,1.63615580822897));
#22090=CARTESIAN_POINT('Ctrl Pts',(1.24558623976355,-0.990330805779366,
1.90869858745619));
#22091=CARTESIAN_POINT('Ctrl Pts',(1.28099787676127,-1.02450444247951,1.85971261136954));
#22092=CARTESIAN_POINT('Ctrl Pts',(1.31864023203821,-1.04239377091596,1.81924683990037));
#22093=CARTESIAN_POINT('Ctrl Pts',(1.41407631065895,-1.06560081915269,1.72946791921561));
#22094=CARTESIAN_POINT('Ctrl Pts',(1.46561476759698,-1.07189861347413,1.68453186313418));
#22095=CARTESIAN_POINT('Ctrl Pts',(1.52399042602929,-1.07301833748062,1.63615580822897));
#22096=CARTESIAN_POINT('',(1.59279130921887,-0.967951970128402,1.63615580822897));
#22097=CARTESIAN_POINT('Origin',(0.,0.,1.63615580822897));
#22098=CARTESIAN_POINT('',(1.41284463836769,-0.732195474855993,1.90869858745619));
#22099=CARTESIAN_POINT('Ctrl Pts',(1.59279130921887,-0.967951970128402,
1.63615580822897));
#22100=CARTESIAN_POINT('Ctrl Pts',(1.58042744248116,-0.93071971304077,1.66605750083532));
#22101=CARTESIAN_POINT('Ctrl Pts',(1.56278639305871,-0.887832231474075,
1.7027884126318));
#22102=CARTESIAN_POINT('Ctrl Pts',(1.52428552078368,-0.824582081178599,
1.76702045133218));
#22103=CARTESIAN_POINT('Ctrl Pts',(1.50612290809471,-0.798317781239404,
1.79540516147646));
#22104=CARTESIAN_POINT('Ctrl Pts',(1.46790189965391,-0.761468116018828,
1.84635863460502));
#22105=CARTESIAN_POINT('Ctrl Pts',(1.44591574321668,-0.744952250887404,
1.87346655258662));
#22106=CARTESIAN_POINT('Ctrl Pts',(1.41284463836769,-0.732195474855994,
1.90869858745619));
#22107=CARTESIAN_POINT('',(1.49065195897357,-0.556953250077771,1.90869858745619));
#22108=CARTESIAN_POINT('Ctrl Pts',(1.41284463836769,-0.732195474855994,
1.90869858745619));
#22109=CARTESIAN_POINT('Ctrl Pts',(1.42701478571971,-0.702714598502428,
1.90968240330487));
#22110=CARTESIAN_POINT('Ctrl Pts',(1.44068509220622,-0.673005678918828,
1.91020759224355));
#22111=CARTESIAN_POINT('Ctrl Pts',(1.45391861530618,-0.643086573508103,
1.91020766105751));
#22112=CARTESIAN_POINT('Ctrl Pts',(1.46655152316666,-0.614525373360053,
1.91020772674828));
#22113=CARTESIAN_POINT('Ctrl Pts',(1.47877245207676,-0.585803416586618,
1.90972920064616));
#22114=CARTESIAN_POINT('Ctrl Pts',(1.49065195897357,-0.556953250077771,
1.90869858745619));
#22115=CARTESIAN_POINT('',(1.78098192700405,-0.54956214105737,1.63615580822897));
#22116=CARTESIAN_POINT('Ctrl Pts',(1.49065195897357,-0.556953250077771,
1.90869858745619));
#22117=CARTESIAN_POINT('Ctrl Pts',(1.53489066158786,-0.578511512313559,
1.85971261137509));
#22118=CARTESIAN_POINT('Ctrl Pts',(1.57621877536647,-0.583893147209275,
1.8192468399059));
#22119=CARTESIAN_POINT('Ctrl Pts',(1.67415525211499,-0.576472991488994,
1.72946791922834));
#22120=CARTESIAN_POINT('Ctrl Pts',(1.72511736289743,-0.56653629076237,1.68453186314677));
#22121=CARTESIAN_POINT('Ctrl Pts',(1.78098192700405,-0.549562141057369,
1.63615580822897));
#22122=CARTESIAN_POINT('Origin',(0.,0.,1.63615580822897));
#22123=CARTESIAN_POINT('',(1.85754313061971,0.153129647965885,1.63615580822897));
#22124=CARTESIAN_POINT('Origin',(0.,0.,1.63615580822897));
#22125=CARTESIAN_POINT('',(1.57338902476662,0.238090659850088,1.90869858745619));
#22126=CARTESIAN_POINT('Ctrl Pts',(1.85754313061971,0.153129647965885,1.63615580822897));
#22127=CARTESIAN_POINT('Ctrl Pts',(1.82091613387028,0.179381031885754,1.670502220505));
#22128=CARTESIAN_POINT('Ctrl Pts',(1.7769385116542,0.205636042642618,1.71137352645763));
#22129=CARTESIAN_POINT('Ctrl Pts',(1.68891823997117,0.239331856619953,1.79432582270636));
#22130=CARTESIAN_POINT('Ctrl Pts',(1.66303434064729,0.243146486728477,1.81928768858642));
#22131=CARTESIAN_POINT('Ctrl Pts',(1.6309352979637,0.246645694090263,1.85052786620714));
#22132=CARTESIAN_POINT('Ctrl Pts',(1.60542169144917,0.24661777674522,1.87575066654868));
#22133=CARTESIAN_POINT('Ctrl Pts',(1.57338902476662,0.238090659850087,1.90869858745619));
#22134=CARTESIAN_POINT('',(1.53333167412,0.425598593400271,1.90869858745619));
#22135=CARTESIAN_POINT('Ctrl Pts',(1.57338902476662,0.238090659850087,1.90869858745619));
#22136=CARTESIAN_POINT('Ctrl Pts',(1.56752449044192,0.270270193465537,1.90968240330487));
#22137=CARTESIAN_POINT('Ctrl Pts',(1.56112153591504,0.30234041884027,1.91020759224355));
#22138=CARTESIAN_POINT('Ctrl Pts',(1.55424167207615,0.334323953288058,1.91020766105751));
#22139=CARTESIAN_POINT('Ctrl Pts',(1.54767405698885,0.36485588652155,1.91020772674828));
#22140=CARTESIAN_POINT('Ctrl Pts',(1.54067865355577,0.395275719445624,1.90972920064616));
#22141=CARTESIAN_POINT('Ctrl Pts',(1.53333167412,0.425598593400271,1.90869858745619));
#22142=CARTESIAN_POINT('',(1.76386916735272,0.602229799711917,1.63615580822897));
#22143=CARTESIAN_POINT('Ctrl Pts',(1.53333167412,0.425598593400271,1.90869858745619));
#22144=CARTESIAN_POINT('Ctrl Pts',(1.58179316495472,0.434160449860156,1.85971261137164));
#22145=CARTESIAN_POINT('Ctrl Pts',(1.61839155697147,0.454098671557975,1.81924683990245));
#22146=CARTESIAN_POINT('Ctrl Pts',(1.69326237294042,0.517667320341299,1.72946791921015));
#22147=CARTESIAN_POINT('Ctrl Pts',(1.72865094048853,0.555661057247196,1.6845318631267));
#22148=CARTESIAN_POINT('Ctrl Pts',(1.76386916735272,0.602229799711918,1.63615580822897));
#22149=CARTESIAN_POINT('',(1.71930883511106,0.71964734468187,1.63615580822897));
#22150=CARTESIAN_POINT('Origin',(0.,0.,1.63615580822897));
#22151=CARTESIAN_POINT('',(1.42280782457595,0.712641620935351,1.90869858745619));
#22152=CARTESIAN_POINT('Ctrl Pts',(1.71930883511106,0.71964734468187,1.63615580822897));
#22153=CARTESIAN_POINT('Ctrl Pts',(1.68192000785468,0.731529338001752,1.66605750083837));
#22154=CARTESIAN_POINT('Ctrl Pts',(1.63685415773697,0.742466058392258,1.7027884126341));
#22155=CARTESIAN_POINT('Ctrl Pts',(1.56305346633102,0.748495703972178,1.76702045133142));
#22156=CARTESIAN_POINT('Ctrl Pts',(1.53112948545266,0.749239609810725,1.79540516147611));
#22157=CARTESIAN_POINT('Ctrl Pts',(1.47885173496202,0.739977854208386,1.84635863460557));
#22158=CARTESIAN_POINT('Ctrl Pts',(1.45256698088552,0.731898461962535,1.87346655258725));
#22159=CARTESIAN_POINT('Ctrl Pts',(1.42280782457595,0.71264162093535,1.90869858745619));
#22160=CARTESIAN_POINT('',(1.32676788217082,0.878593860895846,1.90869858745619));
#22161=CARTESIAN_POINT('Ctrl Pts',(1.42280782457595,0.71264162093535,1.90869858745619));
#22162=CARTESIAN_POINT('Ctrl Pts',(1.40728629823316,0.741433935301243,1.90968240330488));
#22163=CARTESIAN_POINT('Ctrl Pts',(1.39128648195261,0.769955910359918,1.91020759224355));
#22164=CARTESIAN_POINT('Ctrl Pts',(1.37485988693288,0.798248064365429,1.91020766105751));
#22165=CARTESIAN_POINT('Ctrl Pts',(1.35917882756731,0.825256153747737,1.91020772674828));
#22166=CARTESIAN_POINT('Ctrl Pts',(1.34312555820857,0.852025435531456,1.90972920064616));
#22167=CARTESIAN_POINT('Ctrl Pts',(1.32676788217082,0.878593860895846,1.90869858745619));
#22168=CARTESIAN_POINT('',(1.4914400228729,1.11782012388912,1.63615580822897));
#22169=CARTESIAN_POINT('Ctrl Pts',(1.32676788217082,0.878593860895847,1.90869858745619));
#22170=CARTESIAN_POINT('Ctrl Pts',(1.37021173966576,0.901712094512517,1.85971261137537));
#22171=CARTESIAN_POINT('Ctrl Pts',(1.39885762953817,0.93198399527982,1.81924683990615));
#22172=CARTESIAN_POINT('Ctrl Pts',(1.45042021415007,1.01557772743474,1.72946791923503));
#22173=CARTESIAN_POINT('Ctrl Pts',(1.4723360315385,1.06264758726748,1.68453186315486));
#22174=CARTESIAN_POINT('Ctrl Pts',(1.4914400228729,1.11782012388912,1.63615580822897));
#22175=CARTESIAN_POINT('',(1.4127766116927,1.21572094522251,1.63615580822897));
#22176=CARTESIAN_POINT('Origin',(0.,0.,1.63615580822897));
#22177=CARTESIAN_POINT('',(1.13295228123076,1.11743425489732,1.90869858745619));
#22178=CARTESIAN_POINT('Ctrl Pts',(1.4127766116927,1.21572094522251,1.63615580822897));
#22179=CARTESIAN_POINT('Ctrl Pts',(1.37354598600622,1.21546760937383,1.66605750085724));
#22180=CARTESIAN_POINT('Ctrl Pts',(1.3273061831347,1.21194293501213,1.70278841264844));
#22181=CARTESIAN_POINT('Ctrl Pts',(1.2552542917288,1.19487180089487,1.76702045133053));
#22182=CARTESIAN_POINT('Ctrl Pts',(1.22466290214095,1.18571424477033,1.79540516147619));
#22183=CARTESIAN_POINT('Ctrl Pts',(1.17780584675802,1.16075107842286,1.84635863460612));
#22184=CARTESIAN_POINT('Ctrl Pts',(1.15530422962257,1.14494468407682,1.873466552588));
#22185=CARTESIAN_POINT('Ctrl Pts',(1.13295228123076,1.11743425489733,1.90869858745619));
#22186=CARTESIAN_POINT('',(0.990330805779366,1.24558623976355,1.90869858745619));
#22187=CARTESIAN_POINT('Ctrl Pts',(1.13295228123076,1.11743425489732,1.90869858745619));
#22188=CARTESIAN_POINT('Ctrl Pts',(1.10929311801315,1.14002095767567,1.90968240330487));
#22189=CARTESIAN_POINT('Ctrl Pts',(1.08526261347374,1.16220275277526,1.91020759224355));
#22190=CARTESIAN_POINT('Ctrl Pts',(1.0608972368445,1.18403409318141,1.91020766105751));
#22191=CARTESIAN_POINT('Ctrl Pts',(1.03763770454776,1.20487459874736,1.91020772674828));
#22192=CARTESIAN_POINT('Ctrl Pts',(1.0140979751179,1.22537296557719,1.90972920064616));
#22193=CARTESIAN_POINT('Ctrl Pts',(0.990330805779366,1.24558623976355,1.90869858745619));
#22194=CARTESIAN_POINT('',(1.07301833748062,1.52399042602929,1.63615580822897));
#22195=CARTESIAN_POINT('Ctrl Pts',(0.990330805779366,1.24558623976356,1.90869858745619));
#22196=CARTESIAN_POINT('Ctrl Pts',(1.02450444247754,1.28099787675924,1.85971261137236));
#22197=CARTESIAN_POINT('Ctrl Pts',(1.04239377091547,1.31864023203516,1.81924683990311));
#22198=CARTESIAN_POINT('Ctrl Pts',(1.06560081915497,1.41407631066917,1.72946791920612));
#22199=CARTESIAN_POINT('Ctrl Pts',(1.07189861347441,1.46561476761072,1.68453186312278));
#22200=CARTESIAN_POINT('Ctrl Pts',(1.07301833748062,1.52399042602929,1.63615580822897));
#22201=CARTESIAN_POINT('',(0.967951970128401,1.59279130921887,1.63615580822897));
#22202=CARTESIAN_POINT('Origin',(0.,0.,1.63615580822897));
#22203=CARTESIAN_POINT('',(0.732195474855993,1.41284463836769,1.90869858745619));
#22204=CARTESIAN_POINT('Ctrl Pts',(0.967951970128401,1.59279130921887,1.63615580822897));
#22205=CARTESIAN_POINT('Ctrl Pts',(0.930719713031906,1.58042744247821,1.66605750084244));
#22206=CARTESIAN_POINT('Ctrl Pts',(0.887832231468784,1.56278639305548,1.70278841263718));
#22207=CARTESIAN_POINT('Ctrl Pts',(0.824582081181466,1.52428552078543,1.76702045132927));
#22208=CARTESIAN_POINT('Ctrl Pts',(0.798317781240507,1.50612290809584,1.79540516147495));
#22209=CARTESIAN_POINT('Ctrl Pts',(0.761468116016308,1.46790189965131,1.84635863460849));
#22210=CARTESIAN_POINT('Ctrl Pts',(0.744952250886103,1.44591574321331,1.87346655259021));
#22211=CARTESIAN_POINT('Ctrl Pts',(0.732195474855993,1.41284463836769,1.90869858745619));
#22212=CARTESIAN_POINT('',(0.55695325007777,1.49065195897357,1.90869858745619));
#22213=CARTESIAN_POINT('Ctrl Pts',(0.732195474855993,1.41284463836769,1.90869858745619));
#22214=CARTESIAN_POINT('Ctrl Pts',(0.702714598502391,1.42701478571972,1.90968240330487));
#22215=CARTESIAN_POINT('Ctrl Pts',(0.67300567891881,1.44068509220623,1.91020759224355));
#22216=CARTESIAN_POINT('Ctrl Pts',(0.643086573508102,1.45391861530618,1.91020766105751));
#22217=CARTESIAN_POINT('Ctrl Pts',(0.614525373360064,1.46655152316665,1.91020772674828));
#22218=CARTESIAN_POINT('Ctrl Pts',(0.585803416586623,1.47877245207676,1.90972920064616));
#22219=CARTESIAN_POINT('Ctrl Pts',(0.55695325007777,1.49065195897357,1.90869858745619));
#22220=CARTESIAN_POINT('',(0.549562141057369,1.78098192700405,1.63615580822897));
#22221=CARTESIAN_POINT('Ctrl Pts',(0.55695325007777,1.49065195897357,1.90869858745619));
#22222=CARTESIAN_POINT('Ctrl Pts',(0.578511512313229,1.53489066158716,1.85971261137586));
#22223=CARTESIAN_POINT('Ctrl Pts',(0.583893147209425,1.57621877536565,1.81924683990662));
#22224=CARTESIAN_POINT('Ctrl Pts',(0.57647299149051,1.67415525209398,1.72946791924761));
#22225=CARTESIAN_POINT('Ctrl Pts',(0.566536290770542,1.72511736287052,1.68453186317007));
#22226=CARTESIAN_POINT('Ctrl Pts',(0.549562141057369,1.78098192700405,1.63615580822897));
#22227=CARTESIAN_POINT('',(0.428377445609994,1.81394816223928,1.63615580822897));
#22228=CARTESIAN_POINT('Origin',(0.,0.,1.63615580822897));
#22229=CARTESIAN_POINT('',(0.259766273896474,1.5699559447672,1.90869858745619));
#22230=CARTESIAN_POINT('Ctrl Pts',(0.428377445609995,1.81394816223928,1.63615580822897));
#22231=CARTESIAN_POINT('Ctrl Pts',(0.396788109845208,1.79068402604501,1.66605750081957));
#22232=CARTESIAN_POINT('Ctrl Pts',(0.361451075096166,1.76065343038563,1.70278841261988));
#22233=CARTESIAN_POINT('Ctrl Pts',(0.313194031326,1.70449155358005,1.7670204513286));
#22234=CARTESIAN_POINT('Ctrl Pts',(0.29382775370454,1.67910176740199,1.79540516147386));
#22235=CARTESIAN_POINT('Ctrl Pts',(0.270592580620559,1.63136425546867,1.84635863460898));
#22236=CARTESIAN_POINT('Ctrl Pts',(0.261679155446751,1.60535049511798,1.87346655259067));
#22237=CARTESIAN_POINT('Ctrl Pts',(0.259766273896474,1.5699559447672,1.90869858745619));
#22238=CARTESIAN_POINT('',(0.0690572297370888,1.58980227845634,1.90869858745619));
#22239=CARTESIAN_POINT('Ctrl Pts',(0.259766273896474,1.5699559447672,1.90869858745619));
#22240=CARTESIAN_POINT('Ctrl Pts',(0.227349477989723,1.57432246394088,1.90968240330487));
#22241=CARTESIAN_POINT('Ctrl Pts',(0.194870259405019,1.57814313696878,1.91020759224355));
#22242=CARTESIAN_POINT('Ctrl Pts',(0.162326115709102,1.58148345331813,1.91020766105751));
#22243=CARTESIAN_POINT('Ctrl Pts',(0.131259016977809,1.5846721664331,1.91020772674828));
#22244=CARTESIAN_POINT('Ctrl Pts',(0.100166338107427,1.58741938775354,1.90972920064616));
#22245=CARTESIAN_POINT('Ctrl Pts',(0.0690572297370895,1.58980227845634,
1.90869858745619));
#22246=CARTESIAN_POINT('',(-0.0276890267571665,1.86363850813291,1.63615580822897));
#22247=CARTESIAN_POINT('Ctrl Pts',(0.0690572297370894,1.58980227845634,
1.90869858745619));
#22248=CARTESIAN_POINT('Ctrl Pts',(0.0758898445998494,1.63853765425239,
1.85971261137284));
#22249=CARTESIAN_POINT('Ctrl Pts',(0.0682369940313255,1.67950604280803,
1.81924683990368));
#22250=CARTESIAN_POINT('Ctrl Pts',(0.0309159708965805,1.77035621298606,
1.72946791922431));
#22251=CARTESIAN_POINT('Ctrl Pts',(0.00571744861764431,1.81575345113751,
1.68453186314245));
#22252=CARTESIAN_POINT('Ctrl Pts',(-0.0276890267571666,1.86363850813291,
1.63615580822897));
#22253=CARTESIAN_POINT('',(-0.153129647965885,1.85754313061971,1.63615580822897));
#22254=CARTESIAN_POINT('Origin',(0.,0.,1.63615580822897));
#22255=CARTESIAN_POINT('',(-0.238090659850087,1.57338902476662,1.90869858745619));
#22256=CARTESIAN_POINT('Ctrl Pts',(-0.153129647965885,1.85754313061971,
1.63615580822897));
#22257=CARTESIAN_POINT('Ctrl Pts',(-0.179418518274793,1.8208638313382,1.67055126641347));
#22258=CARTESIAN_POINT('Ctrl Pts',(-0.20567438065217,1.77686224466177,1.71144473813517));
#22259=CARTESIAN_POINT('Ctrl Pts',(-0.239335933326219,1.6888882678776,1.79435460643136));
#22260=CARTESIAN_POINT('Ctrl Pts',(-0.243149658729012,1.66302384256867,
1.8192976251428));
#22261=CARTESIAN_POINT('Ctrl Pts',(-0.246644834768781,1.63091267750131,
1.8505503416528));
#22262=CARTESIAN_POINT('Ctrl Pts',(-0.246614602123229,1.60540976577613,
1.87576293296834));
#22263=CARTESIAN_POINT('Ctrl Pts',(-0.238090659850087,1.57338902476663,
1.90869858745619));
#22264=CARTESIAN_POINT('',(-0.425598593400271,1.53333167412,1.90869858745619));
#22265=CARTESIAN_POINT('Ctrl Pts',(-0.238090659850087,1.57338902476662,
1.90869858745619));
#22266=CARTESIAN_POINT('Ctrl Pts',(-0.270270193465531,1.56752449044192,
1.90968240330487));
#22267=CARTESIAN_POINT('Ctrl Pts',(-0.302340418840268,1.56112153591504,
1.91020759224355));
#22268=CARTESIAN_POINT('Ctrl Pts',(-0.334323953288058,1.55424167207615,
1.91020766105751));
#22269=CARTESIAN_POINT('Ctrl Pts',(-0.364855886521545,1.54767405698885,
1.91020772674828));
#22270=CARTESIAN_POINT('Ctrl Pts',(-0.395275719445621,1.54067865355577,
1.90972920064616));
#22271=CARTESIAN_POINT('Ctrl Pts',(-0.425598593400271,1.53333167412,1.90869858745619));
#22272=CARTESIAN_POINT('',(-0.602229799711917,1.76386916735272,1.63615580822897));
#22273=CARTESIAN_POINT('Ctrl Pts',(-0.425598593400271,1.53333167412,1.90869858745619));
#22274=CARTESIAN_POINT('Ctrl Pts',(-0.434160449860446,1.58179316495636,
1.85971261136998));
#22275=CARTESIAN_POINT('Ctrl Pts',(-0.454098671559147,1.61839155697284,
1.8192468399008));
#22276=CARTESIAN_POINT('Ctrl Pts',(-0.517667320349084,1.6932623729496,1.72946791919914));
#22277=CARTESIAN_POINT('Ctrl Pts',(-0.555661057259041,1.72865094049748,
1.6845318631144));
#22278=CARTESIAN_POINT('Ctrl Pts',(-0.602229799711917,1.76386916735272,
1.63615580822897));
#22279=CARTESIAN_POINT('',(-0.71964734468187,1.71930883511106,1.63615580822897));
#22280=CARTESIAN_POINT('Origin',(0.,0.,1.63615580822897));
#22281=CARTESIAN_POINT('',(-0.712641620935351,1.42280782457595,1.90869858745619));
#22282=CARTESIAN_POINT('Ctrl Pts',(-0.71964734468187,1.71930883511106,1.63615580822897));
#22283=CARTESIAN_POINT('Ctrl Pts',(-0.731529338009184,1.6819200078313,1.66605750085707));
#22284=CARTESIAN_POINT('Ctrl Pts',(-0.742466058393576,1.63685415772068,
1.70278841264829));
#22285=CARTESIAN_POINT('Ctrl Pts',(-0.748495703972309,1.56305346632953,
1.76702045133272));
#22286=CARTESIAN_POINT('Ctrl Pts',(-0.749239609810482,1.53112948545126,
1.79540516147747));
#22287=CARTESIAN_POINT('Ctrl Pts',(-0.739977854208578,1.47885173496312,
1.8463586346045));
#22288=CARTESIAN_POINT('Ctrl Pts',(-0.731898461963124,1.45256698088643,
1.87346655258617));
#22289=CARTESIAN_POINT('Ctrl Pts',(-0.71264162093535,1.42280782457595,1.90869858745619));
#22290=CARTESIAN_POINT('',(-0.878593860895847,1.32676788217082,1.90869858745619));
#22291=CARTESIAN_POINT('Ctrl Pts',(-0.712641620935351,1.42280782457595,
1.90869858745619));
#22292=CARTESIAN_POINT('Ctrl Pts',(-0.741433935301275,1.40728629823315,
1.90968240330488));
#22293=CARTESIAN_POINT('Ctrl Pts',(-0.769955910359934,1.3912864819526,1.91020759224355));
#22294=CARTESIAN_POINT('Ctrl Pts',(-0.798248064365429,1.37485988693287,
1.91020766105751));
#22295=CARTESIAN_POINT('Ctrl Pts',(-0.82525615374773,1.35917882756732,1.91020772674828));
#22296=CARTESIAN_POINT('Ctrl Pts',(-0.852025435531453,1.34312555820858,
1.90972920064616));
#22297=CARTESIAN_POINT('Ctrl Pts',(-0.878593860895846,1.32676788217082,
1.90869858745619));
#22298=CARTESIAN_POINT('',(-1.11782012388912,1.4914400228729,1.63615580822897));
#22299=CARTESIAN_POINT('Ctrl Pts',(-0.878593860895847,1.32676788217082,
1.90869858745619));
#22300=CARTESIAN_POINT('Ctrl Pts',(-0.901712094513524,1.37021173966765,
1.85971261137323));
#22301=CARTESIAN_POINT('Ctrl Pts',(-0.931983995281799,1.39885762953939,
1.81924683990403));
#22302=CARTESIAN_POINT('Ctrl Pts',(-1.01557772743753,1.45042021415179,1.72946791923204));
#22303=CARTESIAN_POINT('Ctrl Pts',(-1.06264758727016,1.47233603153943,1.68453186315251));
#22304=CARTESIAN_POINT('Ctrl Pts',(-1.11782012388912,1.4914400228729,1.63615580822897));
#22305=CARTESIAN_POINT('',(-1.21572094522251,1.4127766116927,1.63615580822897));
#22306=CARTESIAN_POINT('Origin',(0.,0.,1.63615580822897));
#22307=CARTESIAN_POINT('',(-1.11743425489732,1.13295228123076,1.90869858745619));
#22308=CARTESIAN_POINT('Ctrl Pts',(-1.21572094522251,1.4127766116927,1.63615580822897));
#22309=CARTESIAN_POINT('Ctrl Pts',(-1.21546760937391,1.37354598601819,1.66605750084812));
#22310=CARTESIAN_POINT('Ctrl Pts',(-1.21194293501399,1.32730618314253,1.70278841264146));
#22311=CARTESIAN_POINT('Ctrl Pts',(-1.19487180089464,1.25525429172787,1.76702045133136));
#22312=CARTESIAN_POINT('Ctrl Pts',(-1.18571424477025,1.2246629021408,1.79540516147636));
#22313=CARTESIAN_POINT('Ctrl Pts',(-1.16075107842331,1.17780584675887,1.84635863460519));
#22314=CARTESIAN_POINT('Ctrl Pts',(-1.14494468407762,1.15530422962322,1.87346655258698));
#22315=CARTESIAN_POINT('Ctrl Pts',(-1.11743425489732,1.13295228123076,1.90869858745619));
#22316=CARTESIAN_POINT('',(-1.24558623976355,0.990330805779366,1.90869858745619));
#22317=CARTESIAN_POINT('Ctrl Pts',(-1.11743425489732,1.13295228123076,1.90869858745619));
#22318=CARTESIAN_POINT('Ctrl Pts',(-1.14002095767565,1.10929311801317,1.90968240330487));
#22319=CARTESIAN_POINT('Ctrl Pts',(-1.16220275277525,1.08526261347375,1.91020759224355));
#22320=CARTESIAN_POINT('Ctrl Pts',(-1.18403409318141,1.0608972368445,1.91020766105751));
#22321=CARTESIAN_POINT('Ctrl Pts',(-1.20487459874736,1.03763770454776,1.91020772674828));
#22322=CARTESIAN_POINT('Ctrl Pts',(-1.22537296557719,1.0140979751179,1.90972920064616));
#22323=CARTESIAN_POINT('Ctrl Pts',(-1.24558623976355,0.990330805779366,
1.90869858745619));
#22324=CARTESIAN_POINT('',(-1.52399042602929,1.07301833748062,1.63615580822897));
#22325=CARTESIAN_POINT('Ctrl Pts',(-1.24558623976355,0.990330805779367,
1.90869858745619));
#22326=CARTESIAN_POINT('Ctrl Pts',(-1.28099787675963,1.02450444247792,1.85971261137182));
#22327=CARTESIAN_POINT('Ctrl Pts',(-1.31864023203577,1.04239377091547,1.81924683990261));
#22328=CARTESIAN_POINT('Ctrl Pts',(-1.41407631064749,1.06560081914982,1.72946791922645));
#22329=CARTESIAN_POINT('Ctrl Pts',(-1.46561476758198,1.07189861347385,1.68453186314661));
#22330=CARTESIAN_POINT('Ctrl Pts',(-1.52399042602929,1.07301833748062,1.63615580822897));
#22331=CARTESIAN_POINT('',(-1.59279130921887,0.967951970128402,1.63615580822897));
#22332=CARTESIAN_POINT('Origin',(0.,0.,1.63615580822897));
#22333=CARTESIAN_POINT('',(-1.41284463836769,0.732195474855993,1.90869858745619));
#22334=CARTESIAN_POINT('Ctrl Pts',(-1.59279130921887,0.967951970128402,
1.63615580822897));
#22335=CARTESIAN_POINT('Ctrl Pts',(-1.58042744247569,0.930719713024315,
1.66605750084853));
#22336=CARTESIAN_POINT('Ctrl Pts',(-1.56278639305271,0.887832231464228,
1.70278841264181));
#22337=CARTESIAN_POINT('Ctrl Pts',(-1.52428552078413,0.824582081179332,
1.76702045133144));
#22338=CARTESIAN_POINT('Ctrl Pts',(-1.50612290809471,0.798317781239413,
1.79540516147645));
#22339=CARTESIAN_POINT('Ctrl Pts',(-1.46790189965197,0.761468116016952,
1.84635863460761));
#22340=CARTESIAN_POINT('Ctrl Pts',(-1.44591574321434,0.744952250886503,
1.87346655258912));
#22341=CARTESIAN_POINT('Ctrl Pts',(-1.41284463836769,0.732195474855993,
1.90869858745619));
#22342=CARTESIAN_POINT('',(-1.49065195897357,0.55695325007777,1.90869858745619));
#22343=CARTESIAN_POINT('Ctrl Pts',(-1.41284463836769,0.732195474855993,
1.90869858745619));
#22344=CARTESIAN_POINT('Ctrl Pts',(-1.42701478571972,0.70271459850241,1.90968240330487));
#22345=CARTESIAN_POINT('Ctrl Pts',(-1.44068509220623,0.673005678918819,
1.91020759224355));
#22346=CARTESIAN_POINT('Ctrl Pts',(-1.45391861530618,0.643086573508102,
1.91020766105751));
#22347=CARTESIAN_POINT('Ctrl Pts',(-1.46655152316666,0.614525373360044,
1.91020772674828));
#22348=CARTESIAN_POINT('Ctrl Pts',(-1.47877245207676,0.585803416586613,
1.90972920064616));
#22349=CARTESIAN_POINT('Ctrl Pts',(-1.49065195897357,0.55695325007777,1.90869858745619));
#22350=CARTESIAN_POINT('',(-1.78098192700405,0.549562141057368,1.63615580822897));
#22351=CARTESIAN_POINT('Ctrl Pts',(-1.49065195897357,0.55695325007777,1.90869858745619));
#22352=CARTESIAN_POINT('Ctrl Pts',(-1.53489066159152,0.578511512315346,
1.85971261137103));
#22353=CARTESIAN_POINT('Ctrl Pts',(-1.57621877537088,0.583893147208912,
1.81924683990186));
#22354=CARTESIAN_POINT('Ctrl Pts',(-1.67415525213672,0.576472991487369,
1.7294679192084));
#22355=CARTESIAN_POINT('Ctrl Pts',(-1.72511736292283,0.566536290754648,
1.68453186312477));
#22356=CARTESIAN_POINT('Ctrl Pts',(-1.78098192700405,0.549562141057369,
1.63615580822897));
#22357=CARTESIAN_POINT('',(-1.81394816223928,0.428377445609995,1.63615580822897));
#22358=CARTESIAN_POINT('Origin',(0.,0.,1.63615580822897));
#22359=CARTESIAN_POINT('',(-1.5699559447672,0.259766273896474,1.90869858745619));
#22360=CARTESIAN_POINT('Ctrl Pts',(-1.81394816223928,0.428377445609995,
1.63615580822897));
#22361=CARTESIAN_POINT('Ctrl Pts',(-1.79068402603114,0.396788109826372,
1.6660575008374));
#22362=CARTESIAN_POINT('Ctrl Pts',(-1.76065343037378,0.361451075086,1.70278841263343));
#22363=CARTESIAN_POINT('Ctrl Pts',(-1.70449155357908,0.313194031325156,
1.76702045132971));
#22364=CARTESIAN_POINT('Ctrl Pts',(-1.67910176740082,0.293827753703966,
1.79540516147511));
#22365=CARTESIAN_POINT('Ctrl Pts',(-1.6313642554699,0.270592580621158,1.84635863460767));
#22366=CARTESIAN_POINT('Ctrl Pts',(-1.60535049511926,0.261679155446819,
1.8734665525894));
#22367=CARTESIAN_POINT('Ctrl Pts',(-1.5699559447672,0.259766273896474,1.90869858745619));
#22368=CARTESIAN_POINT('',(-1.58980227845634,0.0690572297370887,1.90869858745619));
#22369=CARTESIAN_POINT('Ctrl Pts',(-1.5699559447672,0.259766273896474,1.90869858745619));
#22370=CARTESIAN_POINT('Ctrl Pts',(-1.57432246394088,0.227349477989734,
1.90968240330487));
#22371=CARTESIAN_POINT('Ctrl Pts',(-1.57814313696878,0.194870259405024,
1.91020759224355));
#22372=CARTESIAN_POINT('Ctrl Pts',(-1.58148345331813,0.162326115709102,
1.91020766105751));
#22373=CARTESIAN_POINT('Ctrl Pts',(-1.5846721664331,0.131259016977824,1.91020772674828));
#22374=CARTESIAN_POINT('Ctrl Pts',(-1.58741938775354,0.100166338107434,
1.90972920064616));
#22375=CARTESIAN_POINT('Ctrl Pts',(-1.58980227845634,0.0690572297370887,
1.90869858745619));
#22376=CARTESIAN_POINT('Ctrl Pts',(-1.58980227845634,0.0690572297370892,
1.90869858745619));
#22377=CARTESIAN_POINT('Ctrl Pts',(-1.63853765425085,0.0758898445996293,
1.85971261137438));
#22378=CARTESIAN_POINT('Ctrl Pts',(-1.67950604280655,0.0682369940321497,
1.81924683990515));
#22379=CARTESIAN_POINT('Ctrl Pts',(-1.75795323731548,0.0360110823424086,
1.7417246466111));
#22380=CARTESIAN_POINT('Ctrl Pts',(-1.78904228717242,0.0200459877611124,
1.71095771283311));
#22381=CARTESIAN_POINT('Ctrl Pts',(-1.82153560297087,-5.02124314349928E-10,
1.67846439702913));
#22382=CARTESIAN_POINT('Origin',(0.,0.,1.37171309575435));
#22383=CARTESIAN_POINT('',(1.23077165948193,-0.27609248605186,1.10727038327973));
#22384=CARTESIAN_POINT('Origin',(0.,0.,1.10727038327973));
#22385=CARTESIAN_POINT('Ctrl Pts',(1.23077165948193,-0.27609248605186,1.10727038327973));
#22386=CARTESIAN_POINT('Ctrl Pts',(1.31709676330276,-0.275172898999399,
1.1810356590104));
#22387=CARTESIAN_POINT('Ctrl Pts',(1.40429909999041,-0.260135222790519,
1.25302429310882));
#22388=CARTESIAN_POINT('Ctrl Pts',(1.57126422405226,-0.18954862836963,1.38870233571737));
#22389=CARTESIAN_POINT('Ctrl Pts',(1.64663281162092,-0.136344571823203,
1.44896010631748));
#22390=CARTESIAN_POINT('Ctrl Pts',(1.77081457368154,-0.00172234028007623,
1.55344588116294));
#22391=CARTESIAN_POINT('Ctrl Pts',(1.81885265993609,0.0722540415540171,
1.5964737415496));
#22392=CARTESIAN_POINT('Ctrl Pts',(1.85754313061971,0.153129647965885,1.63615580822897));
#22393=CARTESIAN_POINT('Origin',(0.,0.,1.37171309575435));
#22394=CARTESIAN_POINT('',(1.03556549162895,-0.720159740047642,1.10727038327973));
#22395=CARTESIAN_POINT('Ctrl Pts',(1.78098192700405,-0.54956214105737,1.63615580822897));
#22396=CARTESIAN_POINT('Ctrl Pts',(1.70079633666899,-0.620893161259095,
1.58735805514614));
#22397=CARTESIAN_POINT('Ctrl Pts',(1.61925404078172,-0.674133367258213,
1.53858095020842));
#22398=CARTESIAN_POINT('Ctrl Pts',(1.4446131950236,-0.751969574388251,1.42806953503214));
#22399=CARTESIAN_POINT('Ctrl Pts',(1.3500715267369,-0.772017157909611,1.36461306044572));
#22400=CARTESIAN_POINT('Ctrl Pts',(1.1777963531315,-0.767479006699501,1.23357020765532));
#22401=CARTESIAN_POINT('Ctrl Pts',(1.10397180136272,-0.749676646324455,
1.17136442658356));
#22402=CARTESIAN_POINT('Ctrl Pts',(1.03556549162895,-0.720159740047643,
1.10727038327973));
#22403=CARTESIAN_POINT('Origin',(0.,0.,1.10727038327973));
#22404=CARTESIAN_POINT('Ctrl Pts',(0.759649337735664,-0.764532229233201,
1.28318567027397));
#22405=CARTESIAN_POINT('Ctrl Pts',(0.951374367053297,-0.889432488376419,
1.53751096017972));
#22406=CARTESIAN_POINT('Ctrl Pts',(1.16919064445972,-0.87860280381325,1.74607168007008));
#22407=CARTESIAN_POINT('Ctrl Pts',(1.41309816995492,-0.732043175543693,
1.90886782994506));
#22408=CARTESIAN_POINT('Ctrl Pts',(0.771069504093749,-0.773880285955837,
1.26847940010162));
#22409=CARTESIAN_POINT('Ctrl Pts',(0.965585896981729,-0.900241293626995,
1.51987665322459));
#22410=CARTESIAN_POINT('Ctrl Pts',(1.18626243797172,-0.888897245689574,
1.72611612827485));
#22411=CARTESIAN_POINT('Ctrl Pts',(1.43333134754251,-0.739998335618526,
1.88704325648017));
#22412=CARTESIAN_POINT('Ctrl Pts',(0.79001938035927,-0.793756470105421,
1.24117952306876));
#22413=CARTESIAN_POINT('Ctrl Pts',(0.989358920654672,-0.923380672132911,
1.48716712955728));
#22414=CARTESIAN_POINT('Ctrl Pts',(1.21569285383182,-0.911936310735738,
1.68888851879238));
#22415=CARTESIAN_POINT('Ctrl Pts',(1.46902007592141,-0.759433295933255,
1.84634532147278));
#22416=CARTESIAN_POINT('Ctrl Pts',(0.818798433422952,-0.852549487780081,
1.18072779772815));
#22417=CARTESIAN_POINT('Ctrl Pts',(1.02677414338759,-0.993235093958052,
1.41461332256796));
#22418=CARTESIAN_POINT('Ctrl Pts',(1.26586652272339,-0.985480669746802,
1.60644767971085));
#22419=CARTESIAN_POINT('Ctrl Pts',(1.5362079120753,-0.829355339157881,1.75614145458408));
#22420=CARTESIAN_POINT('Ctrl Pts',(0.830120749534202,-0.909788127533567,
1.13430117558029));
#22421=CARTESIAN_POINT('Ctrl Pts',(1.04293872696085,-1.0618660701672,1.35902160674438));
#22422=CARTESIAN_POINT('Ctrl Pts',(1.29215273573924,-1.06009969793961,1.54332567193682));
#22423=CARTESIAN_POINT('Ctrl Pts',(1.57786820262107,-0.904732449133388,
1.68715809360678));
#22424=CARTESIAN_POINT('Ctrl Pts',(0.834133632104406,-0.954061570898026,
1.10192284729582));
#22425=CARTESIAN_POINT('Ctrl Pts',(1.04975978886663,-1.115053684233,1.32027771712106));
#22426=CARTESIAN_POINT('Ctrl Pts',(1.30619109614144,-1.11871505289201,1.4993370241196));
#22427=CARTESIAN_POINT('Ctrl Pts',(1.60342755392884,-0.965045676875053,
1.63910076829144));
#22428=CARTESIAN_POINT('',(0.762735325532963,-0.766529441696069,1.28727233489076));
#22429=CARTESIAN_POINT('',(0.833432097145889,-0.946792943618195,1.10727038327973));
#22430=CARTESIAN_POINT('Ctrl Pts',(0.762735325532963,-0.766529441696069,
1.28727233489076));
#22431=CARTESIAN_POINT('Ctrl Pts',(0.788026430107248,-0.787197175676817,
1.25478273943462));
#22432=CARTESIAN_POINT('Ctrl Pts',(0.802282325162875,-0.810487357658538,
1.2282992378126));
#22433=CARTESIAN_POINT('Ctrl Pts',(0.822697729112149,-0.868959733809562,
1.17205963503304));
#22434=CARTESIAN_POINT('Ctrl Pts',(0.830470338502318,-0.904055468577785,
1.14130666672511));
#22435=CARTESIAN_POINT('Ctrl Pts',(0.833432097145889,-0.946792943618195,
1.10727038327973));
#22436=CARTESIAN_POINT('Ctrl Pts',(0.762735325532963,-0.766529441696069,
1.28727233489076));
#22437=CARTESIAN_POINT('Ctrl Pts',(0.847907059902912,-0.821288554787752,
1.39987124007464));
#22438=CARTESIAN_POINT('Ctrl Pts',(0.938212862837218,-0.849339599532016,
1.50346488650363));
#22439=CARTESIAN_POINT('Ctrl Pts',(1.15213731807335,-0.852349824604396,
1.715480776583));
#22440=CARTESIAN_POINT('Ctrl Pts',(1.27853461941729,-0.812854124246773,
1.81902921434248));
#22441=CARTESIAN_POINT('Ctrl Pts',(1.41284463836769,-0.732195474855993,
1.90869858745619));
#22442=CARTESIAN_POINT('Ctrl Pts',(0.833432097145889,-0.946792943618196,
1.10727038327973));
#22443=CARTESIAN_POINT('Ctrl Pts',(0.90381109288579,-0.996789604993471,
1.18103565901043));
#22444=CARTESIAN_POINT('Ctrl Pts',(0.983198189519679,-1.03588011685504,
1.25302429310888));
#22445=CARTESIAN_POINT('Ctrl Pts',(1.16484813617462,-1.07809517714267,1.39260788389877));
#22446=CARTESIAN_POINT('Ctrl Pts',(1.26249969691991,-1.07820617779495,1.4557470906386));
#22447=CARTESIAN_POINT('Ctrl Pts',(1.4421717994102,-1.03816533347022,1.55895701082589));
#22448=CARTESIAN_POINT('Ctrl Pts',(1.51906903401083,-1.00786966075201,1.5990490209941));
#22449=CARTESIAN_POINT('Ctrl Pts',(1.59279130921887,-0.967951970128402,
1.63615580822897));
#22450=CARTESIAN_POINT('Ctrl Pts',(1.04334803864883,-0.720016914634041,
1.10157231096021));
#22451=CARTESIAN_POINT('Ctrl Pts',(1.29208090893696,-0.823064346331372,
1.31988785480615));
#22452=CARTESIAN_POINT('Ctrl Pts',(1.54167481933163,-0.763481187915707,
1.49890963328679));
#22453=CARTESIAN_POINT('Ctrl Pts',(1.79212976983284,-0.541267439387045,
1.63863764640213));
#22454=CARTESIAN_POINT('Ctrl Pts',(0.99879485818792,-0.721111068024911,
1.13400885567558));
#22455=CARTESIAN_POINT('Ctrl Pts',(1.23841384267289,-0.826338820212016,
1.35870212368824));
#22456=CARTESIAN_POINT('Ctrl Pts',(1.48217213030307,-0.773689391859137,
1.54297833728479));
#22457=CARTESIAN_POINT('Ctrl Pts',(1.73011692219034,-0.56288064822183,1.68678245041579));
#22458=CARTESIAN_POINT('Ctrl Pts',(0.940500318558189,-0.71640818004708,
1.18052127745051));
#22459=CARTESIAN_POINT('Ctrl Pts',(1.16780827731181,-0.823317656434312,
1.4143978468945));
#22460=CARTESIAN_POINT('Ctrl Pts',(1.40296795752834,-0.778775904082548,
1.6062187263882));
#22461=CARTESIAN_POINT('Ctrl Pts',(1.64608829985706,-0.582659795462711,
1.75589536238257));
#22462=CARTESIAN_POINT('Ctrl Pts',(0.878650346215,-0.694504973991427,1.24109742378385));
#22463=CARTESIAN_POINT('Ctrl Pts',(1.09199968627953,-0.79959476424298,1.487102189602));
#22464=CARTESIAN_POINT('Ctrl Pts',(1.3154268563443,-0.76136977052119,1.6888313052158));
#22465=CARTESIAN_POINT('Ctrl Pts',(1.54892786092601,-0.579822225320567,
1.84628707150865));
#22466=CARTESIAN_POINT('Ctrl Pts',(0.856697251076076,-0.677918579829935,
1.26844862066248));
#22467=CARTESIAN_POINT('Ctrl Pts',(1.06477366572489,-0.780508474608168,
1.51987386218775));
#22468=CARTESIAN_POINT('Ctrl Pts',(1.28264229878622,-0.743414485344372,
1.72613059618618));
#22469=CARTESIAN_POINT('Ctrl Pts',(1.51049094310987,-0.566387689879693,
1.88706341654736));
#22470=CARTESIAN_POINT('Ctrl Pts',(0.846087143187382,-0.667616851769879,
1.28318517919043));
#22471=CARTESIAN_POINT('Ctrl Pts',(1.05147036139455,-0.768564946360839,
1.53754499301447));
#22472=CARTESIAN_POINT('Ctrl Pts',(1.26643337142018,-0.731592934569706,
1.7461278323729));
#22473=CARTESIAN_POINT('Ctrl Pts',(1.49097617326428,-0.556700816396479,
1.90893369726572));
#22474=CARTESIAN_POINT('',(0.849391336665505,-0.669228599956957,1.28727233489076));
#22475=CARTESIAN_POINT('Ctrl Pts',(1.03556549162895,-0.720159740047643,
1.10727038327973));
#22476=CARTESIAN_POINT('Ctrl Pts',(1.00975899746849,-0.720933639361777,
1.12801545944037));
#22477=CARTESIAN_POINT('Ctrl Pts',(0.981660765603823,-0.71995266969545,
1.15133239961421));
#22478=CARTESIAN_POINT('Ctrl Pts',(0.932697144981226,-0.712287980257606,
1.19509600545636));
#22479=CARTESIAN_POINT('Ctrl Pts',(0.913389476194193,-0.707566124812362,
1.21324740617548));
#22480=CARTESIAN_POINT('Ctrl Pts',(0.882563548282486,-0.694825406569064,
1.24538218411054));
#22481=CARTESIAN_POINT('Ctrl Pts',(0.866448281269861,-0.685758102882515,
1.26364457694964));
#22482=CARTESIAN_POINT('Ctrl Pts',(0.849391336665505,-0.669228599956958,
1.28727233489076));
#22483=CARTESIAN_POINT('Ctrl Pts',(0.849391336665505,-0.669228599956957,
1.28727233489076));
#22484=CARTESIAN_POINT('Ctrl Pts',(0.940530841324424,-0.713346345736857,
1.39987124007464));
#22485=CARTESIAN_POINT('Ctrl Pts',(1.03355488521186,-0.73033241101646,1.50346488650363));
#22486=CARTESIAN_POINT('Ctrl Pts',(1.2462884798982,-0.707591441492497,1.715480776583));
#22487=CARTESIAN_POINT('Ctrl Pts',(1.36701797678012,-0.653180259586498,
1.81902921434248));
#22488=CARTESIAN_POINT('Ctrl Pts',(1.49065195897357,-0.556953250077771,
1.90869858745619));
#22489=CARTESIAN_POINT('Ctrl Pts',(0.849391336665504,-0.669228599956957,
1.28727233489076));
#22490=CARTESIAN_POINT('Ctrl Pts',(1.05431200258793,-0.768424199911631,
1.54044292999952));
#22491=CARTESIAN_POINT('Ctrl Pts',(1.26875982659235,-0.730457460528791,
1.74808806061869));
#22492=CARTESIAN_POINT('Ctrl Pts',(1.49273480867877,-0.555328381808438,
1.91020772674828));
#22493=CARTESIAN_POINT('Ctrl Pts',(0.820505999621324,-0.701662213869995,
1.28727233489076));
#22494=CARTESIAN_POINT('Ctrl Pts',(1.02095396380933,-0.808833265245786,
1.54044292999951));
#22495=CARTESIAN_POINT('Ctrl Pts',(1.23640500988538,-0.779555824624012,
1.74808806061869));
#22496=CARTESIAN_POINT('Ctrl Pts',(1.46685913784949,-0.613829892004672,
1.91020772674828));
#22497=CARTESIAN_POINT('Ctrl Pts',(0.791620662577143,-0.734095827783032,
1.28727233489076));
#22498=CARTESIAN_POINT('Ctrl Pts',(0.98759592503072,-0.849242330579942,
1.54044292999952));
#22499=CARTESIAN_POINT('Ctrl Pts',(1.20405019317841,-0.828654188719233,
1.74808806061869));
#22500=CARTESIAN_POINT('Ctrl Pts',(1.4409834670202,-0.672331402200905,1.91020772674828));
#22501=CARTESIAN_POINT('Ctrl Pts',(0.762735325532963,-0.766529441696069,
1.28727233489076));
#22502=CARTESIAN_POINT('Ctrl Pts',(0.954237886252114,-0.889651395914097,
1.54044292999952));
#22503=CARTESIAN_POINT('Ctrl Pts',(1.17169537647143,-0.877752552814454,
1.74808806061869));
#22504=CARTESIAN_POINT('Ctrl Pts',(1.41510779619092,-0.730832912397139,
1.91020772674828));
#22505=CARTESIAN_POINT('Ctrl Pts',(0.849391336665504,-0.669228599956957,
1.28727233489076));
#22506=CARTESIAN_POINT('Ctrl Pts',(0.835451887202027,-0.68579028566881,
1.28797191329047));
#22507=CARTESIAN_POINT('Ctrl Pts',(0.821285101590925,-0.702160750604678,
1.28831907556383));
#22508=CARTESIAN_POINT('Ctrl Pts',(0.806883726521851,-0.718337308749603,
1.288319084765));
#22509=CARTESIAN_POINT('Ctrl Pts',(0.792392236721716,-0.734615089602759,
1.28831909402374));
#22510=CARTESIAN_POINT('Ctrl Pts',(0.777677820212489,-0.750680064449599,
1.28796761487395));
#22511=CARTESIAN_POINT('Ctrl Pts',(0.762735325532963,-0.766529441696069,
1.28727233489076));
#22512=CARTESIAN_POINT('Origin',(0.,0.,1.37171309575435));
#22513=CARTESIAN_POINT('',(0.762339710524744,-1.00491994924733,1.10727038327973));
#22514=CARTESIAN_POINT('Ctrl Pts',(1.52399042602929,-1.07301833748062,1.63615580822897));
#22515=CARTESIAN_POINT('Ctrl Pts',(1.42568690035943,-1.11607945894006,1.58735805514599));
#22516=CARTESIAN_POINT('Ctrl Pts',(1.33168344006445,-1.1415159485948,1.53858095020827));
#22517=CARTESIAN_POINT('Ctrl Pts',(1.14153741491427,-1.16157559133822,1.42806953503213));
#22518=CARTESIAN_POINT('Ctrl Pts',(1.04542790122454,-1.15142699410503,1.36461306044571));
#22519=CARTESIAN_POINT('Ctrl Pts',(0.882986840618225,-1.09387499947176,
1.23357020765531));
#22520=CARTESIAN_POINT('Ctrl Pts',(0.818276751491844,-1.05413090753297,
1.17136442658356));
#22521=CARTESIAN_POINT('Ctrl Pts',(0.762339710524743,-1.00491994924733,
1.10727038327973));
#22522=CARTESIAN_POINT('Origin',(0.,0.,1.10727038327973));
#22523=CARTESIAN_POINT('Ctrl Pts',(0.486216001172379,-0.96185791365589,
1.28318567027397));
#22524=CARTESIAN_POINT('Ctrl Pts',(0.629961036964703,-1.13989141130718,
1.53751096017972));
#22525=CARTESIAN_POINT('Ctrl Pts',(0.840463183520967,-1.19690070060403,
1.74607168007008));
#22526=CARTESIAN_POINT('Ctrl Pts',(1.11772244084117,-1.13288578154644,1.90886782994505));
#22527=CARTESIAN_POINT('Ctrl Pts',(0.494188516412735,-0.974277469399886,
1.26847940010162));
#22528=CARTESIAN_POINT('Ctrl Pts',(0.640136900598344,-1.15456280023806,
1.51987665322458));
#22529=CARTESIAN_POINT('Ctrl Pts',(0.853518266498016,-1.2119667709518,1.72611612827485));
#22530=CARTESIAN_POINT('Ctrl Pts',(1.13450705657511,-1.14670398409855,1.88704325648017));
#22531=CARTESIAN_POINT('Ctrl Pts',(0.506068912121111,-0.999036317271854,
1.24117979784214));
#22532=CARTESIAN_POINT('Ctrl Pts',(0.655595999565546,-1.18391556488183,
1.48716740433065));
#22533=CARTESIAN_POINT('Ctrl Pts',(0.87438875535233,-1.24297220725901,1.68888889262423));
#22534=CARTESIAN_POINT('Ctrl Pts',(1.16244328394297,-1.17621563803994,1.84634569530464));
#22535=CARTESIAN_POINT('Ctrl Pts',(0.515271549474752,-1.06384465023928,
1.18072830092662));
#22536=CARTESIAN_POINT('Ctrl Pts',(0.669593960494796,-1.26191264154004,
1.41461382576642));
#22537=CARTESIAN_POINT('Ctrl Pts',(0.899380393905811,-1.32842099300983,
1.60644836271615));
#22538=CARTESIAN_POINT('Ctrl Pts',(1.2047357142776,-1.26347706358718,1.75614213758938));
#22539=CARTESIAN_POINT('Ctrl Pts',(0.508351755467876,-1.12178134612809,
1.13430117558029));
#22540=CARTESIAN_POINT('Ctrl Pts',(0.66375901094087,-1.3321804361879,1.35902160674437));
#22541=CARTESIAN_POINT('Ctrl Pts',(0.901321456978324,-1.4075118803195,1.54332567193682));
#22542=CARTESIAN_POINT('Ctrl Pts',(1.22106413381299,-1.34803978074575,1.68715809360678));
#22543=CARTESIAN_POINT('Ctrl Pts',(0.498486987186291,-1.16512794184932,
1.10192284729582));
#22544=CARTESIAN_POINT('Ctrl Pts',(0.653810349677836,-1.38487268717996,
1.32027771712106));
#22545=CARTESIAN_POINT('Ctrl Pts',(0.896559590305321,-1.46759648753937,
1.4993370241196));
#22546=CARTESIAN_POINT('Ctrl Pts',(1.22673470906875,-1.41329934292755,1.63910076829144));
#22547=CARTESIAN_POINT('',(0.488533777383804,-0.964710998256926,1.28727233489076));
#22548=CARTESIAN_POINT('',(0.500065917147829,-1.15799828028599,1.10727038327973));
#22549=CARTESIAN_POINT('Ctrl Pts',(0.488533777383804,-0.964710998256926,
1.28727233489076));
#22550=CARTESIAN_POINT('Ctrl Pts',(0.506200366158218,-0.992182562456351,
1.2547827394346));
#22551=CARTESIAN_POINT('Ctrl Pts',(0.512561466011952,-1.01873815563797,
1.22829923781264));
#22552=CARTESIAN_POINT('Ctrl Pts',(0.513908711038643,-1.08065739676305,
1.17205963503661));
#22553=CARTESIAN_POINT('Ctrl Pts',(0.510455723375345,-1.11643729240063,
1.14130666672845));
#22554=CARTESIAN_POINT('Ctrl Pts',(0.500065917147829,-1.15799828028599,
1.10727038327973));
#22555=CARTESIAN_POINT('Ctrl Pts',(0.488533777383804,-0.964710998256926,
1.28727233489076));
#22556=CARTESIAN_POINT('Ctrl Pts',(0.552615413818274,-1.04310952295002,
1.39987124007464));
#22557=CARTESIAN_POINT('Ctrl Pts',(0.629833086622262,-1.09769367964031,
1.50346488650363));
#22558=CARTESIAN_POINT('Ctrl Pts',(0.832357123065218,-1.16666286599128,
1.715480776583));
#22559=CARTESIAN_POINT('Ctrl Pts',(0.964772942765736,-1.16815913695893,
1.81902921434248));
#22560=CARTESIAN_POINT('Ctrl Pts',(1.11743425489732,-1.13295228123076,1.90869858745619));
#22561=CARTESIAN_POINT('Ctrl Pts',(0.500065917147829,-1.15799828028599,
1.10727038327973));
#22562=CARTESIAN_POINT('Ctrl Pts',(0.551550501629604,-1.22729623661062,
1.18103565901044));
#22563=CARTESIAN_POINT('Ctrl Pts',(0.614972484708978,-1.28900548463583,
1.25302429310889));
#22564=CARTESIAN_POINT('Ctrl Pts',(0.774686679112385,-1.38528731335186,
1.39260788389878));
#22565=CARTESIAN_POINT('Ctrl Pts',(0.867524531197646,-1.41556887304305,
1.4557470906386));
#22566=CARTESIAN_POINT('Ctrl Pts',(1.05077615643295,-1.43300950021464,1.55895701082589));
#22567=CARTESIAN_POINT('Ctrl Pts',(1.13327165021091,-1.42795915557246,1.5990490209941));
#22568=CARTESIAN_POINT('Ctrl Pts',(1.21572094522251,-1.4127766116927,1.63615580822897));
#22569=CARTESIAN_POINT('Ctrl Pts',(0.769785488061416,-1.0071890534957,1.1015723109602));
#22570=CARTESIAN_POINT('Ctrl Pts',(0.974501097544584,-1.18205566887762,
1.31988785480615));
#22571=CARTESIAN_POINT('Ctrl Pts',(1.23029122098202,-1.2025174778094,1.4989096332868));
#22572=CARTESIAN_POINT('Ctrl Pts',(1.53715585837372,-1.06857448029103,1.63863764640215));
#22573=CARTESIAN_POINT('Ctrl Pts',(0.727074783470156,-0.994461965292039,
1.13400885567557));
#22574=CARTESIAN_POINT('Ctrl Pts',(0.922448816386937,-1.16858584308541,
1.35870212368824));
#22575=CARTESIAN_POINT('Ctrl Pts',(1.17054629234374,-1.19383871456864,1.5429783372848));
#22576=CARTESIAN_POINT('Ctrl Pts',(1.47149928669635,-1.06996683960028,1.6867824504158));
#22577=CARTESIAN_POINT('Ctrl Pts',(0.673083751047337,-0.971974682567371,
1.18052322600158));
#22578=CARTESIAN_POINT('Ctrl Pts',(0.856229621362344,-1.14389365895071,
1.41439979544558));
#22579=CARTESIAN_POINT('Ctrl Pts',(1.09364268483531,-1.17420151395341,1.60622137130567));
#22580=CARTESIAN_POINT('Ctrl Pts',(1.38546708108518,-1.06281232835787,1.75589800730004));
#22581=CARTESIAN_POINT('Ctrl Pts',(0.621030952892817,-0.932030917609336,
1.24109849008298));
#22582=CARTESIAN_POINT('Ctrl Pts',(0.791463701885441,-1.09790581924279,
1.48710325590114));
#22583=CARTESIAN_POINT('Ctrl Pts',(1.01576709402368,-1.13059499103696,1.68883275601271));
#22584=CARTESIAN_POINT('Ctrl Pts',(1.29394102274665,-1.03008879377587,1.84628852230557));
#22585=CARTESIAN_POINT('Ctrl Pts',(0.605279141158067,-0.909472892481624,
1.26844862066248));
#22586=CARTESIAN_POINT('Ctrl Pts',(0.771469550259553,-1.0713408286716,1.51987386218776));
#22587=CARTESIAN_POINT('Ctrl Pts',(0.990137606500536,-1.10338745862407,
1.7261305961862));
#22588=CARTESIAN_POINT('Ctrl Pts',(1.26153883267191,-1.00543407447982,1.88706341654738));
#22589=CARTESIAN_POINT('Ctrl Pts',(0.598371737953918,-0.89639666323125,
1.28318517919043));
#22590=CARTESIAN_POINT('Ctrl Pts',(0.762508109189142,-1.055870911185,1.53754499301449));
#22591=CARTESIAN_POINT('Ctrl Pts',(0.978375060596146,-1.08713566171041,
1.74612783237293));
#22592=CARTESIAN_POINT('Ctrl Pts',(1.24597259217493,-0.990190914807476,
1.90893369726575));
#22593=CARTESIAN_POINT('',(0.601016155111926,-0.89895057878464,1.28727233489076));
#22594=CARTESIAN_POINT('Ctrl Pts',(0.762339710524743,-1.00491994924733,
1.10727038327973));
#22595=CARTESIAN_POINT('Ctrl Pts',(0.737557128050331,-0.997681325972066,
1.12801545944067));
#22596=CARTESIAN_POINT('Ctrl Pts',(0.711137257837026,-0.98806553722051,
1.15133239961449));
#22597=CARTESIAN_POINT('Ctrl Pts',(0.666938606675585,-0.965645393506861,
1.19509600545645));
#22598=CARTESIAN_POINT('Ctrl Pts',(0.650035056038514,-0.955188244339448,
1.21324740617592));
#22599=CARTESIAN_POINT('Ctrl Pts',(0.624654954884888,-0.933545365639724,
1.24538218411107));
#22600=CARTESIAN_POINT('Ctrl Pts',(0.612130376113162,-0.919941956007489,
1.26364457695018));
#22601=CARTESIAN_POINT('Ctrl Pts',(0.601016155111926,-0.89895057878464,
1.28727233489076));
#22602=CARTESIAN_POINT('Ctrl Pts',(0.601016155111926,-0.89895057878464,
1.28727233489076));
#22603=CARTESIAN_POINT('Ctrl Pts',(0.674061841710201,-0.969072704191387,
1.39987124007464));
#22604=CARTESIAN_POINT('Ctrl Pts',(0.757283981982513,-1.01397342270847,
1.50346488650363));
#22605=CARTESIAN_POINT('Ctrl Pts',(0.966632999495317,-1.05808377148838,
1.715480776583));
#22606=CARTESIAN_POINT('Ctrl Pts',(1.09826755410688,-1.04364312863621,1.81902921434248));
#22607=CARTESIAN_POINT('Ctrl Pts',(1.24558623976355,-0.990330805779366,
1.90869858745619));
#22608=CARTESIAN_POINT('Ctrl Pts',(0.601016155111926,-0.89895057878464,
1.28727233489076));
#22609=CARTESIAN_POINT('Ctrl Pts',(0.765254163607779,-1.056615168778,1.54044292999952));
#22610=CARTESIAN_POINT('Ctrl Pts',(0.980938531722803,-1.08677467590956,
1.74808806061869));
#22611=CARTESIAN_POINT('Ctrl Pts',(1.248069259457,-0.989429100179332,1.91020772674828));
#22612=CARTESIAN_POINT('Ctrl Pts',(0.563522029202552,-0.920870718608735,
1.28727233489076));
#22613=CARTESIAN_POINT('Ctrl Pts',(0.721041695541498,-1.08473827279984,
1.54044292999952));
#22614=CARTESIAN_POINT('Ctrl Pts',(0.934995043558668,-1.12347180680942,
1.74808806061869));
#22615=CARTESIAN_POINT('Ctrl Pts',(1.20538207325406,-1.03707132063747,1.91020772674828));
#22616=CARTESIAN_POINT('Ctrl Pts',(0.526027903293178,-0.942790858432831,
1.28727233489076));
#22617=CARTESIAN_POINT('Ctrl Pts',(0.676829227475217,-1.11286137682168,
1.54044292999952));
#22618=CARTESIAN_POINT('Ctrl Pts',(0.889051555394535,-1.16016893770927,
1.74808806061869));
#22619=CARTESIAN_POINT('Ctrl Pts',(1.16269488705113,-1.0847135410956,1.91020772674828));
#22620=CARTESIAN_POINT('Ctrl Pts',(0.488533777383804,-0.964710998256926,
1.28727233489076));
#22621=CARTESIAN_POINT('Ctrl Pts',(0.632616759408936,-1.14098448084351,
1.54044292999952));
#22622=CARTESIAN_POINT('Ctrl Pts',(0.843108067230401,-1.19686606860912,
1.74808806061869));
#22623=CARTESIAN_POINT('Ctrl Pts',(1.1200077008482,-1.13235576155374,1.91020772674828));
#22624=CARTESIAN_POINT('Ctrl Pts',(0.601016155111926,-0.89895057878464,
1.28727233489076));
#22625=CARTESIAN_POINT('Ctrl Pts',(0.582641108525679,-0.910394151125273,
1.28797191329046));
#22626=CARTESIAN_POINT('Ctrl Pts',(0.564108942884271,-0.92158561096782,
1.28831907556383));
#22627=CARTESIAN_POINT('Ctrl Pts',(0.545413589903933,-0.932520162364074,
1.288319084765));
#22628=CARTESIAN_POINT('Ctrl Pts',(0.526601253184352,-0.94352313529324,
1.28831909402374));
#22629=CARTESIAN_POINT('Ctrl Pts',(0.50764266123789,-0.954254829541782,
1.28796761487395));
#22630=CARTESIAN_POINT('Ctrl Pts',(0.488533777383804,-0.964710998256926,
1.28727233489076));
#22631=CARTESIAN_POINT('Origin',(0.,0.,1.37171309575435));
#22632=CARTESIAN_POINT('',(0.414490807021285,-1.19131159212569,1.10727038327973));
#22633=CARTESIAN_POINT('Ctrl Pts',(1.11782012388912,-1.4914400228729,1.63615580822897));
#22634=CARTESIAN_POINT('Ctrl Pts',(1.01102129689823,-1.50201612299692,1.587358055146));
#22635=CARTESIAN_POINT('Ctrl Pts',(0.913758385849818,-1.49715899547354,
1.53858095020828));
#22636=CARTESIAN_POINT('Ctrl Pts',(0.72671999907427,-1.45747849623495,1.42806953503211));
#22637=CARTESIAN_POINT('Ctrl Pts',(0.638450508815826,-1.41812713365383,
1.36461306044569));
#22638=CARTESIAN_POINT('Ctrl Pts',(0.501744424014166,-1.31319488582044,
1.2335702076553));
#22639=CARTESIAN_POINT('Ctrl Pts',(0.452483071915568,-1.25539949095026,
1.17136442658355));
#22640=CARTESIAN_POINT('Ctrl Pts',(0.414490807021284,-1.19131159212569,
1.10727038327973));
#22641=CARTESIAN_POINT('Origin',(0.,0.,1.10727038327973));
#22642=CARTESIAN_POINT('Ctrl Pts',(0.165188454748262,-1.06503024383179,
1.28318567027397));
#22643=CARTESIAN_POINT('Ctrl Pts',(0.246882731381369,-1.27876982080873,
1.53751096017971));
#22644=CARTESIAN_POINT('Ctrl Pts',(0.429465330327856,-1.39803761752215,
1.74607168007008));
#22645=CARTESIAN_POINT('Ctrl Pts',(0.712936251587724,-1.42283363397204,
1.90886782994505));
#22646=CARTESIAN_POINT('Ctrl Pts',(0.168932913531383,-1.07930558594879,
1.26847940010162));
#22647=CARTESIAN_POINT('Ctrl Pts',(0.252026844288349,-1.29586765564978,
1.51987665322458));
#22648=CARTESIAN_POINT('Ctrl Pts',(0.437225780288044,-1.41640054440424,
1.72611612827484));
#22649=CARTESIAN_POINT('Ctrl Pts',(0.724629310334678,-1.44116225705855,
1.88704325648017));
#22650=CARTESIAN_POINT('Ctrl Pts',(0.172580460092752,-1.10652474870095,
1.24117906537517));
#22651=CARTESIAN_POINT('Ctrl Pts',(0.257658341550682,-1.32856177300787,
1.48716667186368));
#22652=CARTESIAN_POINT('Ctrl Pts',(0.447493258920482,-1.45233913898616,
1.68888789608759));
#22653=CARTESIAN_POINT('Ctrl Pts',(0.742078309759795,-1.47786361346603,
1.846344698768));
#22654=CARTESIAN_POINT('Ctrl Pts',(0.161305070542798,-1.171005693206,1.18072695962337));
#22655=CARTESIAN_POINT('Ctrl Pts',(0.246868029800146,-1.40706779462018,
1.41461248446318));
#22656=CARTESIAN_POINT('Ctrl Pts',(0.444855864337698,-1.54132997390971,
1.60644654213682));
#22657=CARTESIAN_POINT('Ctrl Pts',(0.755334809435768,-1.57392460995617,
1.75614031701005));
#22658=CARTESIAN_POINT('Ctrl Pts',(0.136821749681419,-1.22396679065339,
1.13430117558029));
#22659=CARTESIAN_POINT('Ctrl Pts',(0.219605938249048,-1.47209169926767,
1.35902160674437));
#22660=CARTESIAN_POINT('Ctrl Pts',(0.422262554132511,-1.61714699314179,
1.54332567193682));
#22661=CARTESIAN_POINT('Ctrl Pts',(0.744733799933223,-1.65939158627327,
1.68715809360678));
#22662=CARTESIAN_POINT('Ctrl Pts',(0.114044962799315,-1.26214347192869,
1.10192284729582));
#22663=CARTESIAN_POINT('Ctrl Pts',(0.193861398098011,-1.51913070253035,
1.32027771712106));
#22664=CARTESIAN_POINT('Ctrl Pts',(0.399166585072141,-1.67281935264038,
1.4993370241196));
#22665=CARTESIAN_POINT('Ctrl Pts',(0.729960523721706,-1.72320942225876,
1.63910076829143));
#22666=CARTESIAN_POINT('',(0.166511139289342,-1.06845992077163,1.28727233489076));
#22667=CARTESIAN_POINT('',(0.117749801015222,-1.25585067703094,1.10727038327973));
#22668=CARTESIAN_POINT('Ctrl Pts',(0.166511139289342,-1.06845992077163,
1.28727233489076));
#22669=CARTESIAN_POINT('Ctrl Pts',(0.174823883464339,-1.10004620708051,
1.25478273943433));
#22670=CARTESIAN_POINT('Ctrl Pts',(0.17266751934213,-1.12726776497774,1.22829923781233));
#22671=CARTESIAN_POINT('Ctrl Pts',(0.154814727716273,-1.18657278434574,
1.17205963503338));
#22672=CARTESIAN_POINT('Ctrl Pts',(0.140474145488556,-1.21953445537463,
1.14130666672549));
#22673=CARTESIAN_POINT('Ctrl Pts',(0.117749801015222,-1.25585067703094,
1.10727038327973));
#22674=CARTESIAN_POINT('Ctrl Pts',(0.166511139289342,-1.06845992077163,
1.28727233489076));
#22675=CARTESIAN_POINT('Ctrl Pts',(0.203229920731113,-1.16282366323453,
1.39987124007464));
#22676=CARTESIAN_POINT('Ctrl Pts',(0.259800859583567,-1.23859785430383,
1.50346488650363));
#22677=CARTESIAN_POINT('Ctrl Pts',(0.431100013478375,-1.36677481743678,
1.715480776583));
#22678=CARTESIAN_POINT('Ctrl Pts',(0.556572568507924,-1.40911659430226,
1.81902921434248));
#22679=CARTESIAN_POINT('Ctrl Pts',(0.712641620935351,-1.42280782457595,
1.90869858745619));
#22680=CARTESIAN_POINT('Ctrl Pts',(0.117749801015222,-1.25585067703094,
1.10727038327973));
#22681=CARTESIAN_POINT('Ctrl Pts',(0.145300304395592,-1.33766656151261,
1.18103565901042));
#22682=CARTESIAN_POINT('Ctrl Pts',(0.18654898832969,-1.41595401455113,1.25302429310886));
#22683=CARTESIAN_POINT('Ctrl Pts',(0.308693492339104,-1.55687787546587,
1.39260788389873));
#22684=CARTESIAN_POINT('Ctrl Pts',(0.387630019962874,-1.61436582414938,
1.45574709063857));
#22685=CARTESIAN_POINT('Ctrl Pts',(0.556523222076021,-1.68758071271375,
1.55895701082587));
#22686=CARTESIAN_POINT('Ctrl Pts',(0.636541741320434,-1.70827005906903,
1.59904902099409));
#22687=CARTESIAN_POINT('Ctrl Pts',(0.71964734468187,-1.71930883511106,1.63615580822897));
#22688=CARTESIAN_POINT('Ctrl Pts',(0.420870970491666,-1.19577051030242,
1.1015723109602));
#22689=CARTESIAN_POINT('Ctrl Pts',(0.561530328976117,-1.425339146688,1.31988785480614));
#22690=CARTESIAN_POINT('Ctrl Pts',(0.798478145979644,-1.52384297854318,
1.49890963328679));
#22691=CARTESIAN_POINT('Ctrl Pts',(1.13171442150225,-1.49128200586798,1.63863764640213));
#22692=CARTESIAN_POINT('Ctrl Pts',(0.384183563118433,-1.17046799657245,
1.13400885567557));
#22693=CARTESIAN_POINT('Ctrl Pts',(0.516188072874178,-1.39644354162126,
1.35870212368824));
#22694=CARTESIAN_POINT('Ctrl Pts',(0.744339227614173,-1.49712678593272,
1.54297833728479));
#22695=CARTESIAN_POINT('Ctrl Pts',(1.06884104848206,-1.47231722182136,1.68678245041579));
#22696=CARTESIAN_POINT('Ctrl Pts',(0.339783831202729,-1.13239708355232,
1.18052334762519));
#22697=CARTESIAN_POINT('Ctrl Pts',(0.460840019240362,-1.3524969326934,1.41439991706918));
#22698=CARTESIAN_POINT('Ctrl Pts',(0.677267520477999,-1.45468613664231,
1.60622153639668));
#22699=CARTESIAN_POINT('Ctrl Pts',(0.989230165483925,-1.43892742365129,
1.75589817239104));
#22700=CARTESIAN_POINT('Ctrl Pts',(0.302622070510769,-1.07832314329337,
1.24109855662706));
#22701=CARTESIAN_POINT('Ctrl Pts',(0.413455083485284,-1.28874616521844,
1.48710332244522));
#22702=CARTESIAN_POINT('Ctrl Pts',(0.61667872836244,-1.38914899293201,1.68883284655014));
#22703=CARTESIAN_POINT('Ctrl Pts',(0.912295978931507,-1.37952239046626,
1.846288612843));
#22704=CARTESIAN_POINT('Ctrl Pts',(0.294612091675752,-1.05200166174697,
1.26844862066248));
#22705=CARTESIAN_POINT('Ctrl Pts',(0.402648620070371,-1.25730287795417,
1.51987386218775));
#22706=CARTESIAN_POINT('Ctrl Pts',(0.600711346596184,-1.35535317970116,
1.72613059618619));
#22707=CARTESIAN_POINT('Ctrl Pts',(0.889098511634057,-1.34606156659877,
1.88706341654736));
#22708=CARTESIAN_POINT('Ctrl Pts',(0.292083537908477,-1.03743092373275,
1.28318517919043));
#22709=CARTESIAN_POINT('Ctrl Pts',(0.3989062505499,-1.23982087453714,1.53754499301448));
#22710=CARTESIAN_POINT('Ctrl Pts',(0.594546582101045,-1.33626197576335,
1.74612783237291));
#22711=CARTESIAN_POINT('Ctrl Pts',(0.879004532561912,-1.32675422741137,
1.90893369726573));
#22712=CARTESIAN_POINT('',(0.293809324770207,-1.04067701160391,1.28727233489076));
#22713=CARTESIAN_POINT('Ctrl Pts',(0.414490807021284,-1.19131159212569,
1.10727038327973));
#22714=CARTESIAN_POINT('Ctrl Pts',(0.393158028076601,-1.17676901314185,
1.12801545944039));
#22715=CARTESIAN_POINT('Ctrl Pts',(0.371002680489087,-1.15945966570535,
1.15133239961415));
#22716=CARTESIAN_POINT('Ctrl Pts',(0.335895470715215,-1.12447870759369,
1.19509600545509));
#22717=CARTESIAN_POINT('Ctrl Pts',(0.323050675538403,-1.10930988332415,
1.21324740617454));
#22718=CARTESIAN_POINT('Ctrl Pts',(0.30560078227685,-1.08088339992903,1.24538218411075));
#22719=CARTESIAN_POINT('Ctrl Pts',(0.297892884779821,-1.06407548086656,
1.26364457694995));
#22720=CARTESIAN_POINT('Ctrl Pts',(0.293809324770207,-1.04067701160391,
1.28727233489076));
#22721=CARTESIAN_POINT('Ctrl Pts',(0.293809324770207,-1.04067701160391,
1.28727233489076));
#22722=CARTESIAN_POINT('Ctrl Pts',(0.341610972564374,-1.12993947443311,
1.39987124007464));
#22723=CARTESIAN_POINT('Ctrl Pts',(0.406884846288962,-1.19835965101752,
1.50346488650363));
#22724=CARTESIAN_POINT('Ctrl Pts',(0.592356746173702,-1.30500348982786,
1.715480776583));
#22725=CARTESIAN_POINT('Ctrl Pts',(0.722011051157661,-1.33194693676576,
1.81902921434248));
#22726=CARTESIAN_POINT('Ctrl Pts',(0.878593860895847,-1.32676788217082,
1.90869858745619));
#22727=CARTESIAN_POINT('Ctrl Pts',(0.293809324770207,-1.04067701160391,
1.28727233489076));
#22728=CARTESIAN_POINT('Ctrl Pts',(0.401287915254421,-1.24137728305361,
1.54044292999952));
#22729=CARTESIAN_POINT('Ctrl Pts',(0.59709613876759,-1.3367108140079,1.74808806061869));
#22730=CARTESIAN_POINT('Ctrl Pts',(0.881233995309716,-1.32667760446677,
1.91020772674828));
#22731=CARTESIAN_POINT('Ctrl Pts',(0.251376596276585,-1.04993798132648,
1.28727233489076));
#22732=CARTESIAN_POINT('Ctrl Pts',(0.350548842321171,-1.25446154039629,
1.54044292999952));
#22733=CARTESIAN_POINT('Ctrl Pts',(0.542061247874906,-1.35741454085596,
1.74808806061869));
#22734=CARTESIAN_POINT('Ctrl Pts',(0.825913812937791,-1.3587969827055,1.91020772674828));
#22735=CARTESIAN_POINT('Ctrl Pts',(0.208943867782964,-1.05919895104906,
1.28727233489076));
#22736=CARTESIAN_POINT('Ctrl Pts',(0.29980976938792,-1.26754579773896,1.54044292999952));
#22737=CARTESIAN_POINT('Ctrl Pts',(0.487026356982221,-1.37811826770402,
1.74808806061869));
#22738=CARTESIAN_POINT('Ctrl Pts',(0.770593630565866,-1.39091636094422,
1.91020772674828));
#22739=CARTESIAN_POINT('Ctrl Pts',(0.166511139289342,-1.06845992077163,
1.28727233489076));
#22740=CARTESIAN_POINT('Ctrl Pts',(0.24907069645467,-1.28063005508163,1.54044292999952));
#22741=CARTESIAN_POINT('Ctrl Pts',(0.431991466089537,-1.39882199455207,
1.74808806061869));
#22742=CARTESIAN_POINT('Ctrl Pts',(0.715273448193942,-1.42303573918295,
1.91020772674828));
#22743=CARTESIAN_POINT('Ctrl Pts',(0.293809324770207,-1.04067701160391,
1.28727233489076));
#22744=CARTESIAN_POINT('Ctrl Pts',(0.272797358647511,-1.04588229398058,
1.28797191329046));
#22745=CARTESIAN_POINT('Ctrl Pts',(0.25171387046998,-1.05079925066492,1.28831907556383));
#22746=CARTESIAN_POINT('Ctrl Pts',(0.230554570986284,-1.05542144523633,
1.288319084765));
#22747=CARTESIAN_POINT('Ctrl Pts',(0.209262869938635,-1.06007256258898,
1.28831909402374));
#22748=CARTESIAN_POINT('Ctrl Pts',(0.187915901626942,-1.06442048323406,
1.28796761487395));
#22749=CARTESIAN_POINT('Ctrl Pts',(0.166511139289342,-1.06845992077163,
1.28727233489076));
#22750=CARTESIAN_POINT('Origin',(0.,0.,1.37171309575435));
#22751=CARTESIAN_POINT('',(0.0260686553993157,-1.26108935601086,1.10727038327973));
#22752=CARTESIAN_POINT('Ctrl Pts',(0.602229799711917,-1.76386916735272,
1.63615580822897));
#22753=CARTESIAN_POINT('Ctrl Pts',(0.497389884697426,-1.74092498377324,
1.58735805514619));
#22754=CARTESIAN_POINT('Ctrl Pts',(0.406388294299505,-1.70624968855542,
1.53858095020849));
#22755=CARTESIAN_POINT('Ctrl Pts',(0.240766166369039,-1.61071325107048,
1.42806953503218));
#22756=CARTESIAN_POINT('Ctrl Pts',(0.168977132258039,-1.54601110868793,
1.36461306044575));
#22757=CARTESIAN_POINT('Ctrl Pts',(0.071387767328661,-1.40397010717828,
1.23357020765533));
#22758=CARTESIAN_POINT('Ctrl Pts',(0.0423971966252674,-1.33378082531077,
1.17136442658357));
#22759=CARTESIAN_POINT('Ctrl Pts',(0.0260686553993153,-1.26108935601086,
1.10727038327973));
#22760=CARTESIAN_POINT('Origin',(0.,0.,1.10727038327973));
#22761=CARTESIAN_POINT('Ctrl Pts',(-0.172008888562255,-1.06394999323939,
1.28318567027397));
#22762=CARTESIAN_POINT('Ctrl Pts',(-0.160362439116273,-1.2924681694826,
1.5375052164054));
#22763=CARTESIAN_POINT('Ctrl Pts',(-0.023577760251312,-1.46231719972917,
1.74606225962531));
#22764=CARTESIAN_POINT('Ctrl Pts',(0.238345148032627,-1.57349708397912,
1.90885679993368));
#22765=CARTESIAN_POINT('Ctrl Pts',(-0.173142620221682,-1.08359887191535,
1.26357344997188));
#22766=CARTESIAN_POINT('Ctrl Pts',(-0.160807978363557,-1.31626526877614,
1.51398865241804));
#22767=CARTESIAN_POINT('Ctrl Pts',(-0.0213345743744544,-1.48889372807638,
1.71944966391904));
#22768=CARTESIAN_POINT('Ctrl Pts',(0.245622116073242,-1.601562386112,1.87975180733571));
#22769=CARTESIAN_POINT('Ctrl Pts',(-0.181917271417173,-1.11842748291058,
1.2281366482377));
#22770=CARTESIAN_POINT('Ctrl Pts',(-0.169920645136297,-1.35874448434795,
1.47149643610478));
#22771=CARTESIAN_POINT('Ctrl Pts',(-0.0262779583676895,-1.53749711063698,
1.6710635087107));
#22772=CARTESIAN_POINT('Ctrl Pts',(0.249006836337355,-1.6546951488403,1.82683387344445));
#22773=CARTESIAN_POINT('Ctrl Pts',(-0.219636735943001,-1.1753425954218,
1.16789882161102));
#22774=CARTESIAN_POINT('Ctrl Pts',(-0.21298531416801,-1.42921995625554,
1.39924604542984));
#22775=CARTESIAN_POINT('Ctrl Pts',(-0.0659764462771748,-1.62139761687088,
1.58900346231478));
#22776=CARTESIAN_POINT('Ctrl Pts',(0.221543302854981,-1.75191643683035,
1.73707641259309));
#22777=CARTESIAN_POINT('Ctrl Pts',(-0.256493105922012,-1.21368608666858,
1.126177305135));
#22778=CARTESIAN_POINT('Ctrl Pts',(-0.255772600666387,-1.47711033277873,
1.34930521631815));
#22779=CARTESIAN_POINT('Ctrl Pts',(-0.107970878520535,-1.6800421801244,
1.53227487652584));
#22780=CARTESIAN_POINT('Ctrl Pts',(0.187015176303949,-1.82238303426191,
1.67509057207931));
#22781=CARTESIAN_POINT('Ctrl Pts',(-0.281595159362693,-1.235641855012,1.10188938448118));
#22782=CARTESIAN_POINT('Ctrl Pts',(-0.285104353628414,-1.50471757474417,
1.32023273220193));
#22783=CARTESIAN_POINT('Ctrl Pts',(-0.137346783688564,-1.71433282083683,
1.49928348142626));
#22784=CARTESIAN_POINT('Ctrl Pts',(0.161677550456857,-1.86448759328998,
1.63904163215416));
#22785=CARTESIAN_POINT('',(-0.171810769270086,-1.06762054184321,1.28727233489076));
#22786=CARTESIAN_POINT('',(-0.27609248605186,-1.23077165948193,1.10727038327973));
#22787=CARTESIAN_POINT('Ctrl Pts',(-0.171810769270086,-1.06762054184321,
1.28727233489076));
#22788=CARTESIAN_POINT('Ctrl Pts',(-0.173665579012837,-1.10022966448349,
1.25478273943364));
#22789=CARTESIAN_POINT('Ctrl Pts',(-0.184128327166747,-1.12545255134542,
1.22829923781169));
#22790=CARTESIAN_POINT('Ctrl Pts',(-0.219433599813331,-1.1763381604554,
1.17205963503223));
#22791=CARTESIAN_POINT('Ctrl Pts',(-0.24325802049969,-1.20325508885762,
1.14130666672443));
#22792=CARTESIAN_POINT('Ctrl Pts',(-0.27609248605186,-1.23077165948193,
1.10727038327973));
#22793=CARTESIAN_POINT('Ctrl Pts',(-0.171810769270086,-1.06762054184321,
1.28727233489076));
#22794=CARTESIAN_POINT('Ctrl Pts',(-0.166049132983329,-1.16871252149279,
1.39987124007464));
#22795=CARTESIAN_POINT('Ctrl Pts',(-0.135662485730196,-1.2582594411694,
1.50346488650363));
#22796=CARTESIAN_POINT('Ctrl Pts',(-0.0123561690781442,-1.43309732687145,
1.715480776583));
#22797=CARTESIAN_POINT('Ctrl Pts',(0.0938909933754464,-1.51213990150266,
1.81902921434248));
#22798=CARTESIAN_POINT('Ctrl Pts',(0.238090659850087,-1.57338902476662,
1.90869858745619));
#22799=CARTESIAN_POINT('Ctrl Pts',(-0.27609248605186,-1.23077165948193,
1.10727038327973));
#22800=CARTESIAN_POINT('Ctrl Pts',(-0.275172898999399,-1.31709676330278,
1.18103565901041));
#22801=CARTESIAN_POINT('Ctrl Pts',(-0.260135222790515,-1.40429909999044,
1.25302429310884));
#22802=CARTESIAN_POINT('Ctrl Pts',(-0.189563202796486,-1.57122974978687,
1.38867432147861));
#22803=CARTESIAN_POINT('Ctrl Pts',(-0.136388204217752,-1.64657149028472,
1.44891114041811));
#22804=CARTESIAN_POINT('Ctrl Pts',(-0.00179051121356718,-1.77077010917836,
1.55340617058598));
#22805=CARTESIAN_POINT('Ctrl Pts',(0.0722162251277554,-1.81883456875388,
1.59645518670945));
#22806=CARTESIAN_POINT('Ctrl Pts',(0.153129647965885,-1.85754313061971,
1.63615580822897));
#22807=CARTESIAN_POINT('Ctrl Pts',(0.0307586699497045,-1.26730161813769,
1.10157231096021));
#22808=CARTESIAN_POINT('Ctrl Pts',(0.0935930593956122,-1.52910049789876,
1.31988785480616));
#22809=CARTESIAN_POINT('Ctrl Pts',(0.288504466724427,-1.69600411129882,
1.49890963328681));
#22810=CARTESIAN_POINT('Ctrl Pts',(0.615492891936149,-1.76801245833785,
1.63863764640215));
#22811=CARTESIAN_POINT('Ctrl Pts',(0.0104540016207175,-1.24075075344812,
1.12589971949673));
#22812=CARTESIAN_POINT('Ctrl Pts',(0.0678859432465663,-1.4979766733267,
1.34900830339198));
#22813=CARTESIAN_POINT('Ctrl Pts',(0.256119480862723,-1.66433379116766,
1.53195557707746));
#22814=CARTESIAN_POINT('Ctrl Pts',(0.575041124025717,-1.73991331668443,
1.6747462494124));
#22815=CARTESIAN_POINT('Ctrl Pts',(-0.0181391694102216,-1.19576910668283,
1.16769197379075));
#22816=CARTESIAN_POINT('Ctrl Pts',(0.031367240156502,-1.44497975845611,
1.39903467275813));
#22817=CARTESIAN_POINT('Ctrl Pts',(0.208916886053918,-1.60956344041242,
1.58878224232002));
#22818=CARTESIAN_POINT('Ctrl Pts',(0.514553591586042,-1.68965392328532,
1.73683914729674));
#22819=CARTESIAN_POINT('Ctrl Pts',(-0.0438923944102224,-1.13237144427268,
1.22804151155252));
#22820=CARTESIAN_POINT('Ctrl Pts',(-0.00259486397362604,-1.36948062872853,
1.47142038155714));
#22821=CARTESIAN_POINT('Ctrl Pts',(0.161878639424902,-1.52936917527703,
1.67099694623233));
#22822=CARTESIAN_POINT('Ctrl Pts',(0.449540694258314,-1.61203607707659,
1.82676565001254));
#22823=CARTESIAN_POINT('Ctrl Pts',(-0.0455929113995308,-1.09643283244092,
1.2635364344865));
#22824=CARTESIAN_POINT('Ctrl Pts',(-0.00627769421187312,-1.32612616419273,
1.51398418220584));
#22825=CARTESIAN_POINT('Ctrl Pts',(0.152505158025993,-1.48124586260132,
1.71946457116169));
#22826=CARTESIAN_POINT('Ctrl Pts',(0.430838249779537,-1.56208770129018,
1.87977332297458));
#22827=CARTESIAN_POINT('Ctrl Pts',(-0.042795833893119,-1.07691421721301,
1.28318517919043));
#22828=CARTESIAN_POINT('Ctrl Pts',(-0.00374333123643638,-1.30240853234962,
1.53754499301448));
#22829=CARTESIAN_POINT('Ctrl Pts',(0.152519741700297,-1.45458565734394,
1.74612783237292));
#22830=CARTESIAN_POINT('Ctrl Pts',(0.425993384917082,-1.53344559219597,
1.90893369726574));
#22831=CARTESIAN_POINT('',(-0.0421576093699572,-1.08053472770428,1.28727233489076));
#22832=CARTESIAN_POINT('Ctrl Pts',(0.0260686553993155,-1.26108935601086,
1.10727038327973));
#22833=CARTESIAN_POINT('Ctrl Pts',(0.0102738810212638,-1.2406663502733,
1.12801545944049));
#22834=CARTESIAN_POINT('Ctrl Pts',(-0.00544822415320455,-1.21735780368012,
1.15133239961429));
#22835=CARTESIAN_POINT('Ctrl Pts',(-0.0280274542414684,-1.17324021107675,
1.19509600545504));
#22836=CARTESIAN_POINT('Ctrl Pts',(-0.0355561559109315,-1.15484454191159,
1.21324740617467));
#22837=CARTESIAN_POINT('Ctrl Pts',(-0.0433677241466708,-1.12241703607508,
1.24538218411125));
#22838=CARTESIAN_POINT('Ctrl Pts',(-0.0455044376575851,-1.10404988380792,
1.26364457695041));
#22839=CARTESIAN_POINT('Ctrl Pts',(-0.0421576093699572,-1.08053472770428,
1.28727233489076));
#22840=CARTESIAN_POINT('Ctrl Pts',(-0.0421576093699572,-1.08053472770428,
1.28727233489076));
#22841=CARTESIAN_POINT('Ctrl Pts',(-0.024279158719655,-1.18019989616608,
1.39987124007464));
#22842=CARTESIAN_POINT('Ctrl Pts',(0.0166569869072255,-1.26544208722232,
1.50346488650363));
#22843=CARTESIAN_POINT('Ctrl Pts',(0.16009648734447,-1.42418037408903,1.715480776583));
#22844=CARTESIAN_POINT('Ctrl Pts',(0.275079075974332,-1.48987049850469,
1.81902921434248));
#22845=CARTESIAN_POINT('Ctrl Pts',(0.425598593400271,-1.53333167412,1.90869858745619));
#22846=CARTESIAN_POINT('Ctrl Pts',(-0.0421576093699572,-1.08053472770428,
1.28727233489076));
#22847=CARTESIAN_POINT('Ctrl Pts',(-0.00195919018135123,-1.30462473967982,
1.54044292999952));
#22848=CARTESIAN_POINT('Ctrl Pts',(0.154805815536382,-1.45580038421926,
1.74808806061869));
#22849=CARTESIAN_POINT('Ctrl Pts',(0.428137407783241,-1.5340616613226,1.91020772674828));
#22850=CARTESIAN_POINT('Ctrl Pts',(-0.0853753293366669,-1.07622999908393,
1.28727233489076));
#22851=CARTESIAN_POINT('Ctrl Pts',(-0.0542581740029555,-1.30138937207125,
1.54044292999952));
#22852=CARTESIAN_POINT('Ctrl Pts',(0.0960667204863546,-1.45848408198029,
1.74808806061869));
#22853=CARTESIAN_POINT('Ctrl Pts',(0.365599354131263,-1.54751412881105,
1.91020772674828));
#22854=CARTESIAN_POINT('Ctrl Pts',(-0.128593049303377,-1.07192527046357,
1.28727233489076));
#22855=CARTESIAN_POINT('Ctrl Pts',(-0.10655715782456,-1.29815400446268,
1.54044292999952));
#22856=CARTESIAN_POINT('Ctrl Pts',(0.0373276254363271,-1.46116777974132,
1.74808806061869));
#22857=CARTESIAN_POINT('Ctrl Pts',(0.303061300479284,-1.56096659629949,
1.91020772674828));
#22858=CARTESIAN_POINT('Ctrl Pts',(-0.171810769270086,-1.06762054184321,
1.28727233489076));
#22859=CARTESIAN_POINT('Ctrl Pts',(-0.158856141646164,-1.29491863685411,
1.54044292999952));
#22860=CARTESIAN_POINT('Ctrl Pts',(-0.0214114696137,-1.46385147750235,1.74808806061869));
#22861=CARTESIAN_POINT('Ctrl Pts',(0.240523246827306,-1.57441906378793,
1.91020772674828));
#22862=CARTESIAN_POINT('Ctrl Pts',(-0.0421576093699572,-1.08053472770428,
1.28727233489076));
#22863=CARTESIAN_POINT('Ctrl Pts',(-0.0637496973860272,-1.07899219081063,
1.28797191329046));
#22864=CARTESIAN_POINT('Ctrl Pts',(-0.0853207093795707,-1.07715333835806,
1.28831907556383));
#22865=CARTESIAN_POINT('Ctrl Pts',(-0.106872735707655,-1.07501072349525,
1.288319084765));
#22866=CARTESIAN_POINT('Ctrl Pts',(-0.128559621036833,-1.07285470149866,
1.28831909402374));
#22867=CARTESIAN_POINT('Ctrl Pts',(-0.150205375722342,-1.07039324377381,
1.28796761487395));
#22868=CARTESIAN_POINT('Ctrl Pts',(-0.171810769270086,-1.06762054184321,
1.28727233489076));
#22869=CARTESIAN_POINT('Origin',(0.,0.,1.37171309575435));
#22870=CARTESIAN_POINT('',(-0.36490527784414,-1.20742290720348,1.10727038327973));
#22871=CARTESIAN_POINT('Ctrl Pts',(0.0276890267571667,-1.86363850813291,
1.63615580822897));
#22872=CARTESIAN_POINT('Ctrl Pts',(-0.0698239366988097,-1.80655480211407,
1.58477934055792));
#22873=CARTESIAN_POINT('Ctrl Pts',(-0.14869194528843,-1.74187241700968,
1.53343685544663));
#22874=CARTESIAN_POINT('Ctrl Pts',(-0.274785130849248,-1.59669345888594,
1.42076782591243));
#22875=CARTESIAN_POINT('Ctrl Pts',(-0.320436333138567,-1.51444831269989,
1.35830292226021));
#22876=CARTESIAN_POINT('Ctrl Pts',(-0.36627106501613,-1.35321270714143,
1.23020598103186));
#22877=CARTESIAN_POINT('Ctrl Pts',(-0.371649422530895,-1.27957619027631,
1.16961370091491));
#22878=CARTESIAN_POINT('Ctrl Pts',(-0.364905277844141,-1.20742290720348,
1.10727038327973));
#22879=CARTESIAN_POINT('Origin',(0.,0.,1.10727038327973));
#22880=CARTESIAN_POINT('Ctrl Pts',(-0.492368803403902,-0.958722904333223,
1.28318567027397));
#22881=CARTESIAN_POINT('Ctrl Pts',(-0.551909716442827,-1.17966054547972,
1.53751096017971));
#22882=CARTESIAN_POINT('Ctrl Pts',(-0.474301142999538,-1.38346957888851,
1.74607168007007));
#22883=CARTESIAN_POINT('Ctrl Pts',(-0.259543083074032,-1.57015000455958,
1.90886782994505));
#22884=CARTESIAN_POINT('Ctrl Pts',(-0.497730308181424,-0.97247283635693,
1.26847940010162));
#22885=CARTESIAN_POINT('Ctrl Pts',(-0.557797896845799,-1.196516618136,1.51987665322458));
#22886=CARTESIAN_POINT('Ctrl Pts',(-0.478816264707968,-1.40288697684033,
1.72611612827484));
#22887=CARTESIAN_POINT('Ctrl Pts',(-0.260856494176601,-1.59185117960571,
1.88704325648016));
#22888=CARTESIAN_POINT('Ctrl Pts',(-0.510779460904228,-0.996638068239391,
1.24117819097188));
#22889=CARTESIAN_POINT('Ctrl Pts',(-0.572460097309861,-1.22627731830139,
1.48716579746039));
#22890=CARTESIAN_POINT('Ctrl Pts',(-0.491635127338186,-1.43799804358595,
1.68888670640878));
#22891=CARTESIAN_POINT('Ctrl Pts',(-0.268313724592158,-1.63180052564182,
1.84634350908918));
#22892=CARTESIAN_POINT('Ctrl Pts',(-0.557803663431837,-1.04217697649275,
1.18072535874295));
#22893=CARTESIAN_POINT('Ctrl Pts',(-0.62733559714006,-1.28344787385866,
1.41461088358276));
#22894=CARTESIAN_POINT('Ctrl Pts',(-0.546077997260112,-1.50844372983685,
1.60644436926605));
#22895=CARTESIAN_POINT('Ctrl Pts',(-0.314053900652124,-1.71730828939988,
1.75613814413928));
#22896=CARTESIAN_POINT('Ctrl Pts',(-0.608738508149428,-1.07063174084474,
1.13430117558029));
#22897=CARTESIAN_POINT('Ctrl Pts',(-0.687608854742564,-1.32002833380447,
1.35902160674437));
#22898=CARTESIAN_POINT('Ctrl Pts',(-0.608917570976486,-1.55649910176849,
1.54332567193683));
#22899=CARTESIAN_POINT('Ctrl Pts',(-0.372863601758234,-1.78021953810236,
1.68715809360678));
#22900=CARTESIAN_POINT('Ctrl Pts',(-0.649605006049397,-1.08812946536139,
1.10192284729582));
#22901=CARTESIAN_POINT('Ctrl Pts',(-0.736085457637467,-1.34295142581462,
1.32027771712106));
#22902=CARTESIAN_POINT('Ctrl Pts',(-0.660325994321481,-1.58796351671871,
1.49933702411959));
#22903=CARTESIAN_POINT('Ctrl Pts',(-0.422326616101438,-1.82316573807367,
1.63910076829143));
#22904=CARTESIAN_POINT('',(-0.493314642657339,-0.962275025729455,1.28727233489076));
#22905=CARTESIAN_POINT('',(-0.642908916934723,-1.08521613661244,1.10727038327973));
#22906=CARTESIAN_POINT('Ctrl Pts',(-0.493314642657339,-0.962275025729455,
1.28727233489076));
#22907=CARTESIAN_POINT('Ctrl Pts',(-0.505155444616883,-0.992714976574576,
1.25478273943443));
#22908=CARTESIAN_POINT('Ctrl Pts',(-0.522900410114185,-1.0134702004972,
1.22829923781244));
#22909=CARTESIAN_POINT('Ctrl Pts',(-0.572202237708348,-1.05095536138805,
1.17205963503303));
#22910=CARTESIAN_POINT('Ctrl Pts',(-0.603178396561744,-1.06919273067066,
1.14130666672502));
#22911=CARTESIAN_POINT('Ctrl Pts',(-0.642908916934723,-1.08521613661244,
1.10727038327973));
#22912=CARTESIAN_POINT('Ctrl Pts',(-0.493314642657339,-0.962275025729455,
1.28727233489076));
#22913=CARTESIAN_POINT('Ctrl Pts',(-0.519074140629024,-1.06019965524839,
1.39987124007464));
#22914=CARTESIAN_POINT('Ctrl Pts',(-0.517846241724568,-1.15475382712427,
1.50346488650363));
#22915=CARTESIAN_POINT('Ctrl Pts',(-0.454602843714802,-1.35913828497575,
1.715480776583));
#22916=CARTESIAN_POINT('Ctrl Pts',(-0.377981286365637,-1.46714441944577,
1.81902921434248));
#22917=CARTESIAN_POINT('Ctrl Pts',(-0.259766273896474,-1.5699559447672,
1.90869858745619));
#22918=CARTESIAN_POINT('Ctrl Pts',(-0.642908916934723,-1.08521613661244,
1.10727038327973));
#22919=CARTESIAN_POINT('Ctrl Pts',(-0.668710261798003,-1.16760035714813,
1.18103565901042));
#22920=CARTESIAN_POINT('Ctrl Pts',(-0.681355585835302,-1.25518160519556,
1.25302429310885));
#22921=CARTESIAN_POINT('Ctrl Pts',(-0.665371573463992,-1.44098614169382,
1.39260788389873));
#22922=CARTESIAN_POINT('Ctrl Pts',(-0.63530114956013,-1.53389259595497,
1.45574709063856));
#22923=CARTESIAN_POINT('Ctrl Pts',(-0.541698310562567,-1.69239761845938,
1.55895701082587));
#22924=CARTESIAN_POINT('Ctrl Pts',(-0.489122861296312,-1.75616935678546,
1.59904902099409));
#22925=CARTESIAN_POINT('Ctrl Pts',(-0.428377445609995,-1.81394816223928,
1.63615580822897));
#22926=CARTESIAN_POINT('Ctrl Pts',(-0.362330138275325,-1.21487793679796,
1.10149705943222));
#22927=CARTESIAN_POINT('Ctrl Pts',(-0.383459937582896,-1.4832989591636,
1.31979778023781));
#22928=CARTESIAN_POINT('Ctrl Pts',(-0.249644960941924,-1.70227260218964,
1.49880741124996));
#22929=CARTESIAN_POINT('Ctrl Pts',(0.039114791647589,-1.87179886587609,
1.63852595246867));
#22930=CARTESIAN_POINT('Ctrl Pts',(-0.373447482460585,-1.18333690797344,
1.12583385309083));
#22931=CARTESIAN_POINT('Ctrl Pts',(-0.3983051825378,-1.4457367248385,1.34892944774501));
#22932=CARTESIAN_POINT('Ctrl Pts',(-0.270675994878911,-1.66212671668264,
1.5318660237053));
#22933=CARTESIAN_POINT('Ctrl Pts',(0.0093036513012339,-1.83255854794257,
1.67464838892921));
#22934=CARTESIAN_POINT('Ctrl Pts',(-0.386758017000778,-1.13169790455623,
1.16764044916317));
#22935=CARTESIAN_POINT('Ctrl Pts',(-0.416680587119745,-1.38402127269752,
1.39897336709084));
#22936=CARTESIAN_POINT('Ctrl Pts',(-0.298670375694665,-1.59542335194443,
1.58871211231352));
#22937=CARTESIAN_POINT('Ctrl Pts',(-0.0327265383253417,-1.76604232095016,
1.73676275687621));
#22938=CARTESIAN_POINT('Ctrl Pts',(-0.391671741837561,-1.06341115236231,
1.2280160761933));
#22939=CARTESIAN_POINT('Ctrl Pts',(-0.425665904909547,-1.30168216224368,
1.47139032317727));
#22940=CARTESIAN_POINT('Ctrl Pts',(-0.318647566754324,-1.50457544636211,
1.67096220367119));
#22941=CARTESIAN_POINT('Ctrl Pts',(-0.0706042875438574,-1.67209124376878,
1.82672793765153));
#22942=CARTESIAN_POINT('Ctrl Pts',(-0.38218165487343,-1.0286884268729,1.263527751515));
#22943=CARTESIAN_POINT('Ctrl Pts',(-0.415770412604395,-1.25929056133868,
1.51397381108002));
#22944=CARTESIAN_POINT('Ctrl Pts',(-0.312692596804326,-1.45588630034145,
1.71945276482243));
#22945=CARTESIAN_POINT('Ctrl Pts',(-0.0729619965738882,-1.61878272768801,
1.8797604367197));
#22946=CARTESIAN_POINT('Ctrl Pts',(-0.373486051297297,-1.01098164381094,
1.28318517919159));
#22947=CARTESIAN_POINT('Ctrl Pts',(-0.40602648967972,-1.23750736860246,
1.53754499301511));
#22948=CARTESIAN_POINT('Ctrl Pts',(-0.304436793685258,-1.43052436008972,
1.74612783237315));
#22949=CARTESIAN_POINT('Ctrl Pts',(-0.0687169633139101,-1.59003261827273,
1.90893369726572));
#22950=CARTESIAN_POINT('',(-0.373997862975654,-1.01462217612883,1.28727233489076));
#22951=CARTESIAN_POINT('Ctrl Pts',(-0.364905277844141,-1.20742290720348,
1.10727038327973));
#22952=CARTESIAN_POINT('Ctrl Pts',(-0.373615945090689,-1.18311862080926,
1.12801545944052));
#22953=CARTESIAN_POINT('Ctrl Pts',(-0.381365818655258,-1.15609247800023,
1.15133239961429));
#22954=CARTESIAN_POINT('Ctrl Pts',(-0.389206856698301,-1.10715678825424,
1.19509600545515));
#22955=CARTESIAN_POINT('Ctrl Pts',(-0.390682503085324,-1.08733497046169,
1.21324740617476));
#22956=CARTESIAN_POINT('Ctrl Pts',(-0.388091095569743,-1.05408067239125,
1.24538218411121));
#22957=CARTESIAN_POINT('Ctrl Pts',(-0.384447468688947,-1.0359521917548,
1.26364457695037));
#22958=CARTESIAN_POINT('Ctrl Pts',(-0.373997862975654,-1.01462217612883,
1.28727233489076));
#22959=CARTESIAN_POINT('Ctrl Pts',(-0.373997862975654,-1.01462217612883,
1.28727233489076));
#22960=CARTESIAN_POINT('Ctrl Pts',(-0.387792676785359,-1.11493412912611,
1.39987124007464));
#22961=CARTESIAN_POINT('Ctrl Pts',(-0.375201374409042,-1.20865423507634,
1.50346488650363));
#22962=CARTESIAN_POINT('Ctrl Pts',(-0.287835131123856,-1.40394856048621,
1.715480776583));
#22963=CARTESIAN_POINT('Ctrl Pts',(-0.198779555753984,-1.50195515531182,
1.81902921434248));
#22964=CARTESIAN_POINT('Ctrl Pts',(-0.0690572297370888,-1.58980227845634,
1.90869858745619));
#22965=CARTESIAN_POINT('Ctrl Pts',(-0.373997862975653,-1.01462217612883,
1.28727233489076));
#22966=CARTESIAN_POINT('Ctrl Pts',(-0.405014516431691,-1.24016643693111,
1.54044292999952));
#22967=CARTESIAN_POINT('Ctrl Pts',(-0.302637979515068,-1.43238606966553,
1.74808806061869));
#22968=CARTESIAN_POINT('Ctrl Pts',(-0.0668682522257825,-1.59128107433209,
1.91020772674828));
#22969=CARTESIAN_POINT('Ctrl Pts',(-0.413770122869549,-0.997173125995706,
1.28727233489076));
#22970=CARTESIAN_POINT('Ctrl Pts',(-0.453754022216744,-1.22092814469495,
1.54044292999952));
#22971=CARTESIAN_POINT('Ctrl Pts',(-0.359331486839601,-1.41678703930426,
1.74808806061869));
#22972=CARTESIAN_POINT('Ctrl Pts',(-0.130502516738118,-1.58474980982363,
1.91020772674828));
#22973=CARTESIAN_POINT('Ctrl Pts',(-0.453542382763444,-0.979724075862581,
1.28727233489076));
#22974=CARTESIAN_POINT('Ctrl Pts',(-0.502493528001797,-1.2016898524588,
1.54044292999952));
#22975=CARTESIAN_POINT('Ctrl Pts',(-0.416024994164134,-1.40118800894299,
1.74808806061869));
#22976=CARTESIAN_POINT('Ctrl Pts',(-0.194136781250454,-1.57821854531517,
1.91020772674828));
#22977=CARTESIAN_POINT('Ctrl Pts',(-0.493314642657339,-0.962275025729455,
1.28727233489076));
#22978=CARTESIAN_POINT('Ctrl Pts',(-0.55123303378685,-1.18245156022264,
1.54044292999952));
#22979=CARTESIAN_POINT('Ctrl Pts',(-0.472718501488667,-1.38558897858172,
1.74808806061869));
#22980=CARTESIAN_POINT('Ctrl Pts',(-0.257771045762789,-1.5716872808067,
1.91020772674828));
#22981=CARTESIAN_POINT('Ctrl Pts',(-0.373997862975653,-1.01462217612883,
1.28727233489076));
#22982=CARTESIAN_POINT('Ctrl Pts',(-0.394056488869187,-1.00648281422348,
1.28797191329047));
#22983=CARTESIAN_POINT('Ctrl Pts',(-0.414003503730723,-0.998068152324091,
1.28831907556383));
#22984=CARTESIAN_POINT('Ctrl Pts',(-0.433838594404394,-0.989370462098315,
1.288319084765));
#22985=CARTESIAN_POINT('Ctrl Pts',(-0.453797800577657,-0.980618347207412,
1.28831909402374));
#22986=CARTESIAN_POINT('Ctrl Pts',(-0.473623504353515,-0.971588455744714,
1.28796761487395));
#22987=CARTESIAN_POINT('Ctrl Pts',(-0.493314642657339,-0.962275025729455,
1.28727233489076));
#22988=CARTESIAN_POINT('Origin',(0.,0.,1.37171309575435));
#22989=CARTESIAN_POINT('',(-0.720159740047642,-1.03556549162895,1.10727038327973));
#22990=CARTESIAN_POINT('Ctrl Pts',(-0.549562141057369,-1.78098192700405,
1.63615580822897));
#22991=CARTESIAN_POINT('Ctrl Pts',(-0.620893161259053,-1.70079633666903,
1.58735805514616));
#22992=CARTESIAN_POINT('Ctrl Pts',(-0.67413336725818,-1.61925404078178,
1.53858095020846));
#22993=CARTESIAN_POINT('Ctrl Pts',(-0.751969574388241,-1.44461319502364,
1.42806953503217));
#22994=CARTESIAN_POINT('Ctrl Pts',(-0.772017157909609,-1.35007152673693,
1.36461306044574));
#22995=CARTESIAN_POINT('Ctrl Pts',(-0.767479006699504,-1.17779635313151,
1.23357020765533));
#22996=CARTESIAN_POINT('Ctrl Pts',(-0.749676646324456,-1.10397180136273,
1.17136442658357));
#22997=CARTESIAN_POINT('Ctrl Pts',(-0.720159740047643,-1.03556549162895,
1.10727038327973));
#22998=CARTESIAN_POINT('Origin',(0.,0.,1.10727038327973));
#22999=CARTESIAN_POINT('Ctrl Pts',(-0.764532229233201,-0.759649337735664,
1.28318567027397));
#23000=CARTESIAN_POINT('Ctrl Pts',(-0.889432488376416,-0.951374367053292,
1.53751096017971));
#23001=CARTESIAN_POINT('Ctrl Pts',(-0.87860280381325,-1.16919064445971,
1.74607168007007));
#23002=CARTESIAN_POINT('Ctrl Pts',(-0.732043175543704,-1.4130981699549,
1.90886782994505));
#23003=CARTESIAN_POINT('Ctrl Pts',(-0.773880285955837,-0.771069504093749,
1.26847940010162));
#23004=CARTESIAN_POINT('Ctrl Pts',(-0.900241293626992,-0.965585896981723,
1.51987665322458));
#23005=CARTESIAN_POINT('Ctrl Pts',(-0.888897245689575,-1.18626243797171,
1.72611612827484));
#23006=CARTESIAN_POINT('Ctrl Pts',(-0.739998335618538,-1.43333134754249,
1.88704325648016));
#23007=CARTESIAN_POINT('Ctrl Pts',(-0.793756470105422,-0.79001938035927,
1.24117952306876));
#23008=CARTESIAN_POINT('Ctrl Pts',(-0.923380672132909,-0.989358920654668,
1.48716712955727));
#23009=CARTESIAN_POINT('Ctrl Pts',(-0.911936310735738,-1.21569285383181,
1.68888851879237));
#23010=CARTESIAN_POINT('Ctrl Pts',(-0.759433295933266,-1.4690200759214,
1.84634532147277));
#23011=CARTESIAN_POINT('Ctrl Pts',(-0.852549487780078,-0.818798433422952,
1.18072779772815));
#23012=CARTESIAN_POINT('Ctrl Pts',(-0.993235093958044,-1.02677414338758,
1.41461332256795));
#23013=CARTESIAN_POINT('Ctrl Pts',(-0.985480669746803,-1.26586652272338,
1.60644767971085));
#23014=CARTESIAN_POINT('Ctrl Pts',(-0.829355339157893,-1.53620791207527,
1.75614145458407));
#23015=CARTESIAN_POINT('Ctrl Pts',(-0.909788127533563,-0.830120749534188,
1.13430117558028));
#23016=CARTESIAN_POINT('Ctrl Pts',(-1.06186607016719,-1.04293872696083,
1.35902160674436));
#23017=CARTESIAN_POINT('Ctrl Pts',(-1.06009969793961,-1.29215273573923,
1.54332567193682));
#23018=CARTESIAN_POINT('Ctrl Pts',(-0.904732449133398,-1.57786820262105,
1.68715809360678));
#23019=CARTESIAN_POINT('Ctrl Pts',(-0.954061570898026,-0.834133632104406,
1.10192284729582));
#23020=CARTESIAN_POINT('Ctrl Pts',(-1.115053684233,-1.04975978886662,1.32027771712106));
#23021=CARTESIAN_POINT('Ctrl Pts',(-1.11871505289201,-1.30619109614143,
1.49933702411959));
#23022=CARTESIAN_POINT('Ctrl Pts',(-0.965045676875064,-1.60342755392882,
1.63910076829143));
#23023=CARTESIAN_POINT('',(-0.766529441696069,-0.762735325532963,1.28727233489076));
#23024=CARTESIAN_POINT('',(-0.946792943618195,-0.833432097145889,1.10727038327973));
#23025=CARTESIAN_POINT('Ctrl Pts',(-0.766529441696069,-0.762735325532963,
1.28727233489076));
#23026=CARTESIAN_POINT('Ctrl Pts',(-0.787197175677101,-0.788026430107593,
1.25478273943417));
#23027=CARTESIAN_POINT('Ctrl Pts',(-0.810487357658964,-0.80228232516309,
1.22829923781215));
#23028=CARTESIAN_POINT('Ctrl Pts',(-0.868959733810231,-0.822697729112325,
1.17205963503244));
#23029=CARTESIAN_POINT('Ctrl Pts',(-0.904055468578107,-0.83047033850234,
1.14130666672486));
#23030=CARTESIAN_POINT('Ctrl Pts',(-0.946792943618196,-0.833432097145889,
1.10727038327973));
#23031=CARTESIAN_POINT('Ctrl Pts',(-0.766529441696069,-0.762735325532963,
1.28727233489076));
#23032=CARTESIAN_POINT('Ctrl Pts',(-0.821288554787752,-0.847907059902912,
1.39987124007464));
#23033=CARTESIAN_POINT('Ctrl Pts',(-0.849339599532016,-0.938212862837218,
1.50346488650363));
#23034=CARTESIAN_POINT('Ctrl Pts',(-0.852349824604396,-1.15213731807335,
1.715480776583));
#23035=CARTESIAN_POINT('Ctrl Pts',(-0.812854124246773,-1.27853461941729,
1.81902921434248));
#23036=CARTESIAN_POINT('Ctrl Pts',(-0.732195474855993,-1.41284463836769,
1.90869858745619));
#23037=CARTESIAN_POINT('Ctrl Pts',(-0.946792943618196,-0.833432097145889,
1.10727038327973));
#23038=CARTESIAN_POINT('Ctrl Pts',(-0.99678960499347,-0.90381109288579,
1.18103565901043));
#23039=CARTESIAN_POINT('Ctrl Pts',(-1.03588011685504,-0.983198189519685,
1.25302429310889));
#23040=CARTESIAN_POINT('Ctrl Pts',(-1.07809517714267,-1.16484813617463,
1.39260788389878));
#23041=CARTESIAN_POINT('Ctrl Pts',(-1.07820617779495,-1.26249969691992,
1.4557470906386));
#23042=CARTESIAN_POINT('Ctrl Pts',(-1.03816533347022,-1.44217179941021,
1.55895701082589));
#23043=CARTESIAN_POINT('Ctrl Pts',(-1.007869660752,-1.51906903401084,1.5990490209941));
#23044=CARTESIAN_POINT('Ctrl Pts',(-0.967951970128401,-1.59279130921887,
1.63615580822897));
#23045=CARTESIAN_POINT('Ctrl Pts',(-0.720016914634041,-1.04334803864883,
1.10157231096021));
#23046=CARTESIAN_POINT('Ctrl Pts',(-0.823064346331376,-1.29208090893697,
1.31988785480616));
#23047=CARTESIAN_POINT('Ctrl Pts',(-0.763481187915702,-1.54167481933165,
1.4989096332868));
#23048=CARTESIAN_POINT('Ctrl Pts',(-0.541267439387021,-1.79212976983287,
1.63863764640215));
#23049=CARTESIAN_POINT('Ctrl Pts',(-0.720837529677193,-1.00993315330315,
1.12589971949674));
#23050=CARTESIAN_POINT('Ctrl Pts',(-0.825567715093926,-1.25179094217684,
1.34900830339198));
#23051=CARTESIAN_POINT('Ctrl Pts',(-0.771065844731935,-1.49701757504304,
1.53195557707746));
#23052=CARTESIAN_POINT('Ctrl Pts',(-0.557477346013107,-1.74562013410099,
1.6747462494124));
#23053=CARTESIAN_POINT('Ctrl Pts',(-0.717530565095651,-0.956735633325587,
1.16769179538367));
#23054=CARTESIAN_POINT('Ctrl Pts',(-0.823961384252211,-1.18745042322669,
1.39903449435105));
#23055=CARTESIAN_POINT('Ctrl Pts',(-0.777060632929274,-1.42496257773993,
1.58878199846585));
#23056=CARTESIAN_POINT('Ctrl Pts',(-0.576871348730688,-1.66940588754285,
1.73683890344257));
#23057=CARTESIAN_POINT('Ctrl Pts',(-0.701101131459804,-0.890308540641216,
1.22804130170824));
#23058=CARTESIAN_POINT('Ctrl Pts',(-0.807060009317132,-1.10640797973512,
1.47142017171286));
#23059=CARTESIAN_POINT('Ctrl Pts',(-0.767978311363816,-1.33243573819092,
1.67099665961544));
#23060=CARTESIAN_POINT('Ctrl Pts',(-0.583845206097259,-1.56839818009432,
1.82676536339564));
#23061=CARTESIAN_POINT('Ctrl Pts',(-0.681352489183287,-0.86023395370564,
1.2635364344865));
#23062=CARTESIAN_POINT('Ctrl Pts',(-0.784556163294569,-1.06916866744104,
1.51398418220584));
#23063=CARTESIAN_POINT('Ctrl Pts',(-0.747275208483433,-1.28799335847826,
1.71946457116169));
#23064=CARTESIAN_POINT('Ctrl Pts',(-0.569616647707411,-1.51699586639176,
1.87977332297458));
#23065=CARTESIAN_POINT('Ctrl Pts',(-0.667616851769879,-0.846087143187382,
1.28318517919043));
#23066=CARTESIAN_POINT('Ctrl Pts',(-0.768564946360842,-1.05147036139455,
1.53754499301448));
#23067=CARTESIAN_POINT('Ctrl Pts',(-0.731592934569703,-1.26643337142019,
1.74612783237292));
#23068=CARTESIAN_POINT('Ctrl Pts',(-0.556700816396459,-1.4909761732643,
1.90893369726574));
#23069=CARTESIAN_POINT('',(-0.669228599956957,-0.849391336665505,1.28727233489076));
#23070=CARTESIAN_POINT('Ctrl Pts',(-0.720159740047643,-1.03556549162895,
1.10727038327973));
#23071=CARTESIAN_POINT('Ctrl Pts',(-0.720933639361787,-1.00975899746819,
1.12801545944061));
#23072=CARTESIAN_POINT('Ctrl Pts',(-0.719952669695422,-0.981660765603669,
1.15133239961436));
#23073=CARTESIAN_POINT('Ctrl Pts',(-0.712287980257843,-0.932697144982725,
1.19509600545502));
#23074=CARTESIAN_POINT('Ctrl Pts',(-0.707566124812642,-0.913389476194881,
1.21324740617476));
#23075=CARTESIAN_POINT('Ctrl Pts',(-0.694825406568517,-0.882563548281155,
1.24538218411192));
#23076=CARTESIAN_POINT('Ctrl Pts',(-0.685758102881575,-0.866448281268892,
1.26364457695099));
#23077=CARTESIAN_POINT('Ctrl Pts',(-0.669228599956957,-0.849391336665505,
1.28727233489076));
#23078=CARTESIAN_POINT('Ctrl Pts',(-0.669228599956957,-0.849391336665505,
1.28727233489076));
#23079=CARTESIAN_POINT('Ctrl Pts',(-0.713346345736856,-0.940530841324424,
1.39987124007464));
#23080=CARTESIAN_POINT('Ctrl Pts',(-0.73033241101646,-1.03355488521186,
1.50346488650363));
#23081=CARTESIAN_POINT('Ctrl Pts',(-0.707591441492497,-1.2462884798982,
1.715480776583));
#23082=CARTESIAN_POINT('Ctrl Pts',(-0.653180259586498,-1.36701797678012,
1.81902921434248));
#23083=CARTESIAN_POINT('Ctrl Pts',(-0.55695325007777,-1.49065195897357,
1.90869858745619));
#23084=CARTESIAN_POINT('Ctrl Pts',(-0.669228599956957,-0.849391336665505,
1.28727233489076));
#23085=CARTESIAN_POINT('Ctrl Pts',(-0.76842419991163,-1.05431200258793,
1.54044292999952));
#23086=CARTESIAN_POINT('Ctrl Pts',(-0.73045746052879,-1.26875982659235,
1.74808806061869));
#23087=CARTESIAN_POINT('Ctrl Pts',(-0.555328381808437,-1.49273480867877,
1.91020772674828));
#23088=CARTESIAN_POINT('Ctrl Pts',(-0.701662213869994,-0.820505999621324,
1.28727233489076));
#23089=CARTESIAN_POINT('Ctrl Pts',(-0.808833265245786,-1.02095396380933,
1.54044292999952));
#23090=CARTESIAN_POINT('Ctrl Pts',(-0.779555824624011,-1.23640500988538,
1.74808806061869));
#23091=CARTESIAN_POINT('Ctrl Pts',(-0.613829892004671,-1.46685913784949,
1.91020772674828));
#23092=CARTESIAN_POINT('Ctrl Pts',(-0.734095827783032,-0.791620662577143,
1.28727233489076));
#23093=CARTESIAN_POINT('Ctrl Pts',(-0.849242330579942,-0.98759592503072,
1.54044292999952));
#23094=CARTESIAN_POINT('Ctrl Pts',(-0.828654188719232,-1.20405019317841,
1.74808806061869));
#23095=CARTESIAN_POINT('Ctrl Pts',(-0.672331402200905,-1.4409834670202,
1.91020772674828));
#23096=CARTESIAN_POINT('Ctrl Pts',(-0.766529441696069,-0.762735325532963,
1.28727233489076));
#23097=CARTESIAN_POINT('Ctrl Pts',(-0.889651395914097,-0.954237886252114,
1.54044292999952));
#23098=CARTESIAN_POINT('Ctrl Pts',(-0.877752552814453,-1.17169537647143,
1.74808806061869));
#23099=CARTESIAN_POINT('Ctrl Pts',(-0.730832912397138,-1.41510779619092,
1.91020772674828));
#23100=CARTESIAN_POINT('Ctrl Pts',(-0.669228599956957,-0.849391336665505,
1.28727233489076));
#23101=CARTESIAN_POINT('Ctrl Pts',(-0.685790285668801,-0.835451887202035,
1.28797191329047));
#23102=CARTESIAN_POINT('Ctrl Pts',(-0.702160750604673,-0.821285101590929,
1.28831907556383));
#23103=CARTESIAN_POINT('Ctrl Pts',(-0.718337308749603,-0.806883726521851,
1.288319084765));
#23104=CARTESIAN_POINT('Ctrl Pts',(-0.734615089602745,-0.792392236721729,
1.28831909402374));
#23105=CARTESIAN_POINT('Ctrl Pts',(-0.750680064449572,-0.777677820212515,
1.28796761487395));
#23106=CARTESIAN_POINT('Ctrl Pts',(-0.766529441696069,-0.762735325532963,
1.28727233489076));
#23107=CARTESIAN_POINT('Origin',(0.,0.,1.37171309575435));
#23108=CARTESIAN_POINT('',(-1.00491994924733,-0.762339710524744,1.10727038327973));
#23109=CARTESIAN_POINT('Ctrl Pts',(-1.07301833748062,-1.52399042602929,
1.63615580822897));
#23110=CARTESIAN_POINT('Ctrl Pts',(-1.11607945893998,-1.42568690035961,
1.58735805514608));
#23111=CARTESIAN_POINT('Ctrl Pts',(-1.14151594859478,-1.33168344006462,
1.53858095020836));
#23112=CARTESIAN_POINT('Ctrl Pts',(-1.16157559133822,-1.14153741491428,
1.42806953503214));
#23113=CARTESIAN_POINT('Ctrl Pts',(-1.15142699410503,-1.04542790122455,
1.36461306044571));
#23114=CARTESIAN_POINT('Ctrl Pts',(-1.09387499947176,-0.882986840618228,
1.23357020765531));
#23115=CARTESIAN_POINT('Ctrl Pts',(-1.05413090753298,-0.818276751491846,
1.17136442658356));
#23116=CARTESIAN_POINT('Ctrl Pts',(-1.00491994924733,-0.762339710524744,
1.10727038327973));
#23117=CARTESIAN_POINT('Origin',(0.,0.,1.10727038327973));
#23118=CARTESIAN_POINT('Ctrl Pts',(-0.96185791365589,-0.486216001172379,
1.28318567027397));
#23119=CARTESIAN_POINT('Ctrl Pts',(-1.13989141130718,-0.629961036964704,
1.53751096017972));
#23120=CARTESIAN_POINT('Ctrl Pts',(-1.19690070060403,-0.840463183520971,
1.74607168007008));
#23121=CARTESIAN_POINT('Ctrl Pts',(-1.13288578154644,-1.11772244084118,
1.90886782994506));
#23122=CARTESIAN_POINT('Ctrl Pts',(-0.978417321314553,-0.496846021492854,
1.26357731004417));
#23123=CARTESIAN_POINT('Ctrl Pts',(-1.15940183561927,-0.643585521081937,
1.51399891879436));
#23124=CARTESIAN_POINT('Ctrl Pts',(-1.21707904013549,-0.857895946504487,
1.71946418982836));
#23125=CARTESIAN_POINT('Ctrl Pts',(-1.15131005161592,-1.14010192848643,
1.87976839865855));
#23126=CARTESIAN_POINT('Ctrl Pts',(-1.01174306480633,-0.510215828707942,
1.22814964935774));
#23127=CARTESIAN_POINT('Ctrl Pts',(-1.19911435608045,-0.661178469414082,
1.47151698835253));
#23128=CARTESIAN_POINT('Ctrl Pts',(-1.25929534063486,-0.882459067352747,
1.67109028087187));
#23129=CARTESIAN_POINT('Ctrl Pts',(-1.19229498704013,-1.17406335818981,
1.82686350557264));
#23130=CARTESIAN_POINT('Ctrl Pts',(-1.07994419721084,-0.513157287930765,
1.16792318405109));
#23131=CARTESIAN_POINT('Ctrl Pts',(-1.2814248116504,-0.66776628786098,1.39927998114665));
#23132=CARTESIAN_POINT('Ctrl Pts',(-1.35048605385199,-0.899659869879339,
1.58904519906558));
#23133=CARTESIAN_POINT('Ctrl Pts',(-1.28706885932716,-1.20898915642794,
1.73712239616959));
#23134=CARTESIAN_POINT('Ctrl Pts',(-1.1326179950584,-0.505885563397482,
1.12620659350917));
#23135=CARTESIAN_POINT('Ctrl Pts',(-1.34530596753016,-0.661308446532945,
1.34934531900259));
#23136=CARTESIAN_POINT('Ctrl Pts',(-1.42259827975627,-0.900165347523485,
1.53232296148775));
#23137=CARTESIAN_POINT('Ctrl Pts',(-1.3643546712912,-1.22248177762694,1.67514376227794));
#23138=CARTESIAN_POINT('Ctrl Pts',(-1.16512794184932,-0.498486987186291,
1.10192284729582));
#23139=CARTESIAN_POINT('Ctrl Pts',(-1.38487268717996,-0.653810349677837,
1.32027771712106));
#23140=CARTESIAN_POINT('Ctrl Pts',(-1.46759648753937,-0.896559590305325,
1.4993370241196));
#23141=CARTESIAN_POINT('Ctrl Pts',(-1.41329934292755,-1.22673470906876,
1.63910076829144));
#23142=CARTESIAN_POINT('',(-0.964710998256926,-0.488533777383804,1.28727233489076));
#23143=CARTESIAN_POINT('',(-1.15799828028599,-0.500065917147829,1.10727038327973));
#23144=CARTESIAN_POINT('Ctrl Pts',(-0.964710998256926,-0.488533777383804,
1.28727233489076));
#23145=CARTESIAN_POINT('Ctrl Pts',(-0.992182562456595,-0.506200366158372,
1.25478273943432));
#23146=CARTESIAN_POINT('Ctrl Pts',(-1.01873815563829,-0.512561466012044,
1.22829923781232));
#23147=CARTESIAN_POINT('Ctrl Pts',(-1.08065739676493,-0.51390871103861,
1.17205963503494));
#23148=CARTESIAN_POINT('Ctrl Pts',(-1.11643729240226,-0.510455723374939,
1.14130666672712));
#23149=CARTESIAN_POINT('Ctrl Pts',(-1.15799828028599,-0.500065917147829,
1.10727038327973));
#23150=CARTESIAN_POINT('Ctrl Pts',(-0.964710998256926,-0.488533777383804,
1.28727233489076));
#23151=CARTESIAN_POINT('Ctrl Pts',(-1.04310952295002,-0.552615413818275,
1.39987124007464));
#23152=CARTESIAN_POINT('Ctrl Pts',(-1.09769367964031,-0.629833086622262,
1.50346488650363));
#23153=CARTESIAN_POINT('Ctrl Pts',(-1.16666286599128,-0.832357123065218,
1.715480776583));
#23154=CARTESIAN_POINT('Ctrl Pts',(-1.16815913695893,-0.964772942765737,
1.81902921434248));
#23155=CARTESIAN_POINT('Ctrl Pts',(-1.13295228123076,-1.11743425489732,
1.90869858745619));
#23156=CARTESIAN_POINT('Ctrl Pts',(-1.15799828028599,-0.500065917147829,
1.10727038327973));
#23157=CARTESIAN_POINT('Ctrl Pts',(-1.22729623661063,-0.551550501629614,
1.18103565901045));
#23158=CARTESIAN_POINT('Ctrl Pts',(-1.28900548463586,-0.614972484709007,
1.25302429310892));
#23159=CARTESIAN_POINT('Ctrl Pts',(-1.38528731335188,-0.774686679112438,
1.39260788389881));
#23160=CARTESIAN_POINT('Ctrl Pts',(-1.41556887304307,-0.867524531197708,
1.45574709063864));
#23161=CARTESIAN_POINT('Ctrl Pts',(-1.43300950021463,-1.050776156433,1.55895701082591));
#23162=CARTESIAN_POINT('Ctrl Pts',(-1.42795915557246,-1.13327165021093,
1.59904902099411));
#23163=CARTESIAN_POINT('Ctrl Pts',(-1.4127766116927,-1.21572094522251,1.63615580822897));
#23164=CARTESIAN_POINT('Ctrl Pts',(-1.0071890534957,-0.76978548806141,1.1015723109602));
#23165=CARTESIAN_POINT('Ctrl Pts',(-1.18205566887762,-0.974501097544571,
1.31988785480615));
#23166=CARTESIAN_POINT('Ctrl Pts',(-1.2025174778094,-1.230291220982,1.4989096332868));
#23167=CARTESIAN_POINT('Ctrl Pts',(-1.06857448029104,-1.53715585837368,
1.63863764640214));
#23168=CARTESIAN_POINT('Ctrl Pts',(-0.994461965292035,-0.727074783470153,
1.13400885567558));
#23169=CARTESIAN_POINT('Ctrl Pts',(-1.1685858430854,-0.922448816386927,
1.35870212368824));
#23170=CARTESIAN_POINT('Ctrl Pts',(-1.19383871456862,-1.17054629234372,
1.5429783372848));
#23171=CARTESIAN_POINT('Ctrl Pts',(-1.06996683960028,-1.47149928669632,
1.6867824504158));
#23172=CARTESIAN_POINT('Ctrl Pts',(-0.971974682567373,-0.673083751047334,
1.18052322600159));
#23173=CARTESIAN_POINT('Ctrl Pts',(-1.14389365895071,-0.856229621362336,
1.41439979544558));
#23174=CARTESIAN_POINT('Ctrl Pts',(-1.17420151395341,-1.0936426848353,1.60622137130565));
#23175=CARTESIAN_POINT('Ctrl Pts',(-1.06281232835789,-1.38546708108516,
1.75589800730001));
#23176=CARTESIAN_POINT('Ctrl Pts',(-0.932030917609334,-0.621030952892817,
1.24109849008297));
#23177=CARTESIAN_POINT('Ctrl Pts',(-1.09790581924279,-0.791463701885435,
1.48710325590113));
#23178=CARTESIAN_POINT('Ctrl Pts',(-1.13059499103696,-1.01576709402367,
1.6888327560127));
#23179=CARTESIAN_POINT('Ctrl Pts',(-1.03008879377588,-1.29394102274663,
1.84628852230556));
#23180=CARTESIAN_POINT('Ctrl Pts',(-0.909472892481624,-0.605279141158067,
1.26844862066248));
#23181=CARTESIAN_POINT('Ctrl Pts',(-1.07134082867159,-0.771469550259548,
1.51987386218776));
#23182=CARTESIAN_POINT('Ctrl Pts',(-1.10338745862407,-0.990137606500526,
1.72613059618619));
#23183=CARTESIAN_POINT('Ctrl Pts',(-1.00543407447983,-1.26153883267189,
1.88706341654737));
#23184=CARTESIAN_POINT('Ctrl Pts',(-0.89639666323125,-0.598371737953918,
1.28318517919043));
#23185=CARTESIAN_POINT('Ctrl Pts',(-1.055870911185,-0.762508109189138,1.53754499301448));
#23186=CARTESIAN_POINT('Ctrl Pts',(-1.08713566171041,-0.978375060596136,
1.74612783237291));
#23187=CARTESIAN_POINT('Ctrl Pts',(-0.990190914807483,-1.24597259217491,
1.90893369726573));
#23188=CARTESIAN_POINT('',(-0.89895057878464,-0.601016155111926,1.28727233489076));
#23189=CARTESIAN_POINT('Ctrl Pts',(-1.00491994924733,-0.762339710524744,
1.10727038327973));
#23190=CARTESIAN_POINT('Ctrl Pts',(-0.997681325972045,-0.737557128050268,
1.12801545944073));
#23191=CARTESIAN_POINT('Ctrl Pts',(-0.98806553722046,-0.711137257836932,
1.15133239961458));
#23192=CARTESIAN_POINT('Ctrl Pts',(-0.965645393507087,-0.666938606676028,
1.19509600545601));
#23193=CARTESIAN_POINT('Ctrl Pts',(-0.955188244339595,-0.650035056038689,
1.2132474061757));
#23194=CARTESIAN_POINT('Ctrl Pts',(-0.933545365639423,-0.624654954884534,
1.24538218411151));
#23195=CARTESIAN_POINT('Ctrl Pts',(-0.9199419560071,-0.612130376112957,
1.26364457695062));
#23196=CARTESIAN_POINT('Ctrl Pts',(-0.89895057878464,-0.601016155111926,
1.28727233489076));
#23197=CARTESIAN_POINT('Ctrl Pts',(-0.89895057878464,-0.601016155111926,
1.28727233489076));
#23198=CARTESIAN_POINT('Ctrl Pts',(-0.969072704191387,-0.674061841710201,
1.39987124007464));
#23199=CARTESIAN_POINT('Ctrl Pts',(-1.01397342270847,-0.757283981982513,
1.50346488650363));
#23200=CARTESIAN_POINT('Ctrl Pts',(-1.05808377148838,-0.966632999495317,
1.715480776583));
#23201=CARTESIAN_POINT('Ctrl Pts',(-1.04364312863621,-1.09826755410688,
1.81902921434248));
#23202=CARTESIAN_POINT('Ctrl Pts',(-0.990330805779366,-1.24558623976355,
1.90869858745619));
#23203=CARTESIAN_POINT('Ctrl Pts',(-0.89895057878464,-0.601016155111926,
1.28727233489076));
#23204=CARTESIAN_POINT('Ctrl Pts',(-1.056615168778,-0.765254163607779,1.54044292999952));
#23205=CARTESIAN_POINT('Ctrl Pts',(-1.08677467590956,-0.980938531722802,
1.74808806061869));
#23206=CARTESIAN_POINT('Ctrl Pts',(-0.989429100179333,-1.24806925945699,
1.91020772674828));
#23207=CARTESIAN_POINT('Ctrl Pts',(-0.920870718608735,-0.563522029202552,
1.28727233489076));
#23208=CARTESIAN_POINT('Ctrl Pts',(-1.08473827279984,-0.721041695541498,
1.54044292999951));
#23209=CARTESIAN_POINT('Ctrl Pts',(-1.12347180680942,-0.934995043558669,
1.74808806061869));
#23210=CARTESIAN_POINT('Ctrl Pts',(-1.03707132063747,-1.20538207325406,
1.91020772674828));
#23211=CARTESIAN_POINT('Ctrl Pts',(-0.94279085843283,-0.526027903293178,
1.28727233489076));
#23212=CARTESIAN_POINT('Ctrl Pts',(-1.11286137682168,-0.676829227475217,
1.54044292999952));
#23213=CARTESIAN_POINT('Ctrl Pts',(-1.16016893770927,-0.889051555394535,
1.74808806061869));
#23214=CARTESIAN_POINT('Ctrl Pts',(-1.0847135410956,-1.16269488705113,1.91020772674828));
#23215=CARTESIAN_POINT('Ctrl Pts',(-0.964710998256926,-0.488533777383804,
1.28727233489076));
#23216=CARTESIAN_POINT('Ctrl Pts',(-1.14098448084351,-0.632616759408936,
1.54044292999952));
#23217=CARTESIAN_POINT('Ctrl Pts',(-1.19686606860912,-0.843108067230401,
1.74808806061869));
#23218=CARTESIAN_POINT('Ctrl Pts',(-1.13235576155374,-1.1200077008482,1.91020772674828));
#23219=CARTESIAN_POINT('Ctrl Pts',(-0.89895057878464,-0.601016155111926,
1.28727233489076));
#23220=CARTESIAN_POINT('Ctrl Pts',(-0.910394151125288,-0.582641108525654,
1.28797191329047));
#23221=CARTESIAN_POINT('Ctrl Pts',(-0.921585610967828,-0.564108942884259,
1.28831907556383));
#23222=CARTESIAN_POINT('Ctrl Pts',(-0.932520162364073,-0.545413589903933,
1.288319084765));
#23223=CARTESIAN_POINT('Ctrl Pts',(-0.94352313529324,-0.526601253184352,
1.28831909402374));
#23224=CARTESIAN_POINT('Ctrl Pts',(-0.954254829541783,-0.507642661237889,
1.28796761487395));
#23225=CARTESIAN_POINT('Ctrl Pts',(-0.964710998256926,-0.488533777383804,
1.28727233489076));
#23226=CARTESIAN_POINT('Origin',(0.,0.,1.37171309575435));
#23227=CARTESIAN_POINT('',(-1.19131159212569,-0.414490807021284,1.10727038327973));
#23228=CARTESIAN_POINT('Ctrl Pts',(-1.4914400228729,-1.11782012388912,1.63615580822897));
#23229=CARTESIAN_POINT('Ctrl Pts',(-1.50201612299691,-1.01102129689832,
1.58735805514605));
#23230=CARTESIAN_POINT('Ctrl Pts',(-1.49715899547356,-0.913758385849903,
1.53858095020832));
#23231=CARTESIAN_POINT('Ctrl Pts',(-1.45747849623496,-0.726719999074295,
1.42806953503212));
#23232=CARTESIAN_POINT('Ctrl Pts',(-1.41812713365384,-0.638450508815843,
1.3646130604457));
#23233=CARTESIAN_POINT('Ctrl Pts',(-1.31319488582045,-0.501744424014171,
1.23357020765531));
#23234=CARTESIAN_POINT('Ctrl Pts',(-1.25539949095026,-0.452483071915572,
1.17136442658356));
#23235=CARTESIAN_POINT('Ctrl Pts',(-1.19131159212569,-0.414490807021284,
1.10727038327973));
#23236=CARTESIAN_POINT('Origin',(0.,0.,1.10727038327973));
#23237=CARTESIAN_POINT('Ctrl Pts',(-1.06503024383179,-0.165188454748262,
1.28318567027397));
#23238=CARTESIAN_POINT('Ctrl Pts',(-1.27876982080873,-0.246882731381368,
1.53751096017971));
#23239=CARTESIAN_POINT('Ctrl Pts',(-1.39803761752214,-0.429465330327849,
1.74607168007007));
#23240=CARTESIAN_POINT('Ctrl Pts',(-1.42283363397203,-0.712936251587706,
1.90886782994504));
#23241=CARTESIAN_POINT('Ctrl Pts',(-1.07930558594879,-0.168932913531384,
1.26847940010162));
#23242=CARTESIAN_POINT('Ctrl Pts',(-1.29586765564978,-0.252026844288348,
1.51987665322458));
#23243=CARTESIAN_POINT('Ctrl Pts',(-1.41640054440423,-0.437225780288037,
1.72611612827483));
#23244=CARTESIAN_POINT('Ctrl Pts',(-1.44116225705855,-0.72462931033466,
1.88704325648016));
#23245=CARTESIAN_POINT('Ctrl Pts',(-1.10652474870095,-0.172580460092752,
1.24117906537517));
#23246=CARTESIAN_POINT('Ctrl Pts',(-1.32856177300787,-0.25765834155068,
1.48716667186367));
#23247=CARTESIAN_POINT('Ctrl Pts',(-1.45233913898615,-0.447493258920474,
1.68888789608759));
#23248=CARTESIAN_POINT('Ctrl Pts',(-1.47786361346602,-0.742078309759777,
1.84634469876799));
#23249=CARTESIAN_POINT('Ctrl Pts',(-1.171005693206,-0.161305070542798,1.18072695962337));
#23250=CARTESIAN_POINT('Ctrl Pts',(-1.40706779462018,-0.246868029800143,
1.41461248446317));
#23251=CARTESIAN_POINT('Ctrl Pts',(-1.5413299739097,-0.444855864337685,
1.60644654213682));
#23252=CARTESIAN_POINT('Ctrl Pts',(-1.57392460995617,-0.755334809435743,
1.75614031701005));
#23253=CARTESIAN_POINT('Ctrl Pts',(-1.22396679065339,-0.136821749681419,
1.13430117558029));
#23254=CARTESIAN_POINT('Ctrl Pts',(-1.47209169926766,-0.219605938249046,
1.35902160674436));
#23255=CARTESIAN_POINT('Ctrl Pts',(-1.61714699314177,-0.422262554132505,
1.54332567193681));
#23256=CARTESIAN_POINT('Ctrl Pts',(-1.65939158627326,-0.744733799933205,
1.68715809360676));
#23257=CARTESIAN_POINT('Ctrl Pts',(-1.26214347192869,-0.114044962799315,
1.10192284729582));
#23258=CARTESIAN_POINT('Ctrl Pts',(-1.51913070253035,-0.193861398098009,
1.32027771712105));
#23259=CARTESIAN_POINT('Ctrl Pts',(-1.67281935264037,-0.399166585072132,
1.49933702411959));
#23260=CARTESIAN_POINT('Ctrl Pts',(-1.72320942225875,-0.729960523721685,
1.63910076829142));
#23261=CARTESIAN_POINT('',(-1.06845992077163,-0.166511139289342,1.28727233489076));
#23262=CARTESIAN_POINT('',(-1.25585067703094,-0.117749801015222,1.10727038327973));
#23263=CARTESIAN_POINT('Ctrl Pts',(-1.06845992077163,-0.166511139289342,
1.28727233489076));
#23264=CARTESIAN_POINT('Ctrl Pts',(-1.10004620708042,-0.174823883464314,
1.25478273943443));
#23265=CARTESIAN_POINT('Ctrl Pts',(-1.12726776497764,-0.172667519342168,
1.22829923781242));
#23266=CARTESIAN_POINT('Ctrl Pts',(-1.1865727843456,-0.154814727716306,
1.17205963503352));
#23267=CARTESIAN_POINT('Ctrl Pts',(-1.21953445537447,-0.140474145488659,
1.14130666672565));
#23268=CARTESIAN_POINT('Ctrl Pts',(-1.25585067703094,-0.117749801015222,
1.10727038327973));
#23269=CARTESIAN_POINT('Ctrl Pts',(-1.06845992077163,-0.166511139289342,
1.28727233489076));
#23270=CARTESIAN_POINT('Ctrl Pts',(-1.16282366323453,-0.203229920731113,
1.39987124007464));
#23271=CARTESIAN_POINT('Ctrl Pts',(-1.23859785430383,-0.259800859583567,
1.50346488650363));
#23272=CARTESIAN_POINT('Ctrl Pts',(-1.36677481743678,-0.431100013478375,
1.715480776583));
#23273=CARTESIAN_POINT('Ctrl Pts',(-1.40911659430226,-0.556572568507924,
1.81902921434248));
#23274=CARTESIAN_POINT('Ctrl Pts',(-1.42280782457595,-0.712641620935351,
1.90869858745619));
#23275=CARTESIAN_POINT('Ctrl Pts',(-1.25585067703094,-0.117749801015222,
1.10727038327973));
#23276=CARTESIAN_POINT('Ctrl Pts',(-1.33766656151263,-0.145300304395601,
1.18103565901045));
#23277=CARTESIAN_POINT('Ctrl Pts',(-1.41595401455119,-0.186548988329719,
1.25302429310891));
#23278=CARTESIAN_POINT('Ctrl Pts',(-1.55687787546593,-0.308693492339175,
1.3926078838988));
#23279=CARTESIAN_POINT('Ctrl Pts',(-1.61436582414943,-0.387630019962956,
1.45574709063863));
#23280=CARTESIAN_POINT('Ctrl Pts',(-1.68758071271377,-0.556523222076088,
1.5589570108259));
#23281=CARTESIAN_POINT('Ctrl Pts',(-1.70827005906903,-0.63654174132047,
1.59904902099411));
#23282=CARTESIAN_POINT('Ctrl Pts',(-1.71930883511106,-0.71964734468187,
1.63615580822897));
#23283=CARTESIAN_POINT('Ctrl Pts',(-1.19577051030242,-0.420870970491663,
1.1015723109602));
#23284=CARTESIAN_POINT('Ctrl Pts',(-1.425339146688,-0.561530328976118,1.31988785480615));
#23285=CARTESIAN_POINT('Ctrl Pts',(-1.52384297854319,-0.798478145979653,
1.4989096332868));
#23286=CARTESIAN_POINT('Ctrl Pts',(-1.49128200586798,-1.13171442150227,
1.63863764640214));
#23287=CARTESIAN_POINT('Ctrl Pts',(-1.17679362500493,-0.393355414961737,
1.12589971949673));
#23288=CARTESIAN_POINT('Ctrl Pts',(-1.40368256628313,-0.527463617924696,
1.34900830339198));
#23289=CARTESIAN_POINT('Ctrl Pts',(-1.50373022520315,-0.757891527007919,
1.53195557707745));
#23290=CARTESIAN_POINT('Ctrl Pts',(-1.47705841783301,-1.08455939173712,
1.67474624941239));
#23291=CARTESIAN_POINT('Ctrl Pts',(-1.14284817765566,-0.352262141476105,
1.16769296545954));
#23292=CARTESIAN_POINT('Ctrl Pts',(-1.3645632700682,-0.476355861470114,
1.39903566442693));
#23293=CARTESIAN_POINT('Ctrl Pts',(-1.46622517664402,-0.696074558068199,
1.588783597768));
#23294=CARTESIAN_POINT('Ctrl Pts',(-1.44794881615931,-1.01150165877894,
1.73684050274471));
#23295=CARTESIAN_POINT('Ctrl Pts',(-1.09051150146367,-0.308178085105591,
1.22804267083047));
#23296=CARTESIAN_POINT('Ctrl Pts',(-1.30325409768322,-0.42072513805346,
1.47142154083509));
#23297=CARTESIAN_POINT('Ctrl Pts',(-1.40449154295596,-0.626556636662154,
1.6709985296405));
#23298=CARTESIAN_POINT('Ctrl Pts',(-1.39421997501402,-0.925684985930717,
1.82676723342071));
#23299=CARTESIAN_POINT('Ctrl Pts',(-1.05685857441837,-0.295454942931511,
1.2635364344865));
#23300=CARTESIAN_POINT('Ctrl Pts',(-1.26316084408196,-0.403825079433306,
1.51398418220584));
#23301=CARTESIAN_POINT('Ctrl Pts',(-1.36162184430235,-0.602771168700631,
1.71946457116169));
#23302=CARTESIAN_POINT('Ctrl Pts',(-1.35249734632791,-0.892463171324795,
1.87977332297459));
#23303=CARTESIAN_POINT('Ctrl Pts',(-1.03743092373275,-0.292083537908477,
1.28318517919043));
#23304=CARTESIAN_POINT('Ctrl Pts',(-1.23982087453715,-0.398906250549902,
1.53754499301448));
#23305=CARTESIAN_POINT('Ctrl Pts',(-1.33626197576336,-0.594546582101055,
1.74612783237292));
#23306=CARTESIAN_POINT('Ctrl Pts',(-1.32675422741137,-0.879004532561935,
1.90893369726574));
#23307=CARTESIAN_POINT('',(-1.04067701160391,-0.293809324770207,1.28727233489076));
#23308=CARTESIAN_POINT('Ctrl Pts',(-1.19131159212569,-0.414490807021284,
1.10727038327973));
#23309=CARTESIAN_POINT('Ctrl Pts',(-1.1767690131419,-0.393158028076673,
1.12801545944032));
#23310=CARTESIAN_POINT('Ctrl Pts',(-1.1594596657054,-0.371002680489135,
1.15133239961409));
#23311=CARTESIAN_POINT('Ctrl Pts',(-1.12447870759388,-0.335895470715412,
1.19509600545484));
#23312=CARTESIAN_POINT('Ctrl Pts',(-1.10930988332438,-0.323050675538543,
1.21324740617428));
#23313=CARTESIAN_POINT('Ctrl Pts',(-1.08088339992866,-0.305600782276628,
1.24538218411116));
#23314=CARTESIAN_POINT('Ctrl Pts',(-1.06407548086623,-0.297892884779764,
1.26364457695028));
#23315=CARTESIAN_POINT('Ctrl Pts',(-1.04067701160391,-0.293809324770207,
1.28727233489076));
#23316=CARTESIAN_POINT('Ctrl Pts',(-1.04067701160391,-0.293809324770207,
1.28727233489076));
#23317=CARTESIAN_POINT('Ctrl Pts',(-1.12993947443311,-0.341610972564374,
1.39987124007464));
#23318=CARTESIAN_POINT('Ctrl Pts',(-1.19835965101752,-0.406884846288962,
1.50346488650363));
#23319=CARTESIAN_POINT('Ctrl Pts',(-1.30500348982786,-0.592356746173702,
1.715480776583));
#23320=CARTESIAN_POINT('Ctrl Pts',(-1.33194693676576,-0.722011051157661,
1.81902921434248));
#23321=CARTESIAN_POINT('Ctrl Pts',(-1.32676788217082,-0.878593860895847,
1.90869858745619));
#23322=CARTESIAN_POINT('Ctrl Pts',(-1.04067701160391,-0.293809324770207,
1.28727233489076));
#23323=CARTESIAN_POINT('Ctrl Pts',(-1.24137728305361,-0.40128791525442,
1.54044292999952));
#23324=CARTESIAN_POINT('Ctrl Pts',(-1.3367108140079,-0.59709613876759,1.74808806061869));
#23325=CARTESIAN_POINT('Ctrl Pts',(-1.32667760446677,-0.881233995309716,
1.91020772674828));
#23326=CARTESIAN_POINT('Ctrl Pts',(-1.04993798132648,-0.251376596276585,
1.28727233489076));
#23327=CARTESIAN_POINT('Ctrl Pts',(-1.25446154039629,-0.35054884232117,
1.54044292999951));
#23328=CARTESIAN_POINT('Ctrl Pts',(-1.35741454085596,-0.542061247874906,
1.74808806061869));
#23329=CARTESIAN_POINT('Ctrl Pts',(-1.3587969827055,-0.825913812937791,
1.91020772674828));
#23330=CARTESIAN_POINT('Ctrl Pts',(-1.05919895104906,-0.208943867782964,
1.28727233489076));
#23331=CARTESIAN_POINT('Ctrl Pts',(-1.26754579773896,-0.29980976938792,
1.54044292999952));
#23332=CARTESIAN_POINT('Ctrl Pts',(-1.37811826770402,-0.487026356982221,
1.74808806061869));
#23333=CARTESIAN_POINT('Ctrl Pts',(-1.39091636094422,-0.770593630565867,
1.91020772674828));
#23334=CARTESIAN_POINT('Ctrl Pts',(-1.06845992077163,-0.166511139289342,
1.28727233489076));
#23335=CARTESIAN_POINT('Ctrl Pts',(-1.28063005508163,-0.24907069645467,
1.54044292999952));
#23336=CARTESIAN_POINT('Ctrl Pts',(-1.39882199455207,-0.431991466089537,
1.74808806061869));
#23337=CARTESIAN_POINT('Ctrl Pts',(-1.42303573918295,-0.715273448193942,
1.91020772674828));
#23338=CARTESIAN_POINT('Ctrl Pts',(-1.04067701160391,-0.293809324770207,
1.28727233489076));
#23339=CARTESIAN_POINT('Ctrl Pts',(-1.04588229398058,-0.272797358647497,
1.28797191329047));
#23340=CARTESIAN_POINT('Ctrl Pts',(-1.05079925066492,-0.251713870469972,
1.28831907556383));
#23341=CARTESIAN_POINT('Ctrl Pts',(-1.05542144523633,-0.230554570986284,
1.288319084765));
#23342=CARTESIAN_POINT('Ctrl Pts',(-1.06007256258898,-0.209262869938621,
1.28831909402374));
#23343=CARTESIAN_POINT('Ctrl Pts',(-1.06442048323407,-0.187915901626914,
1.28796761487395));
#23344=CARTESIAN_POINT('Ctrl Pts',(-1.06845992077163,-0.166511139289342,
1.28727233489076));
#23345=CARTESIAN_POINT('Origin',(0.,0.,1.37171309575435));
#23346=CARTESIAN_POINT('',(-1.26108935601086,-0.0260686553993158,1.10727038327973));
#23347=CARTESIAN_POINT('Ctrl Pts',(-1.76386916735272,-0.602229799711917,
1.63615580822897));
#23348=CARTESIAN_POINT('Ctrl Pts',(-1.74092498377312,-0.497389884696873,
1.58735805514594));
#23349=CARTESIAN_POINT('Ctrl Pts',(-1.70624968855518,-0.406388294299067,
1.53858095020821));
#23350=CARTESIAN_POINT('Ctrl Pts',(-1.61071325107042,-0.240766166368963,
1.42806953503212));
#23351=CARTESIAN_POINT('Ctrl Pts',(-1.54601110868788,-0.16897713225799,
1.3646130604457));
#23352=CARTESIAN_POINT('Ctrl Pts',(-1.40397010717825,-0.0713877673286483,
1.23357020765531));
#23353=CARTESIAN_POINT('Ctrl Pts',(-1.33378082531076,-0.0423971966252641,
1.17136442658356));
#23354=CARTESIAN_POINT('Ctrl Pts',(-1.26108935601086,-0.0260686553993154,
1.10727038327973));
#23355=CARTESIAN_POINT('Origin',(0.,0.,1.10727038327973));
#23356=CARTESIAN_POINT('Ctrl Pts',(-1.06394999323939,0.172008888562255,
1.28318567027397));
#23357=CARTESIAN_POINT('Ctrl Pts',(-1.2924681694826,0.160362439116273,1.53750521640541));
#23358=CARTESIAN_POINT('Ctrl Pts',(-1.46231719972918,0.023577760251311,
1.74606225962531));
#23359=CARTESIAN_POINT('Ctrl Pts',(-1.57349708397913,-0.23834514803263,
1.90885679993368));
#23360=CARTESIAN_POINT('Ctrl Pts',(-1.07868665224636,0.172859187306825,
1.2684765050474));
#23361=CARTESIAN_POINT('Ctrl Pts',(-1.31032224774096,0.160753683145647,
1.51986749395221));
#23362=CARTESIAN_POINT('Ctrl Pts',(-1.48218332835239,0.0218713714335428,
1.72610289246663));
#23363=CARTESIAN_POINT('Ctrl Pts',(-1.59454606057878,-0.243802874063091,
1.88702805548521));
#23364=CARTESIAN_POINT('Ctrl Pts',(-1.10570688269945,0.177804687773572,
1.24116976953013));
#23365=CARTESIAN_POINT('Ctrl Pts',(-1.34316347164223,0.16550438356704,1.48715026946299));
#23366=CARTESIAN_POINT('Ctrl Pts',(-1.51954478212276,0.0232152493262158,
1.6888660924649));
#23367=CARTESIAN_POINT('Ctrl Pts',(-1.63485294054343,-0.249054092840228,
1.8463203415307));
#23368=CARTESIAN_POINT('Ctrl Pts',(-1.16355954955659,0.208466906889382,
1.18070453025514));
#23369=CARTESIAN_POINT('Ctrl Pts',(-1.41450709648088,0.200040954183215,
1.41458088343679));
#23370=CARTESIAN_POINT('Ctrl Pts',(-1.60338349810865,0.0532384711777712,
1.60640735029516));
#23371=CARTESIAN_POINT('Ctrl Pts',(-1.73033051533549,-0.231963472934464,
1.75609715466375));
#23372=CARTESIAN_POINT('Ctrl Pts',(-1.20636749722078,0.248125754775118,
1.13427327868627));
#23373=CARTESIAN_POINT('Ctrl Pts',(-1.46793051395096,0.246072078233562,
1.35898312394782));
#23374=CARTESIAN_POINT('Ctrl Pts',(-1.66851465914541,0.0981648464084902,
1.54327941073122));
#23375=CARTESIAN_POINT('Ctrl Pts',(-1.80834818125255,-0.195461051586317,
1.68710688538769));
#23376=CARTESIAN_POINT('Ctrl Pts',(-1.235641855012,0.281595159362692,1.10188938448118));
#23377=CARTESIAN_POINT('Ctrl Pts',(-1.50471757474417,0.285104353628414,
1.32023273220194));
#23378=CARTESIAN_POINT('Ctrl Pts',(-1.71433282083683,0.137346783688562,
1.49928348142626));
#23379=CARTESIAN_POINT('Ctrl Pts',(-1.86448759328998,-0.161677550456861,
1.63904163215416));
#23380=CARTESIAN_POINT('',(-1.06762054184321,0.171810769270086,1.28727233489076));
#23381=CARTESIAN_POINT('',(-1.23077165948193,0.27609248605186,1.10727038327973));
#23382=CARTESIAN_POINT('Ctrl Pts',(-1.06762054184321,0.171810769270086,
1.28727233489076));
#23383=CARTESIAN_POINT('Ctrl Pts',(-1.10022966448203,0.173665579012753,
1.25478273943509));
#23384=CARTESIAN_POINT('Ctrl Pts',(-1.12545255134418,0.184128327165882,
1.22829923781306));
#23385=CARTESIAN_POINT('Ctrl Pts',(-1.17633816045214,0.219433599811068,
1.17205963503584));
#23386=CARTESIAN_POINT('Ctrl Pts',(-1.20325508885488,0.243258020496417,
1.14130666672783));
#23387=CARTESIAN_POINT('Ctrl Pts',(-1.23077165948193,0.27609248605186,1.10727038327973));
#23388=CARTESIAN_POINT('Ctrl Pts',(-1.06762054184321,0.171810769270086,
1.28727233489076));
#23389=CARTESIAN_POINT('Ctrl Pts',(-1.16871252149279,0.166049132983329,
1.39987124007464));
#23390=CARTESIAN_POINT('Ctrl Pts',(-1.2582594411694,0.135662485730195,1.50346488650363));
#23391=CARTESIAN_POINT('Ctrl Pts',(-1.43309732687145,0.0123561690781441,
1.715480776583));
#23392=CARTESIAN_POINT('Ctrl Pts',(-1.51213990150266,-0.0938909933754469,
1.81902921434248));
#23393=CARTESIAN_POINT('Ctrl Pts',(-1.57338902476662,-0.238090659850087,
1.90869858745619));
#23394=CARTESIAN_POINT('Ctrl Pts',(-1.23077165948193,0.27609248605186,1.10727038327973));
#23395=CARTESIAN_POINT('Ctrl Pts',(-1.31709676330278,0.275172898999399,
1.18103565901041));
#23396=CARTESIAN_POINT('Ctrl Pts',(-1.40429909999044,0.260135222790514,
1.25302429310884));
#23397=CARTESIAN_POINT('Ctrl Pts',(-1.57122974978687,0.189563202796485,
1.38867432147861));
#23398=CARTESIAN_POINT('Ctrl Pts',(-1.64657149028472,0.13638820421775,1.44891114041812));
#23399=CARTESIAN_POINT('Ctrl Pts',(-1.77077010917836,0.0017905112135637,
1.55340617058598));
#23400=CARTESIAN_POINT('Ctrl Pts',(-1.81883456875388,-0.0722162251277585,
1.59645518670946));
#23401=CARTESIAN_POINT('Ctrl Pts',(-1.85754313061971,-0.153129647965885,
1.63615580822897));
#23402=CARTESIAN_POINT('Ctrl Pts',(-1.26730161813771,-0.030758669949715,
1.1015723109602));
#23403=CARTESIAN_POINT('Ctrl Pts',(-1.52910049789878,-0.0935930593956264,
1.31988785480615));
#23404=CARTESIAN_POINT('Ctrl Pts',(-1.69600411129884,-0.28850446672445,
1.49890963328679));
#23405=CARTESIAN_POINT('Ctrl Pts',(-1.76801245833787,-0.615492891936185,
1.63863764640214));
#23406=CARTESIAN_POINT('Ctrl Pts',(-1.24075075344812,-0.0104540016207254,
1.12589971949672));
#23407=CARTESIAN_POINT('Ctrl Pts',(-1.49797667332671,-0.0678859432465771,
1.34900830339197));
#23408=CARTESIAN_POINT('Ctrl Pts',(-1.66433379116767,-0.256119480862738,
1.53195557707745));
#23409=CARTESIAN_POINT('Ctrl Pts',(-1.73991331668443,-0.575041124025744,
1.67474624941239));
#23410=CARTESIAN_POINT('Ctrl Pts',(-1.19576910668284,0.0181391694102173,
1.16769197379075));
#23411=CARTESIAN_POINT('Ctrl Pts',(-1.44497975845612,-0.0313672401565084,
1.39903467275814));
#23412=CARTESIAN_POINT('Ctrl Pts',(-1.60956344041244,-0.208916886053931,
1.58878224232));
#23413=CARTESIAN_POINT('Ctrl Pts',(-1.68965392328535,-0.514553591586066,
1.73683914729671));
#23414=CARTESIAN_POINT('Ctrl Pts',(-1.13237144427268,0.0438923944102214,
1.22804151155252));
#23415=CARTESIAN_POINT('Ctrl Pts',(-1.36948062872854,0.00259486397362416,
1.47142038155714));
#23416=CARTESIAN_POINT('Ctrl Pts',(-1.52936917527703,-0.161878639424908,
1.67099694623232));
#23417=CARTESIAN_POINT('Ctrl Pts',(-1.61203607707659,-0.449540694258328,
1.82676565001253));
#23418=CARTESIAN_POINT('Ctrl Pts',(-1.09643283244092,0.045592911399531,
1.2635364344865));
#23419=CARTESIAN_POINT('Ctrl Pts',(-1.32612616419274,0.00627769421187267,
1.51398418220585));
#23420=CARTESIAN_POINT('Ctrl Pts',(-1.48124586260133,-0.152505158025998,
1.71946457116169));
#23421=CARTESIAN_POINT('Ctrl Pts',(-1.56208770129018,-0.43083824977955,
1.87977332297459));
#23422=CARTESIAN_POINT('Ctrl Pts',(-1.07691421721301,0.0427958338931189,
1.28318517919043));
#23423=CARTESIAN_POINT('Ctrl Pts',(-1.30240853234962,0.00374333123643575,
1.53754499301448));
#23424=CARTESIAN_POINT('Ctrl Pts',(-1.45458565734394,-0.152519741700302,
1.74612783237292));
#23425=CARTESIAN_POINT('Ctrl Pts',(-1.53344559219597,-0.425993384917094,
1.90893369726574));
#23426=CARTESIAN_POINT('',(-1.22409607597286,-1.56082004234302E-11,1.14453307412866));
#23427=CARTESIAN_POINT('Ctrl Pts',(-1.26108935601086,-0.0260686553993156,
1.10727038327973));
#23428=CARTESIAN_POINT('Ctrl Pts',(-1.24961721838639,-0.0171963166387619,
1.1189234363026));
#23429=CARTESIAN_POINT('Ctrl Pts',(-1.23723544723125,-0.00835451937604592,
1.13139370287006));
#23430=CARTESIAN_POINT('Ctrl Pts',(-1.22409607597286,-3.12160393020622E-11,
1.14453307412866));
#23431=CARTESIAN_POINT('',(-1.08053472770428,0.042157609369957,1.28727233489076));
#23432=CARTESIAN_POINT('Ctrl Pts',(-1.08053472770428,0.0421576093699571,
1.28727233489076));
#23433=CARTESIAN_POINT('Ctrl Pts',(-1.18019989616608,0.024279158719655,
1.39987124007464));
#23434=CARTESIAN_POINT('Ctrl Pts',(-1.26544208722232,-0.0166569869072256,
1.50346488650363));
#23435=CARTESIAN_POINT('Ctrl Pts',(-1.42418037408903,-0.16009648734447,
1.715480776583));
#23436=CARTESIAN_POINT('Ctrl Pts',(-1.48987049850469,-0.275079075974332,
1.81902921434248));
#23437=CARTESIAN_POINT('Ctrl Pts',(-1.53333167412,-0.425598593400271,1.90869858745619));
#23438=CARTESIAN_POINT('Ctrl Pts',(-1.22409607597286,-3.12160393020622E-11,
1.14453307412866));
#23439=CARTESIAN_POINT('Ctrl Pts',(-1.21384438765874,0.00651841905088611,
1.15478476244295));
#23440=CARTESIAN_POINT('Ctrl Pts',(-1.20312882189276,0.0127305674258041,
1.16544721218023));
#23441=CARTESIAN_POINT('Ctrl Pts',(-1.17324021107686,0.0280274542414138,
1.19509600545493));
#23442=CARTESIAN_POINT('Ctrl Pts',(-1.15484454191168,0.0355561559109111,
1.21324740617458));
#23443=CARTESIAN_POINT('Ctrl Pts',(-1.12241703607502,0.0433677241466843,
1.24538218411131));
#23444=CARTESIAN_POINT('Ctrl Pts',(-1.10404988380787,0.0455044376575774,
1.26364457695047));
#23445=CARTESIAN_POINT('Ctrl Pts',(-1.08053472770428,0.0421576093699571,
1.28727233489076));
#23446=CARTESIAN_POINT('Ctrl Pts',(-1.08053472770428,0.0421576093699571,
1.28727233489076));
#23447=CARTESIAN_POINT('Ctrl Pts',(-1.30462473967982,0.00195919018135112,
1.54044292999951));
#23448=CARTESIAN_POINT('Ctrl Pts',(-1.45580038421926,-0.154805815536382,
1.74808806061869));
#23449=CARTESIAN_POINT('Ctrl Pts',(-1.5340616613226,-0.428137407783241,
1.91020772674828));
#23450=CARTESIAN_POINT('Ctrl Pts',(-1.07622999908393,0.0853753293366668,
1.28727233489076));
#23451=CARTESIAN_POINT('Ctrl Pts',(-1.30138937207125,0.0542581740029554,
1.54044292999951));
#23452=CARTESIAN_POINT('Ctrl Pts',(-1.45848408198029,-0.0960667204863548,
1.74808806061869));
#23453=CARTESIAN_POINT('Ctrl Pts',(-1.54751412881105,-0.365599354131263,
1.91020772674828));
#23454=CARTESIAN_POINT('Ctrl Pts',(-1.07192527046357,0.128593049303376,
1.28727233489076));
#23455=CARTESIAN_POINT('Ctrl Pts',(-1.29815400446268,0.10655715782456,1.54044292999952));
#23456=CARTESIAN_POINT('Ctrl Pts',(-1.46116777974132,-0.0373276254363268,
1.74808806061869));
#23457=CARTESIAN_POINT('Ctrl Pts',(-1.56096659629949,-0.303061300479284,
1.91020772674828));
#23458=CARTESIAN_POINT('Ctrl Pts',(-1.06762054184321,0.171810769270086,
1.28727233489076));
#23459=CARTESIAN_POINT('Ctrl Pts',(-1.29491863685411,0.158856141646164,
1.54044292999951));
#23460=CARTESIAN_POINT('Ctrl Pts',(-1.46385147750235,0.0214114696136999,
1.74808806061869));
#23461=CARTESIAN_POINT('Ctrl Pts',(-1.57441906378793,-0.240523246827305,
1.91020772674828));
#23462=CARTESIAN_POINT('Ctrl Pts',(-1.08053472770428,0.0421576093699571,
1.28727233489076));
#23463=CARTESIAN_POINT('Ctrl Pts',(-1.07899219081063,0.0637496973860188,
1.28797191329046));
#23464=CARTESIAN_POINT('Ctrl Pts',(-1.07715333835806,0.0853207093795665,
1.28831907556383));
#23465=CARTESIAN_POINT('Ctrl Pts',(-1.07501072349525,0.106872735707655,
1.288319084765));
#23466=CARTESIAN_POINT('Ctrl Pts',(-1.07285470149866,0.128559621036833,
1.28831909402374));
#23467=CARTESIAN_POINT('Ctrl Pts',(-1.07039324377381,0.150205375722343,
1.28796761487395));
#23468=CARTESIAN_POINT('Ctrl Pts',(-1.06762054184321,0.171810769270086,
1.28727233489076));
#23469=CARTESIAN_POINT('Origin',(0.,0.,1.37171309575435));
#23470=CARTESIAN_POINT('',(-1.20742290720348,0.36490527784414,1.10727038327973));
#23471=CARTESIAN_POINT('Ctrl Pts',(-1.86363850813291,-0.0276890267571663,
1.63615580822897));
#23472=CARTESIAN_POINT('Ctrl Pts',(-1.80655480211394,0.069823936699024,
1.5847793405578));
#23473=CARTESIAN_POINT('Ctrl Pts',(-1.74187241700952,0.148691945288576,
1.5334368554465));
#23474=CARTESIAN_POINT('Ctrl Pts',(-1.59669345888591,0.274785130849269,
1.4207678259124));
#23475=CARTESIAN_POINT('Ctrl Pts',(-1.51444831269986,0.320436333138579,
1.35830292226018));
#23476=CARTESIAN_POINT('Ctrl Pts',(-1.35321270714142,0.366271065016131,
1.23020598103184));
#23477=CARTESIAN_POINT('Ctrl Pts',(-1.2795761902763,0.371649422530894,1.1696137009149));
#23478=CARTESIAN_POINT('Ctrl Pts',(-1.20742290720348,0.364905277844141,
1.10727038327973));
#23479=CARTESIAN_POINT('Origin',(0.,0.,1.10727038327973));
#23480=CARTESIAN_POINT('Ctrl Pts',(-0.958722904333223,0.492368803403902,
1.28318567027397));
#23481=CARTESIAN_POINT('Ctrl Pts',(-1.17966054547972,0.551909716442827,
1.53751096017971));
#23482=CARTESIAN_POINT('Ctrl Pts',(-1.38346957888851,0.474301142999538,
1.74607168007007));
#23483=CARTESIAN_POINT('Ctrl Pts',(-1.57015000455958,0.259543083074033,
1.90886782994505));
#23484=CARTESIAN_POINT('Ctrl Pts',(-0.972472836356931,0.497730308181424,
1.26847940010162));
#23485=CARTESIAN_POINT('Ctrl Pts',(-1.196516618136,0.557797896845799,1.51987665322458));
#23486=CARTESIAN_POINT('Ctrl Pts',(-1.40288697684033,0.478816264707968,
1.72611612827484));
#23487=CARTESIAN_POINT('Ctrl Pts',(-1.59185117960571,0.260856494176603,
1.88704325648016));
#23488=CARTESIAN_POINT('Ctrl Pts',(-0.996638068239392,0.510779460904229,
1.24117819097188));
#23489=CARTESIAN_POINT('Ctrl Pts',(-1.22627731830139,0.572460097309862,
1.48716579746039));
#23490=CARTESIAN_POINT('Ctrl Pts',(-1.43799804358595,0.491635127338186,
1.68888670640878));
#23491=CARTESIAN_POINT('Ctrl Pts',(-1.63180052564183,0.268313724592159,
1.84634350908918));
#23492=CARTESIAN_POINT('Ctrl Pts',(-1.04217697649275,0.557803663431838,
1.18072535874296));
#23493=CARTESIAN_POINT('Ctrl Pts',(-1.28344787385866,0.62733559714006,1.41461088358276));
#23494=CARTESIAN_POINT('Ctrl Pts',(-1.50844372983685,0.546077997260112,
1.60644436926605));
#23495=CARTESIAN_POINT('Ctrl Pts',(-1.71730828939987,0.314053900652125,
1.75613814413928));
#23496=CARTESIAN_POINT('Ctrl Pts',(-1.07063174084474,0.608738508149426,
1.13430117558029));
#23497=CARTESIAN_POINT('Ctrl Pts',(-1.32002833380447,0.687608854742561,
1.35902160674437));
#23498=CARTESIAN_POINT('Ctrl Pts',(-1.55649910176849,0.608917570976486,
1.54332567193681));
#23499=CARTESIAN_POINT('Ctrl Pts',(-1.78021953810235,0.372863601758235,
1.68715809360677));
#23500=CARTESIAN_POINT('Ctrl Pts',(-1.08812946536139,0.649605006049397,
1.10192284729582));
#23501=CARTESIAN_POINT('Ctrl Pts',(-1.34295142581462,0.736085457637467,
1.32027771712106));
#23502=CARTESIAN_POINT('Ctrl Pts',(-1.58796351671871,0.660325994321482,
1.49933702411959));
#23503=CARTESIAN_POINT('Ctrl Pts',(-1.82316573807367,0.42232661610144,1.63910076829143));
#23504=CARTESIAN_POINT('',(-0.962275025729455,0.493314642657339,1.28727233489076));
#23505=CARTESIAN_POINT('',(-1.08521613661244,0.642908916934723,1.10727038327973));
#23506=CARTESIAN_POINT('Ctrl Pts',(-0.962275025729456,0.493314642657339,
1.28727233489076));
#23507=CARTESIAN_POINT('Ctrl Pts',(-0.992714976574408,0.505155444616818,
1.25478273943461));
#23508=CARTESIAN_POINT('Ctrl Pts',(-1.0134702004971,0.522900410114029,1.22829923781261));
#23509=CARTESIAN_POINT('Ctrl Pts',(-1.0509553613873,0.572202237707381,1.17205963503414));
#23510=CARTESIAN_POINT('Ctrl Pts',(-1.0691927306701,0.603178396560383,1.14130666672619));
#23511=CARTESIAN_POINT('Ctrl Pts',(-1.08521613661244,0.642908916934723,
1.10727038327973));
#23512=CARTESIAN_POINT('Ctrl Pts',(-0.962275025729455,0.493314642657339,
1.28727233489076));
#23513=CARTESIAN_POINT('Ctrl Pts',(-1.06019965524839,0.519074140629024,
1.39987124007464));
#23514=CARTESIAN_POINT('Ctrl Pts',(-1.15475382712427,0.517846241724568,
1.50346488650363));
#23515=CARTESIAN_POINT('Ctrl Pts',(-1.35913828497575,0.454602843714802,
1.715480776583));
#23516=CARTESIAN_POINT('Ctrl Pts',(-1.46714441944577,0.377981286365637,
1.81902921434248));
#23517=CARTESIAN_POINT('Ctrl Pts',(-1.5699559447672,0.259766273896474,1.90869858745619));
#23518=CARTESIAN_POINT('Ctrl Pts',(-1.08521613661244,0.642908916934723,
1.10727038327973));
#23519=CARTESIAN_POINT('Ctrl Pts',(-1.16760035714812,0.668710261798002,
1.18103565901041));
#23520=CARTESIAN_POINT('Ctrl Pts',(-1.25518160519554,0.6813555858353,1.25302429310884));
#23521=CARTESIAN_POINT('Ctrl Pts',(-1.44098614169379,0.665371573464,1.3926078838987));
#23522=CARTESIAN_POINT('Ctrl Pts',(-1.53389259595494,0.635301149560143,
1.45574709063854));
#23523=CARTESIAN_POINT('Ctrl Pts',(-1.69239761845936,0.541698310562581,
1.55895701082585));
#23524=CARTESIAN_POINT('Ctrl Pts',(-1.75616935678545,0.489122861296321,
1.59904902099409));
#23525=CARTESIAN_POINT('Ctrl Pts',(-1.81394816223928,0.428377445609995,
1.63615580822897));
#23526=CARTESIAN_POINT('Ctrl Pts',(-1.21487793679797,0.362330138275323,
1.10149705943221));
#23527=CARTESIAN_POINT('Ctrl Pts',(-1.48329895916361,0.383459937582892,
1.31979778023781));
#23528=CARTESIAN_POINT('Ctrl Pts',(-1.70227260218965,0.249644960941919,
1.49880741124996));
#23529=CARTESIAN_POINT('Ctrl Pts',(-1.8717988658761,-0.0391147916475981,
1.63852595246866));
#23530=CARTESIAN_POINT('Ctrl Pts',(-1.18333690797345,0.373447482460584,
1.12583385309083));
#23531=CARTESIAN_POINT('Ctrl Pts',(-1.44573672483851,0.398305182537798,
1.34892944774501));
#23532=CARTESIAN_POINT('Ctrl Pts',(-1.66212671668266,0.270675994878907,
1.53186602370529));
#23533=CARTESIAN_POINT('Ctrl Pts',(-1.83255854794258,-0.00930365130124231,
1.6746483889292));
#23534=CARTESIAN_POINT('Ctrl Pts',(-1.13169790455625,0.386758017000774,
1.16764044916317));
#23535=CARTESIAN_POINT('Ctrl Pts',(-1.38402127269754,0.416680587119741,
1.39897336709084));
#23536=CARTESIAN_POINT('Ctrl Pts',(-1.59542335194443,0.29867037569466,1.58871211231351));
#23537=CARTESIAN_POINT('Ctrl Pts',(-1.76604232095016,0.0327265383253359,
1.7367627568762));
#23538=CARTESIAN_POINT('Ctrl Pts',(-1.06341115236231,0.391671741837562,
1.22801607619329));
#23539=CARTESIAN_POINT('Ctrl Pts',(-1.30168216224368,0.425665904909548,
1.47139032317726));
#23540=CARTESIAN_POINT('Ctrl Pts',(-1.50457544636212,0.318647566754323,
1.67096220367118));
#23541=CARTESIAN_POINT('Ctrl Pts',(-1.67209124376878,0.0706042875438534,
1.82672793765152));
#23542=CARTESIAN_POINT('Ctrl Pts',(-1.0286884268729,0.38218165487343,1.263527751515));
#23543=CARTESIAN_POINT('Ctrl Pts',(-1.25929056133868,0.415770412604395,
1.51397381108001));
#23544=CARTESIAN_POINT('Ctrl Pts',(-1.45588630034145,0.312692596804324,
1.71945276482243));
#23545=CARTESIAN_POINT('Ctrl Pts',(-1.61878272768801,0.0729619965738858,
1.8797604367197));
#23546=CARTESIAN_POINT('Ctrl Pts',(-1.01098164381094,0.373486051297297,
1.28318517919159));
#23547=CARTESIAN_POINT('Ctrl Pts',(-1.23750736860246,0.40602648967972,1.53754499301511));
#23548=CARTESIAN_POINT('Ctrl Pts',(-1.43052436008972,0.304436793685257,
1.74612783237315));
#23549=CARTESIAN_POINT('Ctrl Pts',(-1.59003261827273,0.0687169633139079,
1.90893369726572));
#23550=CARTESIAN_POINT('',(-1.01462217612883,0.373997862975654,1.28727233489076));
#23551=CARTESIAN_POINT('Ctrl Pts',(-1.20742290720348,0.364905277844141,
1.10727038327973));
#23552=CARTESIAN_POINT('Ctrl Pts',(-1.18311862080923,0.3736159450907,1.12801545944054));
#23553=CARTESIAN_POINT('Ctrl Pts',(-1.15609247800018,0.381365818655266,
1.15133239961433));
#23554=CARTESIAN_POINT('Ctrl Pts',(-1.10715678825378,0.389206856698375,
1.19509600545556));
#23555=CARTESIAN_POINT('Ctrl Pts',(-1.08733497046134,0.390682503085297,
1.2132474061751));
#23556=CARTESIAN_POINT('Ctrl Pts',(-1.05408067239149,0.388091095569761,
1.24538218411098));
#23557=CARTESIAN_POINT('Ctrl Pts',(-1.03595219175499,0.38444746868904,1.26364457695016));
#23558=CARTESIAN_POINT('Ctrl Pts',(-1.01462217612883,0.373997862975654,
1.28727233489076));
#23559=CARTESIAN_POINT('Ctrl Pts',(-1.01462217612883,0.373997862975654,
1.28727233489076));
#23560=CARTESIAN_POINT('Ctrl Pts',(-1.11493412912611,0.387792676785359,
1.39987124007464));
#23561=CARTESIAN_POINT('Ctrl Pts',(-1.20865423507634,0.375201374409042,
1.50346488650363));
#23562=CARTESIAN_POINT('Ctrl Pts',(-1.40394856048621,0.287835131123856,
1.715480776583));
#23563=CARTESIAN_POINT('Ctrl Pts',(-1.50195515531182,0.198779555753984,
1.81902921434248));
#23564=CARTESIAN_POINT('Ctrl Pts',(-1.58980227845634,0.0690572297370887,
1.90869858745619));
#23565=CARTESIAN_POINT('Ctrl Pts',(-1.01462217612883,0.373997862975653,
1.28727233489076));
#23566=CARTESIAN_POINT('Ctrl Pts',(-1.24016643693111,0.405014516431691,
1.54044292999952));
#23567=CARTESIAN_POINT('Ctrl Pts',(-1.43238606966553,0.302637979515068,
1.74808806061869));
#23568=CARTESIAN_POINT('Ctrl Pts',(-1.59128107433209,0.0668682522257823,
1.91020772674828));
#23569=CARTESIAN_POINT('Ctrl Pts',(-0.997173125995706,0.413770122869549,
1.28727233489076));
#23570=CARTESIAN_POINT('Ctrl Pts',(-1.22092814469495,0.453754022216744,
1.54044292999952));
#23571=CARTESIAN_POINT('Ctrl Pts',(-1.41678703930426,0.3593314868396,1.74808806061869));
#23572=CARTESIAN_POINT('Ctrl Pts',(-1.58474980982363,0.130502516738118,
1.91020772674828));
#23573=CARTESIAN_POINT('Ctrl Pts',(-0.979724075862581,0.453542382763444,
1.28727233489076));
#23574=CARTESIAN_POINT('Ctrl Pts',(-1.2016898524588,0.502493528001797,1.54044292999952));
#23575=CARTESIAN_POINT('Ctrl Pts',(-1.40118800894299,0.416024994164134,
1.74808806061869));
#23576=CARTESIAN_POINT('Ctrl Pts',(-1.57821854531517,0.194136781250453,
1.91020772674828));
#23577=CARTESIAN_POINT('Ctrl Pts',(-0.962275025729455,0.493314642657339,
1.28727233489076));
#23578=CARTESIAN_POINT('Ctrl Pts',(-1.18245156022264,0.55123303378685,1.54044292999952));
#23579=CARTESIAN_POINT('Ctrl Pts',(-1.38558897858172,0.472718501488667,
1.74808806061869));
#23580=CARTESIAN_POINT('Ctrl Pts',(-1.5716872808067,0.257771045762789,1.91020772674828));
#23581=CARTESIAN_POINT('Ctrl Pts',(-1.01462217612883,0.373997862975654,
1.28727233489076));
#23582=CARTESIAN_POINT('Ctrl Pts',(-1.00648281422349,0.394056488869176,
1.28797191329047));
#23583=CARTESIAN_POINT('Ctrl Pts',(-0.998068152324093,0.414003503730718,
1.28831907556383));
#23584=CARTESIAN_POINT('Ctrl Pts',(-0.989370462098314,0.433838594404394,
1.288319084765));
#23585=CARTESIAN_POINT('Ctrl Pts',(-0.980618347207407,0.453797800577666,
1.28831909402374));
#23586=CARTESIAN_POINT('Ctrl Pts',(-0.971588455744705,0.473623504353535,
1.28796761487395));
#23587=CARTESIAN_POINT('Ctrl Pts',(-0.962275025729455,0.493314642657339,
1.28727233489076));
#23588=CARTESIAN_POINT('Origin',(0.,0.,1.37171309575435));
#23589=CARTESIAN_POINT('',(-1.03556549162895,0.720159740047643,1.10727038327973));
#23590=CARTESIAN_POINT('Ctrl Pts',(-1.78098192700405,0.549562141057369,
1.63615580822897));
#23591=CARTESIAN_POINT('Ctrl Pts',(-1.70079633666886,0.620893161259203,
1.58735805514606));
#23592=CARTESIAN_POINT('Ctrl Pts',(-1.61925404078159,0.67413336725827,1.53858095020834));
#23593=CARTESIAN_POINT('Ctrl Pts',(-1.44461319502359,0.751969574388254,
1.42806953503213));
#23594=CARTESIAN_POINT('Ctrl Pts',(-1.35007152673689,0.772017157909612,
1.36461306044571));
#23595=CARTESIAN_POINT('Ctrl Pts',(-1.1777963531315,0.7674790066995,1.23357020765531));
#23596=CARTESIAN_POINT('Ctrl Pts',(-1.10397180136272,0.749676646324454,
1.17136442658356));
#23597=CARTESIAN_POINT('Ctrl Pts',(-1.03556549162895,0.720159740047643,
1.10727038327973));
#23598=CARTESIAN_POINT('Origin',(0.,0.,1.10727038327973));
#23599=CARTESIAN_POINT('Ctrl Pts',(-0.759649337735664,0.764532229233201,
1.28318567027397));
#23600=CARTESIAN_POINT('Ctrl Pts',(-0.951374367053292,0.889432488376416,
1.53751096017971));
#23601=CARTESIAN_POINT('Ctrl Pts',(-1.16919064445971,0.87860280381325,1.74607168007007));
#23602=CARTESIAN_POINT('Ctrl Pts',(-1.41309816995491,0.732043175543704,
1.90886782994505));
#23603=CARTESIAN_POINT('Ctrl Pts',(-0.771069504093749,0.773880285955837,
1.26847940010162));
#23604=CARTESIAN_POINT('Ctrl Pts',(-0.965585896981724,0.900241293626992,
1.51987665322458));
#23605=CARTESIAN_POINT('Ctrl Pts',(-1.18626243797171,0.888897245689575,
1.72611612827484));
#23606=CARTESIAN_POINT('Ctrl Pts',(-1.43333134754249,0.739998335618538,
1.88704325648016));
#23607=CARTESIAN_POINT('Ctrl Pts',(-0.790019380359266,0.793756470105417,
1.24117952306876));
#23608=CARTESIAN_POINT('Ctrl Pts',(-0.989358920654663,0.923380672132903,
1.48716712955727));
#23609=CARTESIAN_POINT('Ctrl Pts',(-1.2156928538318,0.911936310735737,1.68888851879236));
#23610=CARTESIAN_POINT('Ctrl Pts',(-1.46902007592139,0.759433295933264,
1.84634532147277));
#23611=CARTESIAN_POINT('Ctrl Pts',(-0.818798433422957,0.852549487780084,
1.18072779772815));
#23612=CARTESIAN_POINT('Ctrl Pts',(-1.02677414338759,0.993235093958051,
1.41461332256795));
#23613=CARTESIAN_POINT('Ctrl Pts',(-1.26586652272339,0.985480669746802,
1.60644767971083));
#23614=CARTESIAN_POINT('Ctrl Pts',(-1.53620791207528,0.829355339157892,
1.75614145458406));
#23615=CARTESIAN_POINT('Ctrl Pts',(-0.830120749534189,0.909788127533561,
1.13430117558029));
#23616=CARTESIAN_POINT('Ctrl Pts',(-1.04293872696083,1.06186607016719,1.35902160674437));
#23617=CARTESIAN_POINT('Ctrl Pts',(-1.29215273573923,1.06009969793961,1.54332567193681));
#23618=CARTESIAN_POINT('Ctrl Pts',(-1.57786820262105,0.9047324491334,1.68715809360677));
#23619=CARTESIAN_POINT('Ctrl Pts',(-0.834133632104406,0.954061570898026,
1.10192284729582));
#23620=CARTESIAN_POINT('Ctrl Pts',(-1.04975978886662,1.115053684233,1.32027771712106));
#23621=CARTESIAN_POINT('Ctrl Pts',(-1.30619109614143,1.11871505289201,1.49933702411959));
#23622=CARTESIAN_POINT('Ctrl Pts',(-1.60342755392882,0.965045676875065,
1.63910076829143));
#23623=CARTESIAN_POINT('',(-0.762735325532963,0.766529441696069,1.28727233489076));
#23624=CARTESIAN_POINT('',(-0.833432097145889,0.946792943618196,1.10727038327973));
#23625=CARTESIAN_POINT('Ctrl Pts',(-0.762735325532963,0.766529441696069,
1.28727233489076));
#23626=CARTESIAN_POINT('Ctrl Pts',(-0.788026430107593,0.787197175677101,
1.25478273943417));
#23627=CARTESIAN_POINT('Ctrl Pts',(-0.80228232516309,0.810487357658964,
1.22829923781215));
#23628=CARTESIAN_POINT('Ctrl Pts',(-0.822697729112326,0.868959733810234,
1.17205963503243));
#23629=CARTESIAN_POINT('Ctrl Pts',(-0.830470338502341,0.90405546857811,
1.14130666672486));
#23630=CARTESIAN_POINT('Ctrl Pts',(-0.833432097145889,0.946792943618196,
1.10727038327973));
#23631=CARTESIAN_POINT('Ctrl Pts',(-0.762735325532963,0.766529441696069,
1.28727233489076));
#23632=CARTESIAN_POINT('Ctrl Pts',(-0.847907059902912,0.821288554787752,
1.39987124007464));
#23633=CARTESIAN_POINT('Ctrl Pts',(-0.938212862837218,0.849339599532016,
1.50346488650363));
#23634=CARTESIAN_POINT('Ctrl Pts',(-1.15213731807335,0.852349824604396,
1.715480776583));
#23635=CARTESIAN_POINT('Ctrl Pts',(-1.27853461941729,0.812854124246773,
1.81902921434248));
#23636=CARTESIAN_POINT('Ctrl Pts',(-1.41284463836769,0.732195474855993,
1.90869858745619));
#23637=CARTESIAN_POINT('Ctrl Pts',(-0.833432097145889,0.946792943618196,
1.10727038327973));
#23638=CARTESIAN_POINT('Ctrl Pts',(-0.903811092885819,0.996789604993491,
1.18103565901046));
#23639=CARTESIAN_POINT('Ctrl Pts',(-0.983198189519745,1.03588011685507,
1.25302429310894));
#23640=CARTESIAN_POINT('Ctrl Pts',(-1.16484813617473,1.07809517714268,1.39260788389885));
#23641=CARTESIAN_POINT('Ctrl Pts',(-1.26249969692003,1.07820617779494,1.45574709063867));
#23642=CARTESIAN_POINT('Ctrl Pts',(-1.44217179941028,1.03816533347019,1.55895701082593));
#23643=CARTESIAN_POINT('Ctrl Pts',(-1.51906903401087,1.00786966075199,1.59904902099412));
#23644=CARTESIAN_POINT('Ctrl Pts',(-1.59279130921887,0.967951970128402,
1.63615580822897));
#23645=CARTESIAN_POINT('Ctrl Pts',(-1.04334803864884,0.720016914634041,
1.1015723109602));
#23646=CARTESIAN_POINT('Ctrl Pts',(-1.29208090893698,0.823064346331375,
1.31988785480615));
#23647=CARTESIAN_POINT('Ctrl Pts',(-1.54167481933166,0.763481187915701,
1.4989096332868));
#23648=CARTESIAN_POINT('Ctrl Pts',(-1.79212976983288,0.541267439387018,
1.63863764640214));
#23649=CARTESIAN_POINT('Ctrl Pts',(-1.00993315330316,0.720837529677195,
1.12589971949673));
#23650=CARTESIAN_POINT('Ctrl Pts',(-1.25179094217685,0.825567715093928,
1.34900830339197));
#23651=CARTESIAN_POINT('Ctrl Pts',(-1.49701757504304,0.771065844731935,
1.53195557707745));
#23652=CARTESIAN_POINT('Ctrl Pts',(-1.74562013410099,0.557477346013106,
1.67474624941239));
#23653=CARTESIAN_POINT('Ctrl Pts',(-0.956735633325592,0.717530565095652,
1.16769179538367));
#23654=CARTESIAN_POINT('Ctrl Pts',(-1.1874504232267,0.823961384252212,1.39903449435105));
#23655=CARTESIAN_POINT('Ctrl Pts',(-1.42496257773994,0.777060632929274,
1.58878199846585));
#23656=CARTESIAN_POINT('Ctrl Pts',(-1.66940588754285,0.576871348730687,
1.73683890344256));
#23657=CARTESIAN_POINT('Ctrl Pts',(-0.890308540641222,0.701101131459803,
1.22804130170825));
#23658=CARTESIAN_POINT('Ctrl Pts',(-1.10640797973513,0.80706000931713,1.47142017171287));
#23659=CARTESIAN_POINT('Ctrl Pts',(-1.33243573819092,0.767978311363814,
1.67099665961543));
#23660=CARTESIAN_POINT('Ctrl Pts',(-1.56839818009432,0.583845206097258,
1.82676536339563));
#23661=CARTESIAN_POINT('Ctrl Pts',(-0.860233953705641,0.681352489183287,
1.2635364344865));
#23662=CARTESIAN_POINT('Ctrl Pts',(-1.06916866744104,0.784556163294569,
1.51398418220584));
#23663=CARTESIAN_POINT('Ctrl Pts',(-1.28799335847826,0.747275208483434,
1.71946457116169));
#23664=CARTESIAN_POINT('Ctrl Pts',(-1.51699586639177,0.569616647707412,
1.87977332297458));
#23665=CARTESIAN_POINT('Ctrl Pts',(-0.846087143187382,0.667616851769879,
1.28318517919043));
#23666=CARTESIAN_POINT('Ctrl Pts',(-1.05147036139455,0.768564946360843,
1.53754499301448));
#23667=CARTESIAN_POINT('Ctrl Pts',(-1.26643337142019,0.731592934569703,
1.74612783237292));
#23668=CARTESIAN_POINT('Ctrl Pts',(-1.4909761732643,0.556700816396459,1.90893369726574));
#23669=CARTESIAN_POINT('',(-0.849391336665505,0.669228599956957,1.28727233489076));
#23670=CARTESIAN_POINT('Ctrl Pts',(-1.03556549162895,0.720159740047643,
1.10727038327973));
#23671=CARTESIAN_POINT('Ctrl Pts',(-1.00975899746819,0.720933639361786,
1.12801545944061));
#23672=CARTESIAN_POINT('Ctrl Pts',(-0.981660765603669,0.719952669695422,
1.15133239961436));
#23673=CARTESIAN_POINT('Ctrl Pts',(-0.932697144982725,0.712287980257843,
1.19509600545502));
#23674=CARTESIAN_POINT('Ctrl Pts',(-0.91338947619488,0.707566124812641,
1.21324740617476));
#23675=CARTESIAN_POINT('Ctrl Pts',(-0.882563548281158,0.694825406568518,
1.24538218411192));
#23676=CARTESIAN_POINT('Ctrl Pts',(-0.866448281268894,0.685758102881577,
1.26364457695098));
#23677=CARTESIAN_POINT('Ctrl Pts',(-0.849391336665505,0.669228599956957,
1.28727233489076));
#23678=CARTESIAN_POINT('Ctrl Pts',(-0.849391336665505,0.669228599956957,
1.28727233489076));
#23679=CARTESIAN_POINT('Ctrl Pts',(-0.940530841324424,0.713346345736856,
1.39987124007464));
#23680=CARTESIAN_POINT('Ctrl Pts',(-1.03355488521186,0.73033241101646,1.50346488650363));
#23681=CARTESIAN_POINT('Ctrl Pts',(-1.2462884798982,0.707591441492497,1.715480776583));
#23682=CARTESIAN_POINT('Ctrl Pts',(-1.36701797678012,0.653180259586498,
1.81902921434248));
#23683=CARTESIAN_POINT('Ctrl Pts',(-1.49065195897357,0.55695325007777,1.90869858745619));
#23684=CARTESIAN_POINT('Ctrl Pts',(-0.849391336665504,0.669228599956957,
1.28727233489076));
#23685=CARTESIAN_POINT('Ctrl Pts',(-1.05431200258793,0.768424199911631,
1.54044292999952));
#23686=CARTESIAN_POINT('Ctrl Pts',(-1.26875982659235,0.73045746052879,1.74808806061869));
#23687=CARTESIAN_POINT('Ctrl Pts',(-1.49273480867877,0.555328381808437,
1.91020772674828));
#23688=CARTESIAN_POINT('Ctrl Pts',(-0.820505999621324,0.701662213869995,
1.28727233489076));
#23689=CARTESIAN_POINT('Ctrl Pts',(-1.02095396380933,0.808833265245786,
1.54044292999952));
#23690=CARTESIAN_POINT('Ctrl Pts',(-1.23640500988538,0.779555824624011,
1.74808806061869));
#23691=CARTESIAN_POINT('Ctrl Pts',(-1.46685913784949,0.613829892004671,
1.91020772674828));
#23692=CARTESIAN_POINT('Ctrl Pts',(-0.791620662577143,0.734095827783032,
1.28727233489076));
#23693=CARTESIAN_POINT('Ctrl Pts',(-0.98759592503072,0.849242330579942,
1.54044292999952));
#23694=CARTESIAN_POINT('Ctrl Pts',(-1.20405019317841,0.828654188719233,
1.74808806061869));
#23695=CARTESIAN_POINT('Ctrl Pts',(-1.4409834670202,0.672331402200905,1.91020772674828));
#23696=CARTESIAN_POINT('Ctrl Pts',(-0.762735325532963,0.766529441696069,
1.28727233489076));
#23697=CARTESIAN_POINT('Ctrl Pts',(-0.954237886252114,0.889651395914097,
1.54044292999952));
#23698=CARTESIAN_POINT('Ctrl Pts',(-1.17169537647143,0.877752552814453,
1.74808806061869));
#23699=CARTESIAN_POINT('Ctrl Pts',(-1.41510779619092,0.730832912397138,
1.91020772674828));
#23700=CARTESIAN_POINT('Ctrl Pts',(-0.849391336665504,0.669228599956957,
1.28727233489076));
#23701=CARTESIAN_POINT('Ctrl Pts',(-0.835451887202037,0.685790285668798,
1.28797191329046));
#23702=CARTESIAN_POINT('Ctrl Pts',(-0.82128510159093,0.702160750604672,
1.28831907556383));
#23703=CARTESIAN_POINT('Ctrl Pts',(-0.806883726521851,0.718337308749603,
1.288319084765));
#23704=CARTESIAN_POINT('Ctrl Pts',(-0.792392236721721,0.734615089602754,
1.28831909402374));
#23705=CARTESIAN_POINT('Ctrl Pts',(-0.777677820212499,0.750680064449589,
1.28796761487395));
#23706=CARTESIAN_POINT('Ctrl Pts',(-0.762735325532963,0.766529441696069,
1.28727233489076));
#23707=CARTESIAN_POINT('Origin',(0.,0.,1.37171309575435));
#23708=CARTESIAN_POINT('',(-0.762339710524744,1.00491994924733,1.10727038327973));
#23709=CARTESIAN_POINT('Ctrl Pts',(-1.52399042602929,1.07301833748062,1.63615580822897));
#23710=CARTESIAN_POINT('Ctrl Pts',(-1.42568690035968,1.11607945893995,1.58735805514612));
#23711=CARTESIAN_POINT('Ctrl Pts',(-1.33168344006467,1.14151594859478,1.5385809502084));
#23712=CARTESIAN_POINT('Ctrl Pts',(-1.14153741491427,1.16157559133822,1.42806953503213));
#23713=CARTESIAN_POINT('Ctrl Pts',(-1.04542790122454,1.15142699410503,1.36461306044571));
#23714=CARTESIAN_POINT('Ctrl Pts',(-0.882986840618225,1.09387499947176,
1.23357020765531));
#23715=CARTESIAN_POINT('Ctrl Pts',(-0.818276751491845,1.05413090753297,
1.17136442658356));
#23716=CARTESIAN_POINT('Ctrl Pts',(-0.762339710524744,1.00491994924733,
1.10727038327973));
#23717=CARTESIAN_POINT('Origin',(0.,0.,1.10727038327973));
#23718=CARTESIAN_POINT('Ctrl Pts',(-0.486216001172379,0.96185791365589,
1.28318567027397));
#23719=CARTESIAN_POINT('Ctrl Pts',(-0.629961036964704,1.13989141130718,
1.53751096017972));
#23720=CARTESIAN_POINT('Ctrl Pts',(-0.84046318352097,1.19690070060403,1.74607168007008));
#23721=CARTESIAN_POINT('Ctrl Pts',(-1.11772244084118,1.13288578154644,1.90886782994506));
#23722=CARTESIAN_POINT('Ctrl Pts',(-0.496846021492854,0.978417321314553,
1.26357731004417));
#23723=CARTESIAN_POINT('Ctrl Pts',(-0.643585521081937,1.15940183561927,
1.51399891879436));
#23724=CARTESIAN_POINT('Ctrl Pts',(-0.857895946504486,1.21707904013549,
1.71946418982835));
#23725=CARTESIAN_POINT('Ctrl Pts',(-1.14010192848643,1.15131005161592,1.87976839865855));
#23726=CARTESIAN_POINT('Ctrl Pts',(-0.510215828707944,1.01174306480633,
1.22814964935774));
#23727=CARTESIAN_POINT('Ctrl Pts',(-0.661178469414083,1.19911435608045,
1.47151698835253));
#23728=CARTESIAN_POINT('Ctrl Pts',(-0.882459067352746,1.25929534063486,
1.67109028087187));
#23729=CARTESIAN_POINT('Ctrl Pts',(-1.17406335818981,1.19229498704013,1.82686350557264));
#23730=CARTESIAN_POINT('Ctrl Pts',(-0.513157287930765,1.07994419721084,
1.16792318405107));
#23731=CARTESIAN_POINT('Ctrl Pts',(-0.667766287860981,1.2814248116504,1.39927998114664));
#23732=CARTESIAN_POINT('Ctrl Pts',(-0.899659869879336,1.35048605385199,
1.58904519906558));
#23733=CARTESIAN_POINT('Ctrl Pts',(-1.20898915642793,1.28706885932715,1.73712239616959));
#23734=CARTESIAN_POINT('Ctrl Pts',(-0.505885563397483,1.13261799505841,
1.12620659350917));
#23735=CARTESIAN_POINT('Ctrl Pts',(-0.661308446532945,1.34530596753016,
1.34934531900259));
#23736=CARTESIAN_POINT('Ctrl Pts',(-0.90016534752349,1.42259827975627,1.53232296148775));
#23737=CARTESIAN_POINT('Ctrl Pts',(-1.22248177762695,1.3643546712912,1.67514376227795));
#23738=CARTESIAN_POINT('Ctrl Pts',(-0.498486987186291,1.16512794184932,
1.10192284729582));
#23739=CARTESIAN_POINT('Ctrl Pts',(-0.653810349677836,1.38487268717996,
1.32027771712106));
#23740=CARTESIAN_POINT('Ctrl Pts',(-0.896559590305325,1.46759648753937,
1.4993370241196));
#23741=CARTESIAN_POINT('Ctrl Pts',(-1.22673470906876,1.41329934292755,1.63910076829144));
#23742=CARTESIAN_POINT('',(-0.488533777383804,0.964710998256926,1.28727233489076));
#23743=CARTESIAN_POINT('',(-0.500065917147829,1.15799828028599,1.10727038327973));
#23744=CARTESIAN_POINT('Ctrl Pts',(-0.488533777383804,0.964710998256926,
1.28727233489076));
#23745=CARTESIAN_POINT('Ctrl Pts',(-0.50620036615867,0.992182562457059,
1.25478273943377));
#23746=CARTESIAN_POINT('Ctrl Pts',(-0.512561466012053,1.01873815563885,
1.2282992378118));
#23747=CARTESIAN_POINT('Ctrl Pts',(-0.513908711038649,1.08065739676658,
1.17205963503343));
#23748=CARTESIAN_POINT('Ctrl Pts',(-0.510455723374509,1.11643729240398,
1.14130666672571));
#23749=CARTESIAN_POINT('Ctrl Pts',(-0.500065917147829,1.15799828028599,
1.10727038327973));
#23750=CARTESIAN_POINT('Ctrl Pts',(-0.488533777383804,0.964710998256926,
1.28727233489076));
#23751=CARTESIAN_POINT('Ctrl Pts',(-0.552615413818275,1.04310952295002,
1.39987124007464));
#23752=CARTESIAN_POINT('Ctrl Pts',(-0.629833086622262,1.09769367964031,
1.50346488650363));
#23753=CARTESIAN_POINT('Ctrl Pts',(-0.832357123065218,1.16666286599128,
1.715480776583));
#23754=CARTESIAN_POINT('Ctrl Pts',(-0.964772942765737,1.16815913695893,
1.81902921434248));
#23755=CARTESIAN_POINT('Ctrl Pts',(-1.11743425489732,1.13295228123076,1.90869858745619));
#23756=CARTESIAN_POINT('Ctrl Pts',(-0.500065917147829,1.15799828028599,
1.10727038327973));
#23757=CARTESIAN_POINT('Ctrl Pts',(-0.551550501629625,1.22729623661065,
1.18103565901047));
#23758=CARTESIAN_POINT('Ctrl Pts',(-0.614972484709036,1.28900548463589,
1.25302429310895));
#23759=CARTESIAN_POINT('Ctrl Pts',(-0.774686679112503,1.38528731335191,
1.39260788389886));
#23760=CARTESIAN_POINT('Ctrl Pts',(-0.867524531197774,1.41556887304308,
1.45574709063869));
#23761=CARTESIAN_POINT('Ctrl Pts',(-1.05077615643305,1.43300950021463,1.55895701082594));
#23762=CARTESIAN_POINT('Ctrl Pts',(-1.13327165021096,1.42795915557245,1.59904902099413));
#23763=CARTESIAN_POINT('Ctrl Pts',(-1.21572094522251,1.4127766116927,1.63615580822897));
#23764=CARTESIAN_POINT('Ctrl Pts',(-0.769785488061408,1.0071890534957,1.10157231096021));
#23765=CARTESIAN_POINT('Ctrl Pts',(-0.974501097544568,1.18205566887762,
1.31988785480615));
#23766=CARTESIAN_POINT('Ctrl Pts',(-1.23029122098199,1.2025174778094,1.4989096332868));
#23767=CARTESIAN_POINT('Ctrl Pts',(-1.53715585837368,1.06857448029104,1.63863764640214));
#23768=CARTESIAN_POINT('Ctrl Pts',(-0.727074783470151,0.994461965292039,
1.13400885567558));
#23769=CARTESIAN_POINT('Ctrl Pts',(-0.922448816386925,1.16858584308541,
1.35870212368825));
#23770=CARTESIAN_POINT('Ctrl Pts',(-1.17054629234371,1.19383871456862,1.54297833728481));
#23771=CARTESIAN_POINT('Ctrl Pts',(-1.47149928669632,1.06996683960028,1.68678245041581));
#23772=CARTESIAN_POINT('Ctrl Pts',(-0.673083751047335,0.971974682567364,
1.18052322600159));
#23773=CARTESIAN_POINT('Ctrl Pts',(-0.856229621362336,1.1438936589507,1.41439979544558));
#23774=CARTESIAN_POINT('Ctrl Pts',(-1.0936426848353,1.17420151395341,1.60622137130565));
#23775=CARTESIAN_POINT('Ctrl Pts',(-1.38546708108516,1.06281232835789,1.75589800730002));
#23776=CARTESIAN_POINT('Ctrl Pts',(-0.621030952892813,0.932030917609336,
1.24109849008298));
#23777=CARTESIAN_POINT('Ctrl Pts',(-0.791463701885433,1.09790581924279,
1.48710325590114));
#23778=CARTESIAN_POINT('Ctrl Pts',(-1.01576709402367,1.13059499103696,1.68883275601271));
#23779=CARTESIAN_POINT('Ctrl Pts',(-1.29394102274663,1.03008879377588,1.84628852230556));
#23780=CARTESIAN_POINT('Ctrl Pts',(-0.605279141158067,0.909472892481623,
1.26844862066248));
#23781=CARTESIAN_POINT('Ctrl Pts',(-0.771469550259548,1.07134082867159,
1.51987386218776));
#23782=CARTESIAN_POINT('Ctrl Pts',(-0.990137606500526,1.10338745862407,
1.72613059618619));
#23783=CARTESIAN_POINT('Ctrl Pts',(-1.26153883267189,1.00543407447983,1.88706341654737));
#23784=CARTESIAN_POINT('Ctrl Pts',(-0.598371737953918,0.89639666323125,
1.28318517919043));
#23785=CARTESIAN_POINT('Ctrl Pts',(-0.762508109189138,1.055870911185,1.53754499301448));
#23786=CARTESIAN_POINT('Ctrl Pts',(-0.978375060596135,1.08713566171041,
1.74612783237291));
#23787=CARTESIAN_POINT('Ctrl Pts',(-1.24597259217491,0.990190914807483,
1.90893369726573));
#23788=CARTESIAN_POINT('',(-0.601016155111926,0.89895057878464,1.28727233489076));
#23789=CARTESIAN_POINT('Ctrl Pts',(-0.762339710524744,1.00491994924733,
1.10727038327973));
#23790=CARTESIAN_POINT('Ctrl Pts',(-0.737557128050267,0.997681325972047,
1.12801545944073));
#23791=CARTESIAN_POINT('Ctrl Pts',(-0.711137257836933,0.988065537220461,
1.15133239961458));
#23792=CARTESIAN_POINT('Ctrl Pts',(-0.666938606676026,0.965645393507086,
1.19509600545601));
#23793=CARTESIAN_POINT('Ctrl Pts',(-0.650035056038688,0.955188244339594,
1.2132474061757));
#23794=CARTESIAN_POINT('Ctrl Pts',(-0.624654954884539,0.933545365639427,
1.24538218411151));
#23795=CARTESIAN_POINT('Ctrl Pts',(-0.612130376112959,0.919941956007105,
1.26364457695062));
#23796=CARTESIAN_POINT('Ctrl Pts',(-0.601016155111926,0.89895057878464,
1.28727233489076));
#23797=CARTESIAN_POINT('Ctrl Pts',(-0.601016155111926,0.89895057878464,
1.28727233489076));
#23798=CARTESIAN_POINT('Ctrl Pts',(-0.674061841710201,0.969072704191387,
1.39987124007464));
#23799=CARTESIAN_POINT('Ctrl Pts',(-0.757283981982513,1.01397342270847,
1.50346488650363));
#23800=CARTESIAN_POINT('Ctrl Pts',(-0.966632999495317,1.05808377148838,
1.715480776583));
#23801=CARTESIAN_POINT('Ctrl Pts',(-1.09826755410688,1.04364312863621,1.81902921434248));
#23802=CARTESIAN_POINT('Ctrl Pts',(-1.24558623976355,0.990330805779366,
1.90869858745619));
#23803=CARTESIAN_POINT('Ctrl Pts',(-0.601016155111926,0.89895057878464,
1.28727233489076));
#23804=CARTESIAN_POINT('Ctrl Pts',(-0.765254163607779,1.056615168778,1.54044292999952));
#23805=CARTESIAN_POINT('Ctrl Pts',(-0.980938531722802,1.08677467590956,
1.74808806061869));
#23806=CARTESIAN_POINT('Ctrl Pts',(-1.24806925945699,0.989429100179333,
1.91020772674828));
#23807=CARTESIAN_POINT('Ctrl Pts',(-0.563522029202552,0.920870718608735,
1.28727233489076));
#23808=CARTESIAN_POINT('Ctrl Pts',(-0.721041695541499,1.08473827279984,
1.54044292999952));
#23809=CARTESIAN_POINT('Ctrl Pts',(-0.934995043558668,1.12347180680942,
1.74808806061869));
#23810=CARTESIAN_POINT('Ctrl Pts',(-1.20538207325406,1.03707132063747,1.91020772674828));
#23811=CARTESIAN_POINT('Ctrl Pts',(-0.526027903293178,0.94279085843283,
1.28727233489076));
#23812=CARTESIAN_POINT('Ctrl Pts',(-0.676829227475217,1.11286137682168,
1.54044292999952));
#23813=CARTESIAN_POINT('Ctrl Pts',(-0.889051555394535,1.16016893770927,
1.74808806061869));
#23814=CARTESIAN_POINT('Ctrl Pts',(-1.16269488705113,1.0847135410956,1.91020772674828));
#23815=CARTESIAN_POINT('Ctrl Pts',(-0.488533777383804,0.964710998256926,
1.28727233489076));
#23816=CARTESIAN_POINT('Ctrl Pts',(-0.632616759408936,1.14098448084351,
1.54044292999952));
#23817=CARTESIAN_POINT('Ctrl Pts',(-0.843108067230401,1.19686606860912,
1.74808806061869));
#23818=CARTESIAN_POINT('Ctrl Pts',(-1.1200077008482,1.13235576155374,1.91020772674828));
#23819=CARTESIAN_POINT('Ctrl Pts',(-0.601016155111926,0.89895057878464,
1.28727233489076));
#23820=CARTESIAN_POINT('Ctrl Pts',(-0.582641108525671,0.910394151125278,
1.28797191329047));
#23821=CARTESIAN_POINT('Ctrl Pts',(-0.564108942884267,0.921585610967823,
1.28831907556383));
#23822=CARTESIAN_POINT('Ctrl Pts',(-0.545413589903933,0.932520162364073,
1.288319084765));
#23823=CARTESIAN_POINT('Ctrl Pts',(-0.526601253184359,0.943523135293236,
1.28831909402374));
#23824=CARTESIAN_POINT('Ctrl Pts',(-0.507642661237903,0.954254829541775,
1.28796761487395));
#23825=CARTESIAN_POINT('Ctrl Pts',(-0.488533777383804,0.964710998256926,
1.28727233489076));
#23826=CARTESIAN_POINT('Origin',(0.,0.,1.37171309575435));
#23827=CARTESIAN_POINT('',(-0.414490807021284,1.19131159212569,1.10727038327973));
#23828=CARTESIAN_POINT('Ctrl Pts',(-1.11782012388912,1.4914400228729,1.63615580822897));
#23829=CARTESIAN_POINT('Ctrl Pts',(-1.01102129689809,1.50201612299693,1.58735805514594));
#23830=CARTESIAN_POINT('Ctrl Pts',(-0.913758385849714,1.49715899547352,
1.53858095020821));
#23831=CARTESIAN_POINT('Ctrl Pts',(-0.726719999074283,1.45747849623496,
1.42806953503212));
#23832=CARTESIAN_POINT('Ctrl Pts',(-0.638450508815834,1.41812713365384,
1.3646130604457));
#23833=CARTESIAN_POINT('Ctrl Pts',(-0.501744424014167,1.31319488582044,
1.2335702076553));
#23834=CARTESIAN_POINT('Ctrl Pts',(-0.45248307191557,1.25539949095026,1.17136442658356));
#23835=CARTESIAN_POINT('Ctrl Pts',(-0.414490807021284,1.19131159212569,
1.10727038327973));
#23836=CARTESIAN_POINT('Origin',(0.,0.,1.10727038327973));
#23837=CARTESIAN_POINT('Ctrl Pts',(-0.165188454748262,1.06503024383179,
1.28318567027397));
#23838=CARTESIAN_POINT('Ctrl Pts',(-0.246882731381371,1.27876982080874,
1.53751096017972));
#23839=CARTESIAN_POINT('Ctrl Pts',(-0.429465330327865,1.39803761752215,
1.74607168007008));
#23840=CARTESIAN_POINT('Ctrl Pts',(-0.712936251587744,1.42283363397204,
1.90886782994506));
#23841=CARTESIAN_POINT('Ctrl Pts',(-0.168932913531384,1.07930558594879,
1.26847940010162));
#23842=CARTESIAN_POINT('Ctrl Pts',(-0.252026844288351,1.29586765564979,
1.51987665322459));
#23843=CARTESIAN_POINT('Ctrl Pts',(-0.437225780288053,1.41640054440424,
1.72611612827485));
#23844=CARTESIAN_POINT('Ctrl Pts',(-0.724629310334697,1.44116225705855,
1.88704325648018));
#23845=CARTESIAN_POINT('Ctrl Pts',(-0.172580460092752,1.10652474870095,
1.24117906537517));
#23846=CARTESIAN_POINT('Ctrl Pts',(-0.257658341550684,1.32856177300788,
1.48716667186368));
#23847=CARTESIAN_POINT('Ctrl Pts',(-0.447493258920491,1.45233913898617,
1.68888789608761));
#23848=CARTESIAN_POINT('Ctrl Pts',(-0.742078309759816,1.47786361346603,
1.84634469876801));
#23849=CARTESIAN_POINT('Ctrl Pts',(-0.161305070542798,1.171005693206,1.18072695962337));
#23850=CARTESIAN_POINT('Ctrl Pts',(-0.246868029800147,1.40706779462019,
1.41461248446318));
#23851=CARTESIAN_POINT('Ctrl Pts',(-0.444855864337702,1.54132997390971,
1.60644654213684));
#23852=CARTESIAN_POINT('Ctrl Pts',(-0.755334809435783,1.57392460995617,
1.75614031701006));
#23853=CARTESIAN_POINT('Ctrl Pts',(-0.136821749681419,1.22396679065339,
1.13430117558029));
#23854=CARTESIAN_POINT('Ctrl Pts',(-0.21960593824905,1.47209169926767,1.35902160674437));
#23855=CARTESIAN_POINT('Ctrl Pts',(-0.422262554132523,1.61714699314179,
1.54332567193682));
#23856=CARTESIAN_POINT('Ctrl Pts',(-0.744733799933248,1.65939158627326,
1.68715809360678));
#23857=CARTESIAN_POINT('Ctrl Pts',(-0.114044962799315,1.26214347192869,
1.10192284729582));
#23858=CARTESIAN_POINT('Ctrl Pts',(-0.193861398098013,1.51913070253036,
1.32027771712106));
#23859=CARTESIAN_POINT('Ctrl Pts',(-0.399166585072151,1.67281935264038,
1.4993370241196));
#23860=CARTESIAN_POINT('Ctrl Pts',(-0.729960523721729,1.72320942225876,
1.63910076829144));
#23861=CARTESIAN_POINT('',(-0.166511139289342,1.06845992077163,1.28727233489076));
#23862=CARTESIAN_POINT('',(-0.117749801015222,1.25585067703094,1.10727038327973));
#23863=CARTESIAN_POINT('Ctrl Pts',(-0.166511139289342,1.06845992077163,
1.28727233489076));
#23864=CARTESIAN_POINT('Ctrl Pts',(-0.174823883464338,1.10004620708051,
1.25478273943433));
#23865=CARTESIAN_POINT('Ctrl Pts',(-0.172667519342151,1.12726776497775,
1.22829923781232));
#23866=CARTESIAN_POINT('Ctrl Pts',(-0.154814727716362,1.18657278434537,
1.17205963503373));
#23867=CARTESIAN_POINT('Ctrl Pts',(-0.14047414548886,1.21953445537415,1.14130666672595));
#23868=CARTESIAN_POINT('Ctrl Pts',(-0.117749801015222,1.25585067703094,
1.10727038327973));
#23869=CARTESIAN_POINT('Ctrl Pts',(-0.166511139289342,1.06845992077163,
1.28727233489076));
#23870=CARTESIAN_POINT('Ctrl Pts',(-0.203229920731113,1.16282366323453,
1.39987124007464));
#23871=CARTESIAN_POINT('Ctrl Pts',(-0.259800859583567,1.23859785430383,
1.50346488650363));
#23872=CARTESIAN_POINT('Ctrl Pts',(-0.431100013478375,1.36677481743678,
1.715480776583));
#23873=CARTESIAN_POINT('Ctrl Pts',(-0.556572568507924,1.40911659430226,
1.81902921434248));
#23874=CARTESIAN_POINT('Ctrl Pts',(-0.712641620935351,1.42280782457595,
1.90869858745619));
#23875=CARTESIAN_POINT('Ctrl Pts',(-0.117749801015222,1.25585067703094,
1.10727038327973));
#23876=CARTESIAN_POINT('Ctrl Pts',(-0.145300304395599,1.33766656151262,
1.18103565901044));
#23877=CARTESIAN_POINT('Ctrl Pts',(-0.18654898832971,1.41595401455117,1.25302429310889));
#23878=CARTESIAN_POINT('Ctrl Pts',(-0.30869349233915,1.55687787546591,1.39260788389877));
#23879=CARTESIAN_POINT('Ctrl Pts',(-0.387630019962927,1.61436582414941,
1.45574709063861));
#23880=CARTESIAN_POINT('Ctrl Pts',(-0.556523222076064,1.68758071271376,
1.55895701082589));
#23881=CARTESIAN_POINT('Ctrl Pts',(-0.636541741320461,1.70827005906903,
1.59904902099411));
#23882=CARTESIAN_POINT('Ctrl Pts',(-0.71964734468187,1.71930883511106,1.63615580822897));
#23883=CARTESIAN_POINT('Ctrl Pts',(-0.420870970491669,1.19577051030242,
1.1015723109602));
#23884=CARTESIAN_POINT('Ctrl Pts',(-0.561530328976122,1.425339146688,1.31988785480614));
#23885=CARTESIAN_POINT('Ctrl Pts',(-0.79847814597965,1.52384297854319,1.49890963328678));
#23886=CARTESIAN_POINT('Ctrl Pts',(-1.13171442150225,1.49128200586798,1.63863764640213));
#23887=CARTESIAN_POINT('Ctrl Pts',(-0.393355414961742,1.17679362500494,
1.12589971949673));
#23888=CARTESIAN_POINT('Ctrl Pts',(-0.527463617924698,1.40368256628313,
1.34900830339197));
#23889=CARTESIAN_POINT('Ctrl Pts',(-0.757891527007923,1.50373022520315,
1.53195557707744));
#23890=CARTESIAN_POINT('Ctrl Pts',(-1.08455939173712,1.47705841783302,1.67474624941237));
#23891=CARTESIAN_POINT('Ctrl Pts',(-0.352262141476107,1.14284817765567,
1.16769296545954));
#23892=CARTESIAN_POINT('Ctrl Pts',(-0.476355861470115,1.3645632700682,1.39903566442692));
#23893=CARTESIAN_POINT('Ctrl Pts',(-0.696074558068188,1.46622517664402,
1.58878359776798));
#23894=CARTESIAN_POINT('Ctrl Pts',(-1.01150165877891,1.44794881615932,1.73684050274469));
#23895=CARTESIAN_POINT('Ctrl Pts',(-0.308178085105591,1.09051150146367,
1.22804267083047));
#23896=CARTESIAN_POINT('Ctrl Pts',(-0.420725138053456,1.30325409768322,
1.47142154083508));
#23897=CARTESIAN_POINT('Ctrl Pts',(-0.626556636662153,1.40449154295595,
1.67099852964049));
#23898=CARTESIAN_POINT('Ctrl Pts',(-0.925684985930704,1.39421997501402,
1.8267672334207));
#23899=CARTESIAN_POINT('Ctrl Pts',(-0.295454942931511,1.05685857441837,
1.2635364344865));
#23900=CARTESIAN_POINT('Ctrl Pts',(-0.403825079433304,1.26316084408195,
1.51398418220584));
#23901=CARTESIAN_POINT('Ctrl Pts',(-0.602771168700623,1.36162184430235,
1.71946457116168));
#23902=CARTESIAN_POINT('Ctrl Pts',(-0.892463171324776,1.35249734632791,
1.87977332297457));
#23903=CARTESIAN_POINT('Ctrl Pts',(-0.292083537908477,1.03743092373275,
1.28318517919043));
#23904=CARTESIAN_POINT('Ctrl Pts',(-0.3989062505499,1.23982087453714,1.53754499301448));
#23905=CARTESIAN_POINT('Ctrl Pts',(-0.594546582101046,1.33626197576335,
1.74612783237291));
#23906=CARTESIAN_POINT('Ctrl Pts',(-0.879004532561914,1.32675422741137,
1.90893369726573));
#23907=CARTESIAN_POINT('',(-0.293809324770207,1.04067701160391,1.28727233489076));
#23908=CARTESIAN_POINT('Ctrl Pts',(-0.414490807021284,1.19131159212569,
1.10727038327973));
#23909=CARTESIAN_POINT('Ctrl Pts',(-0.393158028076679,1.17676901314191,
1.12801545944031));
#23910=CARTESIAN_POINT('Ctrl Pts',(-0.371002680489146,1.15945966570541,
1.15133239961407));
#23911=CARTESIAN_POINT('Ctrl Pts',(-0.335895470715533,1.124478707594,1.19509600545469));
#23912=CARTESIAN_POINT('Ctrl Pts',(-0.323050675538606,1.10930988332448,
1.21324740617417));
#23913=CARTESIAN_POINT('Ctrl Pts',(-0.305600782276718,1.08088339992881,
1.24538218411099));
#23914=CARTESIAN_POINT('Ctrl Pts',(-0.297892884779784,1.06407548086635,
1.26364457695016));
#23915=CARTESIAN_POINT('Ctrl Pts',(-0.293809324770207,1.04067701160391,
1.28727233489076));
#23916=CARTESIAN_POINT('Ctrl Pts',(-0.293809324770207,1.04067701160391,
1.28727233489076));
#23917=CARTESIAN_POINT('Ctrl Pts',(-0.341610972564374,1.12993947443311,
1.39987124007464));
#23918=CARTESIAN_POINT('Ctrl Pts',(-0.406884846288962,1.19835965101752,
1.50346488650363));
#23919=CARTESIAN_POINT('Ctrl Pts',(-0.592356746173702,1.30500348982786,
1.715480776583));
#23920=CARTESIAN_POINT('Ctrl Pts',(-0.722011051157661,1.33194693676576,
1.81902921434248));
#23921=CARTESIAN_POINT('Ctrl Pts',(-0.878593860895847,1.32676788217082,
1.90869858745619));
#23922=CARTESIAN_POINT('Ctrl Pts',(-0.293809324770207,1.04067701160391,
1.28727233489076));
#23923=CARTESIAN_POINT('Ctrl Pts',(-0.401287915254421,1.24137728305361,
1.54044292999952));
#23924=CARTESIAN_POINT('Ctrl Pts',(-0.59709613876759,1.3367108140079,1.74808806061869));
#23925=CARTESIAN_POINT('Ctrl Pts',(-0.881233995309716,1.32667760446677,
1.91020772674828));
#23926=CARTESIAN_POINT('Ctrl Pts',(-0.251376596276585,1.04993798132648,
1.28727233489076));
#23927=CARTESIAN_POINT('Ctrl Pts',(-0.35054884232117,1.25446154039629,1.54044292999952));
#23928=CARTESIAN_POINT('Ctrl Pts',(-0.542061247874906,1.35741454085596,
1.74808806061869));
#23929=CARTESIAN_POINT('Ctrl Pts',(-0.825913812937791,1.3587969827055,1.91020772674828));
#23930=CARTESIAN_POINT('Ctrl Pts',(-0.208943867782964,1.05919895104906,
1.28727233489076));
#23931=CARTESIAN_POINT('Ctrl Pts',(-0.299809769387921,1.26754579773896,
1.54044292999952));
#23932=CARTESIAN_POINT('Ctrl Pts',(-0.487026356982221,1.37811826770401,
1.74808806061869));
#23933=CARTESIAN_POINT('Ctrl Pts',(-0.770593630565866,1.39091636094422,
1.91020772674828));
#23934=CARTESIAN_POINT('Ctrl Pts',(-0.166511139289342,1.06845992077163,
1.28727233489076));
#23935=CARTESIAN_POINT('Ctrl Pts',(-0.24907069645467,1.28063005508163,1.54044292999952));
#23936=CARTESIAN_POINT('Ctrl Pts',(-0.431991466089537,1.39882199455207,
1.74808806061869));
#23937=CARTESIAN_POINT('Ctrl Pts',(-0.715273448193941,1.42303573918295,
1.91020772674828));
#23938=CARTESIAN_POINT('Ctrl Pts',(-0.293809324770207,1.04067701160391,
1.28727233489076));
#23939=CARTESIAN_POINT('Ctrl Pts',(-0.272797358647504,1.04588229398058,
1.28797191329047));
#23940=CARTESIAN_POINT('Ctrl Pts',(-0.251713870469976,1.05079925066492,
1.28831907556383));
#23941=CARTESIAN_POINT('Ctrl Pts',(-0.230554570986284,1.05542144523633,
1.288319084765));
#23942=CARTESIAN_POINT('Ctrl Pts',(-0.209262869938631,1.06007256258898,
1.28831909402374));
#23943=CARTESIAN_POINT('Ctrl Pts',(-0.187915901626935,1.06442048323406,
1.28796761487395));
#23944=CARTESIAN_POINT('Ctrl Pts',(-0.166511139289342,1.06845992077163,
1.28727233489076));
#23945=CARTESIAN_POINT('Origin',(0.,0.,1.37171309575435));
#23946=CARTESIAN_POINT('',(-0.0260686553993153,1.26108935601086,1.10727038327973));
#23947=CARTESIAN_POINT('Ctrl Pts',(-0.602229799711917,1.76386916735272,
1.63615580822897));
#23948=CARTESIAN_POINT('Ctrl Pts',(-0.497389884697211,1.74092498377319,
1.58735805514609));
#23949=CARTESIAN_POINT('Ctrl Pts',(-0.406388294299314,1.70624968855532,
1.53858095020837));
#23950=CARTESIAN_POINT('Ctrl Pts',(-0.240766166368975,1.61071325107043,
1.42806953503213));
#23951=CARTESIAN_POINT('Ctrl Pts',(-0.168977132257998,1.54601110868789,
1.36461306044571));
#23952=CARTESIAN_POINT('Ctrl Pts',(-0.0713877673286501,1.40397010717826,
1.23357020765531));
#23953=CARTESIAN_POINT('Ctrl Pts',(-0.0423971966252646,1.33378082531076,
1.17136442658356));
#23954=CARTESIAN_POINT('Ctrl Pts',(-0.0260686553993154,1.26108935601086,
1.10727038327973));
#23955=CARTESIAN_POINT('Origin',(0.,0.,1.10727038327973));
#23956=CARTESIAN_POINT('Ctrl Pts',(0.172008888562255,1.06394999323939,1.28318567027397));
#23957=CARTESIAN_POINT('Ctrl Pts',(0.160362439116273,1.2924681694826,1.53750521640541));
#23958=CARTESIAN_POINT('Ctrl Pts',(0.0235777602513121,1.46231719972917,
1.74606225962531));
#23959=CARTESIAN_POINT('Ctrl Pts',(-0.238345148032627,1.57349708397912,
1.90885679993368));
#23960=CARTESIAN_POINT('Ctrl Pts',(0.172859187306825,1.07868665224636,1.2684765050474));
#23961=CARTESIAN_POINT('Ctrl Pts',(0.160753683145647,1.31032224774096,1.51986749395221));
#23962=CARTESIAN_POINT('Ctrl Pts',(0.0218713714335433,1.48218332835239,
1.72610289246662));
#23963=CARTESIAN_POINT('Ctrl Pts',(-0.243802874063088,1.59454606057878,
1.8870280554852));
#23964=CARTESIAN_POINT('Ctrl Pts',(0.177804687773572,1.10570688269946,1.24116976953012));
#23965=CARTESIAN_POINT('Ctrl Pts',(0.16550438356704,1.34316347164223,1.48715026946299));
#23966=CARTESIAN_POINT('Ctrl Pts',(0.0232152493262187,1.51954478212276,
1.68886609246491));
#23967=CARTESIAN_POINT('Ctrl Pts',(-0.249054092840224,1.63485294054343,
1.84632034153071));
#23968=CARTESIAN_POINT('Ctrl Pts',(0.208466906889381,1.16355954955659,1.18070453025513));
#23969=CARTESIAN_POINT('Ctrl Pts',(0.200040954183214,1.41450709648089,1.41458088343679));
#23970=CARTESIAN_POINT('Ctrl Pts',(0.0532384711777704,1.60338349810865,
1.60640735029516));
#23971=CARTESIAN_POINT('Ctrl Pts',(-0.231963472934463,1.73033051533549,
1.75609715466375));
#23972=CARTESIAN_POINT('Ctrl Pts',(0.248125754775117,1.20636749722078,1.13427327868628));
#23973=CARTESIAN_POINT('Ctrl Pts',(0.246072078233561,1.46793051395096,1.35898312394783));
#23974=CARTESIAN_POINT('Ctrl Pts',(0.0981648464084913,1.6685146591454,1.54327941073123));
#23975=CARTESIAN_POINT('Ctrl Pts',(-0.195461051586314,1.80834818125255,
1.6871068853877));
#23976=CARTESIAN_POINT('Ctrl Pts',(0.281595159362692,1.235641855012,1.10188938448118));
#23977=CARTESIAN_POINT('Ctrl Pts',(0.285104353628413,1.50471757474417,1.32023273220193));
#23978=CARTESIAN_POINT('Ctrl Pts',(0.137346783688563,1.71433282083683,1.49928348142626));
#23979=CARTESIAN_POINT('Ctrl Pts',(-0.161677550456858,1.86448759328998,
1.63904163215416));
#23980=CARTESIAN_POINT('',(0.171810769270086,1.06762054184321,1.28727233489076));
#23981=CARTESIAN_POINT('',(0.27609248605186,1.23077165948193,1.10727038327973));
#23982=CARTESIAN_POINT('Ctrl Pts',(0.171810769270086,1.06762054184321,1.28727233489076));
#23983=CARTESIAN_POINT('Ctrl Pts',(0.173665579012839,1.10022966448354,1.25478273943359));
#23984=CARTESIAN_POINT('Ctrl Pts',(0.184128327166778,1.12545255134546,1.22829923781164));
#23985=CARTESIAN_POINT('Ctrl Pts',(0.219433599813404,1.17633816045551,1.17205963503211));
#23986=CARTESIAN_POINT('Ctrl Pts',(0.243258020499799,1.20325508885771,1.14130666672433));
#23987=CARTESIAN_POINT('Ctrl Pts',(0.27609248605186,1.23077165948193,1.10727038327973));
#23988=CARTESIAN_POINT('Ctrl Pts',(0.171810769270086,1.06762054184321,1.28727233489076));
#23989=CARTESIAN_POINT('Ctrl Pts',(0.166049132983329,1.16871252149279,1.39987124007464));
#23990=CARTESIAN_POINT('Ctrl Pts',(0.135662485730195,1.2582594411694,1.50346488650363));
#23991=CARTESIAN_POINT('Ctrl Pts',(0.012356169078144,1.43309732687145,1.715480776583));
#23992=CARTESIAN_POINT('Ctrl Pts',(-0.093890993375447,1.51213990150266,
1.81902921434248));
#23993=CARTESIAN_POINT('Ctrl Pts',(-0.238090659850087,1.57338902476662,
1.90869858745619));
#23994=CARTESIAN_POINT('Ctrl Pts',(0.27609248605186,1.23077165948193,1.10727038327973));
#23995=CARTESIAN_POINT('Ctrl Pts',(0.275172898999398,1.31709676330282,1.18103565901045));
#23996=CARTESIAN_POINT('Ctrl Pts',(0.260135222790497,1.40429909999054,1.25302429310892));
#23997=CARTESIAN_POINT('Ctrl Pts',(0.18956320279641,1.57122974978699,1.38867432147871));
#23998=CARTESIAN_POINT('Ctrl Pts',(0.136388204217674,1.64657149028481,1.44891114041819));
#23999=CARTESIAN_POINT('Ctrl Pts',(0.00179051121351582,1.7707701091784,
1.55340617058601));
#24000=CARTESIAN_POINT('Ctrl Pts',(-0.0722162251277863,1.8188345687539,
1.59645518670947));
#24001=CARTESIAN_POINT('Ctrl Pts',(-0.153129647965885,1.85754313061971,
1.63615580822897));
#24002=CARTESIAN_POINT('Ctrl Pts',(-0.0307586699497086,1.2673016181377,
1.10157231096021));
#24003=CARTESIAN_POINT('Ctrl Pts',(-0.0935930593956182,1.52910049789877,
1.31988785480615));
#24004=CARTESIAN_POINT('Ctrl Pts',(-0.288504466724439,1.69600411129883,
1.4989096332868));
#24005=CARTESIAN_POINT('Ctrl Pts',(-0.615492891936171,1.76801245833786,
1.63863764640215));
#24006=CARTESIAN_POINT('Ctrl Pts',(-0.0104540016207206,1.24075075344812,
1.12589971949673));
#24007=CARTESIAN_POINT('Ctrl Pts',(-0.067885943246571,1.49797667332671,
1.34900830339198));
#24008=CARTESIAN_POINT('Ctrl Pts',(-0.256119480862732,1.66433379116766,
1.53195557707745));
#24009=CARTESIAN_POINT('Ctrl Pts',(-0.575041124025735,1.73991331668443,
1.67474624941239));
#24010=CARTESIAN_POINT('Ctrl Pts',(0.0181391694102201,1.19576910668283,
1.16769197379075));
#24011=CARTESIAN_POINT('Ctrl Pts',(-0.0313672401565047,1.44497975845611,
1.39903467275813));
#24012=CARTESIAN_POINT('Ctrl Pts',(-0.208916886053927,1.60956344041243,
1.58878224232001));
#24013=CARTESIAN_POINT('Ctrl Pts',(-0.514553591586059,1.68965392328533,
1.73683914729673));
#24014=CARTESIAN_POINT('Ctrl Pts',(0.0438923944102215,1.13237144427268,
1.22804151155252));
#24015=CARTESIAN_POINT('Ctrl Pts',(0.00259486397362439,1.36948062872854,
1.47142038155714));
#24016=CARTESIAN_POINT('Ctrl Pts',(-0.161878639424906,1.52936917527703,
1.67099694623232));
#24017=CARTESIAN_POINT('Ctrl Pts',(-0.449540694258325,1.61203607707659,
1.82676565001253));
#24018=CARTESIAN_POINT('Ctrl Pts',(0.0455929113995307,1.09643283244092,
1.2635364344865));
#24019=CARTESIAN_POINT('Ctrl Pts',(0.00627769421187257,1.32612616419273,
1.51398418220584));
#24020=CARTESIAN_POINT('Ctrl Pts',(-0.152505158025998,1.48124586260132,
1.71946457116169));
#24021=CARTESIAN_POINT('Ctrl Pts',(-0.430838249779549,1.56208770129018,
1.87977332297459));
#24022=CARTESIAN_POINT('Ctrl Pts',(0.0427958338931189,1.07691421721301,
1.28318517919043));
#24023=CARTESIAN_POINT('Ctrl Pts',(0.00374333123643569,1.30240853234962,
1.53754499301448));
#24024=CARTESIAN_POINT('Ctrl Pts',(-0.152519741700302,1.45458565734394,
1.74612783237292));
#24025=CARTESIAN_POINT('Ctrl Pts',(-0.425993384917093,1.53344559219597,
1.90893369726574));
#24026=CARTESIAN_POINT('',(0.042157609369957,1.08053472770428,1.28727233489076));
#24027=CARTESIAN_POINT('Ctrl Pts',(-0.0260686553993156,1.26108935601086,
1.10727038327973));
#24028=CARTESIAN_POINT('Ctrl Pts',(-0.0102738810212675,1.2406663502733,
1.12801545944048));
#24029=CARTESIAN_POINT('Ctrl Pts',(0.00544822415320251,1.21735780368012,
1.15133239961429));
#24030=CARTESIAN_POINT('Ctrl Pts',(0.0280274542413815,1.17324021107692,
1.19509600545487));
#24031=CARTESIAN_POINT('Ctrl Pts',(0.0355561559109005,1.15484454191172,
1.21324740617454));
#24032=CARTESIAN_POINT('Ctrl Pts',(0.0433677241466949,1.12241703607498,
1.24538218411135));
#24033=CARTESIAN_POINT('Ctrl Pts',(0.0455044376575714,1.10404988380783,
1.26364457695051));
#24034=CARTESIAN_POINT('Ctrl Pts',(0.042157609369957,1.08053472770428,1.28727233489076));
#24035=CARTESIAN_POINT('Ctrl Pts',(0.042157609369957,1.08053472770428,1.28727233489076));
#24036=CARTESIAN_POINT('Ctrl Pts',(0.0242791587196549,1.18019989616608,
1.39987124007464));
#24037=CARTESIAN_POINT('Ctrl Pts',(-0.0166569869072257,1.26544208722232,
1.50346488650363));
#24038=CARTESIAN_POINT('Ctrl Pts',(-0.16009648734447,1.42418037408903,1.715480776583));
#24039=CARTESIAN_POINT('Ctrl Pts',(-0.275079075974333,1.48987049850469,
1.81902921434248));
#24040=CARTESIAN_POINT('Ctrl Pts',(-0.425598593400271,1.53333167412,1.90869858745619));
#24041=CARTESIAN_POINT('Ctrl Pts',(0.042157609369957,1.08053472770428,1.28727233489076));
#24042=CARTESIAN_POINT('Ctrl Pts',(0.00195919018135101,1.30462473967982,
1.54044292999952));
#24043=CARTESIAN_POINT('Ctrl Pts',(-0.154805815536382,1.45580038421926,
1.74808806061869));
#24044=CARTESIAN_POINT('Ctrl Pts',(-0.428137407783241,1.5340616613226,1.91020772674828));
#24045=CARTESIAN_POINT('Ctrl Pts',(0.0853753293366667,1.07622999908393,
1.28727233489076));
#24046=CARTESIAN_POINT('Ctrl Pts',(0.0542581740029553,1.30138937207125,
1.54044292999952));
#24047=CARTESIAN_POINT('Ctrl Pts',(-0.0960667204863544,1.45848408198029,
1.74808806061869));
#24048=CARTESIAN_POINT('Ctrl Pts',(-0.365599354131263,1.54751412881105,
1.91020772674828));
#24049=CARTESIAN_POINT('Ctrl Pts',(0.128593049303376,1.07192527046357,1.28727233489076));
#24050=CARTESIAN_POINT('Ctrl Pts',(0.106557157824559,1.29815400446268,1.54044292999952));
#24051=CARTESIAN_POINT('Ctrl Pts',(-0.0373276254363276,1.46116777974132,
1.74808806061869));
#24052=CARTESIAN_POINT('Ctrl Pts',(-0.303061300479284,1.56096659629949,
1.91020772674828));
#24053=CARTESIAN_POINT('Ctrl Pts',(0.171810769270086,1.06762054184321,1.28727233489076));
#24054=CARTESIAN_POINT('Ctrl Pts',(0.158856141646164,1.29491863685411,1.54044292999952));
#24055=CARTESIAN_POINT('Ctrl Pts',(0.0214114696136998,1.46385147750235,
1.74808806061869));
#24056=CARTESIAN_POINT('Ctrl Pts',(-0.240523246827306,1.57441906378793,
1.91020772674828));
#24057=CARTESIAN_POINT('Ctrl Pts',(0.042157609369957,1.08053472770428,1.28727233489076));
#24058=CARTESIAN_POINT('Ctrl Pts',(0.0637496973860413,1.07899219081063,
1.28797191329047));
#24059=CARTESIAN_POINT('Ctrl Pts',(0.0853207093795777,1.07715333835806,
1.28831907556383));
#24060=CARTESIAN_POINT('Ctrl Pts',(0.106872735707655,1.07501072349525,1.288319084765));
#24061=CARTESIAN_POINT('Ctrl Pts',(0.128559621036836,1.07285470149866,1.28831909402374));
#24062=CARTESIAN_POINT('Ctrl Pts',(0.150205375722349,1.07039324377381,1.28796761487395));
#24063=CARTESIAN_POINT('Ctrl Pts',(0.171810769270086,1.06762054184321,1.28727233489076));
#24064=CARTESIAN_POINT('Origin',(0.,0.,1.37171309575435));
#24065=CARTESIAN_POINT('',(0.364905277844141,1.20742290720348,1.10727038327973));
#24066=CARTESIAN_POINT('Ctrl Pts',(-0.0276890267571662,1.86363850813291,
1.63615580822897));
#24067=CARTESIAN_POINT('Ctrl Pts',(0.0698239366988456,1.80655480211405,
1.5847793405579));
#24068=CARTESIAN_POINT('Ctrl Pts',(0.148691945288455,1.74187241700965,1.53343685544661));
#24069=CARTESIAN_POINT('Ctrl Pts',(0.274785130849249,1.59669345888594,1.42076782591243));
#24070=CARTESIAN_POINT('Ctrl Pts',(0.320436333138568,1.51444831269989,1.3583029222602));
#24071=CARTESIAN_POINT('Ctrl Pts',(0.36627106501613,1.35321270714143,1.23020598103185));
#24072=CARTESIAN_POINT('Ctrl Pts',(0.371649422530895,1.27957619027631,1.16961370091491));
#24073=CARTESIAN_POINT('Ctrl Pts',(0.364905277844141,1.20742290720348,1.10727038327973));
#24074=CARTESIAN_POINT('Origin',(0.,0.,1.10727038327973));
#24075=CARTESIAN_POINT('Ctrl Pts',(0.492368803403902,0.958722904333223,
1.28318567027397));
#24076=CARTESIAN_POINT('Ctrl Pts',(0.551909716442827,1.17966054547972,1.53751096017971));
#24077=CARTESIAN_POINT('Ctrl Pts',(0.47430114299954,1.3834695788885,1.74607168007007));
#24078=CARTESIAN_POINT('Ctrl Pts',(0.259543083074042,1.57015000455957,1.90886782994504));
#24079=CARTESIAN_POINT('Ctrl Pts',(0.497730308181424,0.97247283635693,1.26847940010162));
#24080=CARTESIAN_POINT('Ctrl Pts',(0.557797896845798,1.19651661813599,1.51987665322458));
#24081=CARTESIAN_POINT('Ctrl Pts',(0.47881626470797,1.40288697684033,1.72611612827483));
#24082=CARTESIAN_POINT('Ctrl Pts',(0.260856494176611,1.5918511796057,1.88704325648016));
#24083=CARTESIAN_POINT('Ctrl Pts',(0.510779460904231,0.996638068239397,
1.24117819097188));
#24084=CARTESIAN_POINT('Ctrl Pts',(0.572460097309863,1.2262773183014,1.48716579746039));
#24085=CARTESIAN_POINT('Ctrl Pts',(0.491635127338188,1.43799804358594,1.68888670640877));
#24086=CARTESIAN_POINT('Ctrl Pts',(0.268313724592168,1.63180052564182,1.84634350908917));
#24087=CARTESIAN_POINT('Ctrl Pts',(0.557803663431837,1.04217697649276,1.18072535874296));
#24088=CARTESIAN_POINT('Ctrl Pts',(0.627335597140059,1.28344787385866,1.41461088358276));
#24089=CARTESIAN_POINT('Ctrl Pts',(0.546077997260116,1.50844372983685,1.60644436926605));
#24090=CARTESIAN_POINT('Ctrl Pts',(0.314053900652136,1.71730828939987,1.75613814413928));
#24091=CARTESIAN_POINT('Ctrl Pts',(0.608738508149429,1.07063174084475,1.13430117558029));
#24092=CARTESIAN_POINT('Ctrl Pts',(0.687608854742563,1.32002833380447,1.35902160674437));
#24093=CARTESIAN_POINT('Ctrl Pts',(0.60891757097649,1.55649910176849,1.54332567193681));
#24094=CARTESIAN_POINT('Ctrl Pts',(0.372863601758246,1.78021953810235,1.68715809360677));
#24095=CARTESIAN_POINT('Ctrl Pts',(0.649605006049397,1.08812946536139,1.10192284729582));
#24096=CARTESIAN_POINT('Ctrl Pts',(0.736085457637466,1.34295142581461,1.32027771712105));
#24097=CARTESIAN_POINT('Ctrl Pts',(0.660325994321484,1.58796351671871,1.49933702411959));
#24098=CARTESIAN_POINT('Ctrl Pts',(0.422326616101449,1.82316573807366,1.63910076829142));
#24099=CARTESIAN_POINT('',(0.493314642657339,0.962275025729455,1.28727233489076));
#24100=CARTESIAN_POINT('',(0.642908916934723,1.08521613661244,1.10727038327973));
#24101=CARTESIAN_POINT('Ctrl Pts',(0.493314642657339,0.962275025729455,
1.28727233489076));
#24102=CARTESIAN_POINT('Ctrl Pts',(0.505155444617114,0.992714976575168,
1.2547827394338));
#24103=CARTESIAN_POINT('Ctrl Pts',(0.522900410114692,1.01347020049763,1.22829923781183));
#24104=CARTESIAN_POINT('Ctrl Pts',(0.572202237707941,1.0509553613877,1.17205963503352));
#24105=CARTESIAN_POINT('Ctrl Pts',(0.603178396560795,1.06919273067027,1.14130666672584));
#24106=CARTESIAN_POINT('Ctrl Pts',(0.642908916934723,1.08521613661244,1.10727038327973));
#24107=CARTESIAN_POINT('Ctrl Pts',(0.493314642657339,0.962275025729455,
1.28727233489076));
#24108=CARTESIAN_POINT('Ctrl Pts',(0.519074140629024,1.06019965524839,1.39987124007464));
#24109=CARTESIAN_POINT('Ctrl Pts',(0.517846241724568,1.15475382712427,1.50346488650363));
#24110=CARTESIAN_POINT('Ctrl Pts',(0.454602843714802,1.35913828497575,1.715480776583));
#24111=CARTESIAN_POINT('Ctrl Pts',(0.377981286365637,1.46714441944577,1.81902921434248));
#24112=CARTESIAN_POINT('Ctrl Pts',(0.259766273896474,1.5699559447672,1.90869858745619));
#24113=CARTESIAN_POINT('Ctrl Pts',(0.642908916934723,1.08521613661244,1.10727038327973));
#24114=CARTESIAN_POINT('Ctrl Pts',(0.668710261798007,1.16760035714814,1.18103565901043));
#24115=CARTESIAN_POINT('Ctrl Pts',(0.681355585835306,1.25518160519559,1.25302429310887));
#24116=CARTESIAN_POINT('Ctrl Pts',(0.665371573463983,1.44098614169386,1.39260788389875));
#24117=CARTESIAN_POINT('Ctrl Pts',(0.635301149560116,1.533892595955,1.45574709063858));
#24118=CARTESIAN_POINT('Ctrl Pts',(0.54169831056255,1.6923976184594,1.55895701082588));
#24119=CARTESIAN_POINT('Ctrl Pts',(0.489122861296305,1.75616935678547,1.5990490209941));
#24120=CARTESIAN_POINT('Ctrl Pts',(0.428377445609995,1.81394816223928,1.63615580822897));
#24121=CARTESIAN_POINT('Ctrl Pts',(0.362330138275325,1.21487793679796,1.10149705943222));
#24122=CARTESIAN_POINT('Ctrl Pts',(0.383459937582895,1.48329895916361,1.31979778023781));
#24123=CARTESIAN_POINT('Ctrl Pts',(0.24964496094192,1.70227260218965,1.49880741124997));
#24124=CARTESIAN_POINT('Ctrl Pts',(-0.0391147916476021,1.8717988658761,
1.63852595246867));
#24125=CARTESIAN_POINT('Ctrl Pts',(0.373447482460586,1.18333690797345,1.12583385309083));
#24126=CARTESIAN_POINT('Ctrl Pts',(0.398305182537801,1.44573672483851,1.34892944774502));
#24127=CARTESIAN_POINT('Ctrl Pts',(0.270675994878907,1.66212671668266,1.5318660237053));
#24128=CARTESIAN_POINT('Ctrl Pts',(-0.00930365130124667,1.83255854794258,
1.67464838892921));
#24129=CARTESIAN_POINT('Ctrl Pts',(0.386758017000779,1.13169790455625,1.16764044916317));
#24130=CARTESIAN_POINT('Ctrl Pts',(0.416680587119747,1.38402127269754,1.39897336709084));
#24131=CARTESIAN_POINT('Ctrl Pts',(0.298670375694659,1.59542335194444,1.58871211231352));
#24132=CARTESIAN_POINT('Ctrl Pts',(0.0327265383253287,1.76604232095016,
1.73676275687621));
#24133=CARTESIAN_POINT('Ctrl Pts',(0.391671741837559,1.06341115236232,1.22801607619329));
#24134=CARTESIAN_POINT('Ctrl Pts',(0.425665904909546,1.30168216224369,1.47139032317727));
#24135=CARTESIAN_POINT('Ctrl Pts',(0.318647566754322,1.50457544636211,1.67096220367119));
#24136=CARTESIAN_POINT('Ctrl Pts',(0.0706042875438467,1.67209124376878,
1.82672793765153));
#24137=CARTESIAN_POINT('Ctrl Pts',(0.38218165487343,1.0286884268729,1.263527751515));
#24138=CARTESIAN_POINT('Ctrl Pts',(0.415770412604395,1.25929056133869,1.51397381108002));
#24139=CARTESIAN_POINT('Ctrl Pts',(0.312692596804323,1.45588630034146,1.71945276482244));
#24140=CARTESIAN_POINT('Ctrl Pts',(0.0729619965738786,1.61878272768801,
1.8797604367197));
#24141=CARTESIAN_POINT('Ctrl Pts',(0.373486051297297,1.01098164381094,1.28318517919159));
#24142=CARTESIAN_POINT('Ctrl Pts',(0.40602648967972,1.23750736860246,1.53754499301511));
#24143=CARTESIAN_POINT('Ctrl Pts',(0.304436793685255,1.43052436008973,1.74612783237316));
#24144=CARTESIAN_POINT('Ctrl Pts',(0.0687169633139001,1.59003261827273,
1.90893369726573));
#24145=CARTESIAN_POINT('',(0.373997862975654,1.01462217612883,1.28727233489076));
#24146=CARTESIAN_POINT('Ctrl Pts',(0.364905277844141,1.20742290720348,1.10727038327973));
#24147=CARTESIAN_POINT('Ctrl Pts',(0.373615945090653,1.18311862080936,1.12801545944044));
#24148=CARTESIAN_POINT('Ctrl Pts',(0.381365818655247,1.15609247800031,1.15133239961422));
#24149=CARTESIAN_POINT('Ctrl Pts',(0.389206856698251,1.10715678825455,1.19509600545488));
#24150=CARTESIAN_POINT('Ctrl Pts',(0.390682503085348,1.08733497046199,1.21324740617447));
#24151=CARTESIAN_POINT('Ctrl Pts',(0.388091095569742,1.05408067239124,1.24538218411122));
#24152=CARTESIAN_POINT('Ctrl Pts',(0.384447468688942,1.03595219175479,1.26364457695038));
#24153=CARTESIAN_POINT('Ctrl Pts',(0.373997862975654,1.01462217612883,1.28727233489076));
#24154=CARTESIAN_POINT('Ctrl Pts',(0.373997862975654,1.01462217612883,1.28727233489076));
#24155=CARTESIAN_POINT('Ctrl Pts',(0.387792676785359,1.11493412912611,1.39987124007464));
#24156=CARTESIAN_POINT('Ctrl Pts',(0.375201374409042,1.20865423507634,1.50346488650363));
#24157=CARTESIAN_POINT('Ctrl Pts',(0.287835131123856,1.40394856048621,1.715480776583));
#24158=CARTESIAN_POINT('Ctrl Pts',(0.198779555753984,1.50195515531182,1.81902921434248));
#24159=CARTESIAN_POINT('Ctrl Pts',(0.0690572297370888,1.58980227845634,
1.90869858745619));
#24160=CARTESIAN_POINT('Ctrl Pts',(0.373997862975653,1.01462217612883,1.28727233489076));
#24161=CARTESIAN_POINT('Ctrl Pts',(0.405014516431692,1.24016643693111,1.54044292999952));
#24162=CARTESIAN_POINT('Ctrl Pts',(0.302637979515068,1.43238606966553,1.74808806061869));
#24163=CARTESIAN_POINT('Ctrl Pts',(0.0668682522257825,1.59128107433209,
1.91020772674828));
#24164=CARTESIAN_POINT('Ctrl Pts',(0.413770122869549,0.997173125995706,
1.28727233489076));
#24165=CARTESIAN_POINT('Ctrl Pts',(0.453754022216744,1.22092814469495,1.54044292999952));
#24166=CARTESIAN_POINT('Ctrl Pts',(0.359331486839601,1.41678703930426,1.74808806061869));
#24167=CARTESIAN_POINT('Ctrl Pts',(0.130502516738118,1.58474980982363,1.91020772674828));
#24168=CARTESIAN_POINT('Ctrl Pts',(0.453542382763444,0.97972407586258,1.28727233489076));
#24169=CARTESIAN_POINT('Ctrl Pts',(0.502493528001797,1.2016898524588,1.54044292999952));
#24170=CARTESIAN_POINT('Ctrl Pts',(0.416024994164134,1.40118800894299,1.74808806061869));
#24171=CARTESIAN_POINT('Ctrl Pts',(0.194136781250454,1.57821854531517,1.91020772674828));
#24172=CARTESIAN_POINT('Ctrl Pts',(0.493314642657339,0.962275025729455,
1.28727233489076));
#24173=CARTESIAN_POINT('Ctrl Pts',(0.55123303378685,1.18245156022264,1.54044292999952));
#24174=CARTESIAN_POINT('Ctrl Pts',(0.472718501488667,1.38558897858172,1.74808806061869));
#24175=CARTESIAN_POINT('Ctrl Pts',(0.257771045762789,1.5716872808067,1.91020772674828));
#24176=CARTESIAN_POINT('Ctrl Pts',(0.373997862975653,1.01462217612883,1.28727233489076));
#24177=CARTESIAN_POINT('Ctrl Pts',(0.394056488869171,1.00648281422349,1.28797191329047));
#24178=CARTESIAN_POINT('Ctrl Pts',(0.414003503730716,0.998068152324094,
1.28831907556383));
#24179=CARTESIAN_POINT('Ctrl Pts',(0.433838594404394,0.989370462098314,
1.288319084765));
#24180=CARTESIAN_POINT('Ctrl Pts',(0.453797800577664,0.980618347207408,
1.28831909402374));
#24181=CARTESIAN_POINT('Ctrl Pts',(0.473623504353529,0.971588455744707,
1.28796761487395));
#24182=CARTESIAN_POINT('Ctrl Pts',(0.493314642657339,0.962275025729455,
1.28727233489076));
#24183=CARTESIAN_POINT('Origin',(0.,0.,1.37171309575435));
#24184=CARTESIAN_POINT('',(0.720159740047642,1.03556549162895,1.10727038327973));
#24185=CARTESIAN_POINT('Ctrl Pts',(0.549562141057369,1.78098192700405,1.63615580822897));
#24186=CARTESIAN_POINT('Ctrl Pts',(0.620893161259242,1.70079633666882,1.58735805514603));
#24187=CARTESIAN_POINT('Ctrl Pts',(0.674133367258296,1.61925404078154,1.53858095020831));
#24188=CARTESIAN_POINT('Ctrl Pts',(0.751969574388259,1.44461319502357,1.42806953503212));
#24189=CARTESIAN_POINT('Ctrl Pts',(0.772017157909613,1.35007152673687,1.3646130604457));
#24190=CARTESIAN_POINT('Ctrl Pts',(0.767479006699498,1.17779635313149,1.23357020765531));
#24191=CARTESIAN_POINT('Ctrl Pts',(0.749676646324452,1.10397180136272,1.17136442658356));
#24192=CARTESIAN_POINT('Ctrl Pts',(0.720159740047642,1.03556549162895,1.10727038327973));
#24193=CARTESIAN_POINT('Origin',(0.,0.,1.10727038327973));
#24194=CARTESIAN_POINT('Ctrl Pts',(0.764532229233201,0.759649337735664,
1.28318567027397));
#24195=CARTESIAN_POINT('Ctrl Pts',(0.889432488376415,0.951374367053291,
1.53751096017971));
#24196=CARTESIAN_POINT('Ctrl Pts',(0.87860280381325,1.1691906444597,1.74607168007007));
#24197=CARTESIAN_POINT('Ctrl Pts',(0.732043175543707,1.4130981699549,1.90886782994504));
#24198=CARTESIAN_POINT('Ctrl Pts',(0.773880285955837,0.771069504093749,
1.26847940010162));
#24199=CARTESIAN_POINT('Ctrl Pts',(0.90024129362699,0.965585896981722,1.51987665322458));
#24200=CARTESIAN_POINT('Ctrl Pts',(0.888897245689574,1.18626243797171,1.72611612827484));
#24201=CARTESIAN_POINT('Ctrl Pts',(0.739998335618541,1.43333134754249,1.88704325648016));
#24202=CARTESIAN_POINT('Ctrl Pts',(0.793756470105422,0.790019380359273,
1.24117952306876));
#24203=CARTESIAN_POINT('Ctrl Pts',(0.923380672132907,0.989358920654668,
1.48716712955727));
#24204=CARTESIAN_POINT('Ctrl Pts',(0.911936310735741,1.2156928538318,1.68888851879237));
#24205=CARTESIAN_POINT('Ctrl Pts',(0.759433295933273,1.46902007592139,1.84634532147277));
#24206=CARTESIAN_POINT('Ctrl Pts',(0.852549487780079,0.818798433422949,
1.18072779772815));
#24207=CARTESIAN_POINT('Ctrl Pts',(0.993235093958044,1.02677414338758,1.41461332256794));
#24208=CARTESIAN_POINT('Ctrl Pts',(0.985480669746799,1.26586652272337,1.60644767971084));
#24209=CARTESIAN_POINT('Ctrl Pts',(0.829355339157893,1.53620791207526,1.75614145458407));
#24210=CARTESIAN_POINT('Ctrl Pts',(0.909788127533563,0.830120749534194,
1.13430117558029));
#24211=CARTESIAN_POINT('Ctrl Pts',(1.06186607016719,1.04293872696083,1.35902160674436));
#24212=CARTESIAN_POINT('Ctrl Pts',(1.06009969793962,1.29215273573923,1.54332567193682));
#24213=CARTESIAN_POINT('Ctrl Pts',(0.904732449133408,1.57786820262104,1.68715809360678));
#24214=CARTESIAN_POINT('Ctrl Pts',(0.954061570898026,0.834133632104406,
1.10192284729582));
#24215=CARTESIAN_POINT('Ctrl Pts',(1.115053684233,1.04975978886662,1.32027771712105));
#24216=CARTESIAN_POINT('Ctrl Pts',(1.11871505289201,1.30619109614142,1.49933702411959));
#24217=CARTESIAN_POINT('Ctrl Pts',(0.965045676875069,1.60342755392881,1.63910076829143));
#24218=CARTESIAN_POINT('',(0.766529441696069,0.762735325532963,1.28727233489076));
#24219=CARTESIAN_POINT('',(0.946792943618195,0.833432097145889,1.10727038327973));
#24220=CARTESIAN_POINT('Ctrl Pts',(0.766529441696069,0.762735325532963,
1.28727233489076));
#24221=CARTESIAN_POINT('Ctrl Pts',(0.787197175677519,0.788026430108106,
1.25478273943352));
#24222=CARTESIAN_POINT('Ctrl Pts',(0.81048735765961,0.8022823251633,1.22829923781154));
#24223=CARTESIAN_POINT('Ctrl Pts',(0.868959733809894,0.822697729112222,
1.17205963503275));
#24224=CARTESIAN_POINT('Ctrl Pts',(0.904055468577541,0.830470338502301,
1.14130666672531));
#24225=CARTESIAN_POINT('Ctrl Pts',(0.946792943618196,0.833432097145889,
1.10727038327973));
#24226=CARTESIAN_POINT('Ctrl Pts',(0.766529441696069,0.762735325532963,
1.28727233489076));
#24227=CARTESIAN_POINT('Ctrl Pts',(0.821288554787752,0.847907059902912,
1.39987124007464));
#24228=CARTESIAN_POINT('Ctrl Pts',(0.849339599532016,0.938212862837218,
1.50346488650363));
#24229=CARTESIAN_POINT('Ctrl Pts',(0.852349824604395,1.15213731807335,1.715480776583));
#24230=CARTESIAN_POINT('Ctrl Pts',(0.812854124246773,1.27853461941729,1.81902921434248));
#24231=CARTESIAN_POINT('Ctrl Pts',(0.732195474855993,1.41284463836769,1.90869858745619));
#24232=CARTESIAN_POINT('Ctrl Pts',(0.946792943618195,0.833432097145889,
1.10727038327973));
#24233=CARTESIAN_POINT('Ctrl Pts',(0.996789604993468,0.903811092885787,
1.18103565901043));
#24234=CARTESIAN_POINT('Ctrl Pts',(1.03588011685503,0.983198189519663,1.25302429310887));
#24235=CARTESIAN_POINT('Ctrl Pts',(1.07809517714267,1.16484813617459,1.39260788389875));
#24236=CARTESIAN_POINT('Ctrl Pts',(1.07820617779495,1.26249969691988,1.45574709063858));
#24237=CARTESIAN_POINT('Ctrl Pts',(1.03816533347023,1.44217179941018,1.55895701082588));
#24238=CARTESIAN_POINT('Ctrl Pts',(1.00786966075201,1.51906903401083,1.5990490209941));
#24239=CARTESIAN_POINT('Ctrl Pts',(0.967951970128401,1.59279130921887,1.63615580822897));
#24240=CARTESIAN_POINT('Ctrl Pts',(0.720016914634041,1.04334803864884,1.1015723109602));
#24241=CARTESIAN_POINT('Ctrl Pts',(0.823064346331371,1.29208090893697,1.31988785480614));
#24242=CARTESIAN_POINT('Ctrl Pts',(0.763481187915705,1.54167481933164,1.49890963328678));
#24243=CARTESIAN_POINT('Ctrl Pts',(0.541267439387044,1.79212976983285,1.63863764640212));
#24244=CARTESIAN_POINT('Ctrl Pts',(0.720837529677195,1.00993315330316,1.12589971949674));
#24245=CARTESIAN_POINT('Ctrl Pts',(0.825567715093924,1.25179094217684,1.34900830339197));
#24246=CARTESIAN_POINT('Ctrl Pts',(0.771065844731941,1.49701757504302,1.53195557707744));
#24247=CARTESIAN_POINT('Ctrl Pts',(0.557477346013133,1.74562013410096,1.67474624941237));
#24248=CARTESIAN_POINT('Ctrl Pts',(0.717530565095653,0.95673563332559,1.16769179538366));
#24249=CARTESIAN_POINT('Ctrl Pts',(0.823961384252209,1.18745042322669,1.39903449435103));
#24250=CARTESIAN_POINT('Ctrl Pts',(0.777060632929278,1.42496257773992,1.58878199846584));
#24251=CARTESIAN_POINT('Ctrl Pts',(0.576871348730713,1.66940588754283,1.73683890344255));
#24252=CARTESIAN_POINT('Ctrl Pts',(0.701101131459801,0.89030854064122,1.22804130170825));
#24253=CARTESIAN_POINT('Ctrl Pts',(0.807060009317124,1.10640797973512,1.47142017171286));
#24254=CARTESIAN_POINT('Ctrl Pts',(0.767978311363819,1.3324357381909,1.67099665961542));
#24255=CARTESIAN_POINT('Ctrl Pts',(0.583845206097281,1.56839818009429,1.82676536339562));
#24256=CARTESIAN_POINT('Ctrl Pts',(0.681352489183287,0.86023395370564,1.2635364344865));
#24257=CARTESIAN_POINT('Ctrl Pts',(0.784556163294565,1.06916866744103,1.51398418220583));
#24258=CARTESIAN_POINT('Ctrl Pts',(0.747275208483436,1.28799335847824,1.71946457116167));
#24259=CARTESIAN_POINT('Ctrl Pts',(0.569616647707433,1.51699586639173,1.87977332297456));
#24260=CARTESIAN_POINT('Ctrl Pts',(0.667616851769879,0.846087143187382,
1.28318517919043));
#24261=CARTESIAN_POINT('Ctrl Pts',(0.768564946360838,1.05147036139454,1.53754499301447));
#24262=CARTESIAN_POINT('Ctrl Pts',(0.731592934569706,1.26643337142018,1.7461278323729));
#24263=CARTESIAN_POINT('Ctrl Pts',(0.55670081639648,1.49097617326428,1.90893369726572));
#24264=CARTESIAN_POINT('',(0.669228599956957,0.849391336665505,1.28727233489076));
#24265=CARTESIAN_POINT('Ctrl Pts',(0.720159740047642,1.03556549162895,1.10727038327973));
#24266=CARTESIAN_POINT('Ctrl Pts',(0.720933639361785,1.00975899746822,1.12801545944058));
#24267=CARTESIAN_POINT('Ctrl Pts',(0.719952669695418,0.981660765603644,
1.15133239961438));
#24268=CARTESIAN_POINT('Ctrl Pts',(0.712287980257497,0.932697144980519,
1.19509600545699));
#24269=CARTESIAN_POINT('Ctrl Pts',(0.70756612481209,0.913389476193535,1.21324740617616));
#24270=CARTESIAN_POINT('Ctrl Pts',(0.694825406569049,0.882563548282451,
1.24538218411057));
#24271=CARTESIAN_POINT('Ctrl Pts',(0.685758102882491,0.866448281269836,
1.26364457694968));
#24272=CARTESIAN_POINT('Ctrl Pts',(0.669228599956957,0.849391336665505,
1.28727233489076));
#24273=CARTESIAN_POINT('Ctrl Pts',(0.669228599956957,0.849391336665505,
1.28727233489076));
#24274=CARTESIAN_POINT('Ctrl Pts',(0.713346345736856,0.940530841324424,
1.39987124007464));
#24275=CARTESIAN_POINT('Ctrl Pts',(0.73033241101646,1.03355488521186,1.50346488650363));
#24276=CARTESIAN_POINT('Ctrl Pts',(0.707591441492497,1.2462884798982,1.715480776583));
#24277=CARTESIAN_POINT('Ctrl Pts',(0.653180259586498,1.36701797678012,1.81902921434248));
#24278=CARTESIAN_POINT('Ctrl Pts',(0.55695325007777,1.49065195897357,1.90869858745619));
#24279=CARTESIAN_POINT('Ctrl Pts',(0.669228599956957,0.849391336665505,
1.28727233489076));
#24280=CARTESIAN_POINT('Ctrl Pts',(0.76842419991163,1.05431200258793,1.54044292999952));
#24281=CARTESIAN_POINT('Ctrl Pts',(0.73045746052879,1.26875982659235,1.74808806061869));
#24282=CARTESIAN_POINT('Ctrl Pts',(0.555328381808437,1.49273480867877,1.91020772674828));
#24283=CARTESIAN_POINT('Ctrl Pts',(0.701662213869994,0.820505999621324,
1.28727233489076));
#24284=CARTESIAN_POINT('Ctrl Pts',(0.808833265245786,1.02095396380933,1.54044292999952));
#24285=CARTESIAN_POINT('Ctrl Pts',(0.779555824624012,1.23640500988538,1.74808806061869));
#24286=CARTESIAN_POINT('Ctrl Pts',(0.613829892004671,1.46685913784949,1.91020772674828));
#24287=CARTESIAN_POINT('Ctrl Pts',(0.734095827783032,0.791620662577144,
1.28727233489076));
#24288=CARTESIAN_POINT('Ctrl Pts',(0.849242330579941,0.98759592503072,1.54044292999952));
#24289=CARTESIAN_POINT('Ctrl Pts',(0.828654188719232,1.20405019317841,1.74808806061869));
#24290=CARTESIAN_POINT('Ctrl Pts',(0.672331402200905,1.44098346702021,1.91020772674828));
#24291=CARTESIAN_POINT('Ctrl Pts',(0.766529441696069,0.762735325532963,
1.28727233489076));
#24292=CARTESIAN_POINT('Ctrl Pts',(0.889651395914097,0.954237886252115,
1.54044292999952));
#24293=CARTESIAN_POINT('Ctrl Pts',(0.877752552814453,1.17169537647143,1.74808806061869));
#24294=CARTESIAN_POINT('Ctrl Pts',(0.730832912397138,1.41510779619092,1.91020772674828));
#24295=CARTESIAN_POINT('Ctrl Pts',(0.669228599956957,0.849391336665505,
1.28727233489076));
#24296=CARTESIAN_POINT('Ctrl Pts',(0.685790285668792,0.835451887202042,
1.28797191329046));
#24297=CARTESIAN_POINT('Ctrl Pts',(0.702160750604669,0.821285101590933,
1.28831907556383));
#24298=CARTESIAN_POINT('Ctrl Pts',(0.718337308749603,0.806883726521852,
1.288319084765));
#24299=CARTESIAN_POINT('Ctrl Pts',(0.73461508960276,0.792392236721716,1.28831909402374));
#24300=CARTESIAN_POINT('Ctrl Pts',(0.7506800644496,0.777677820212488,1.28796761487395));
#24301=CARTESIAN_POINT('Ctrl Pts',(0.766529441696069,0.762735325532963,
1.28727233489076));
#24302=CARTESIAN_POINT('Origin',(0.,0.,1.37171309575435));
#24303=CARTESIAN_POINT('',(1.00491994924733,0.762339710524744,1.10727038327973));
#24304=CARTESIAN_POINT('Ctrl Pts',(1.07301833748062,1.52399042602929,1.63615580822897));
#24305=CARTESIAN_POINT('Ctrl Pts',(1.11607945893996,1.42568690035965,1.5873580551461));
#24306=CARTESIAN_POINT('Ctrl Pts',(1.14151594859478,1.33168344006466,1.53858095020839));
#24307=CARTESIAN_POINT('Ctrl Pts',(1.16157559133822,1.1415374149143,1.42806953503215));
#24308=CARTESIAN_POINT('Ctrl Pts',(1.15142699410503,1.04542790122456,1.36461306044572));
#24309=CARTESIAN_POINT('Ctrl Pts',(1.09387499947176,0.882986840618232,1.23357020765532));
#24310=CARTESIAN_POINT('Ctrl Pts',(1.05413090753298,0.818276751491846,1.17136442658356));
#24311=CARTESIAN_POINT('Ctrl Pts',(1.00491994924733,0.762339710524743,1.10727038327973));
#24312=CARTESIAN_POINT('Origin',(0.,0.,1.10727038327973));
#24313=CARTESIAN_POINT('Ctrl Pts',(0.96185791365589,0.486216001172379,1.28318567027397));
#24314=CARTESIAN_POINT('Ctrl Pts',(1.13989141130718,0.629961036964703,1.53751096017972));
#24315=CARTESIAN_POINT('Ctrl Pts',(1.19690070060403,0.840463183520968,1.74607168007008));
#24316=CARTESIAN_POINT('Ctrl Pts',(1.13288578154644,1.11772244084117,1.90886782994505));
#24317=CARTESIAN_POINT('Ctrl Pts',(0.974277469399888,0.494188516412736,
1.26847940010162));
#24318=CARTESIAN_POINT('Ctrl Pts',(1.15456280023806,0.640136900598344,1.51987665322459));
#24319=CARTESIAN_POINT('Ctrl Pts',(1.2119667709518,0.853518266498017,1.72611612827485));
#24320=CARTESIAN_POINT('Ctrl Pts',(1.14670398409855,1.13450705657511,1.88704325648017));
#24321=CARTESIAN_POINT('Ctrl Pts',(0.999036317271857,0.506068912121109,
1.24117979784214));
#24322=CARTESIAN_POINT('Ctrl Pts',(1.18391556488183,0.655595999565544,1.48716740433065));
#24323=CARTESIAN_POINT('Ctrl Pts',(1.24297220725902,0.874388755352329,1.68888889262423));
#24324=CARTESIAN_POINT('Ctrl Pts',(1.17621563803994,1.16244328394297,1.84634569530463));
#24325=CARTESIAN_POINT('Ctrl Pts',(1.06384465023929,0.515271549474755,1.18072830092663));
#24326=CARTESIAN_POINT('Ctrl Pts',(1.26191264154005,0.669593960494798,1.41461382576643));
#24327=CARTESIAN_POINT('Ctrl Pts',(1.32842099300984,0.89938039390582,1.60644836271615));
#24328=CARTESIAN_POINT('Ctrl Pts',(1.26347706358719,1.20473571427761,1.75614213758938));
#24329=CARTESIAN_POINT('Ctrl Pts',(1.1217813461281,0.508351755467879,1.13430117558029));
#24330=CARTESIAN_POINT('Ctrl Pts',(1.33218043618791,0.663759010940873,1.35902160674437));
#24331=CARTESIAN_POINT('Ctrl Pts',(1.4075118803195,0.901321456978326,1.54332567193682));
#24332=CARTESIAN_POINT('Ctrl Pts',(1.34803978074575,1.22106413381299,1.68715809360678));
#24333=CARTESIAN_POINT('Ctrl Pts',(1.16512794184932,0.498486987186291,1.10192284729582));
#24334=CARTESIAN_POINT('Ctrl Pts',(1.38487268717996,0.653810349677836,1.32027771712106));
#24335=CARTESIAN_POINT('Ctrl Pts',(1.46759648753937,0.896559590305322,1.4993370241196));
#24336=CARTESIAN_POINT('Ctrl Pts',(1.41329934292755,1.22673470906875,1.63910076829144));
#24337=CARTESIAN_POINT('',(0.964710998256926,0.488533777383804,1.28727233489076));
#24338=CARTESIAN_POINT('',(1.15799828028599,0.500065917147829,1.10727038327973));
#24339=CARTESIAN_POINT('Ctrl Pts',(0.964710998256926,0.488533777383804,
1.28727233489076));
#24340=CARTESIAN_POINT('Ctrl Pts',(0.992182562456677,0.506200366158425,
1.25478273943422));
#24341=CARTESIAN_POINT('Ctrl Pts',(1.01873815563839,0.512561466012053,1.22829923781222));
#24342=CARTESIAN_POINT('Ctrl Pts',(1.08065739676596,0.513908711038628,1.172059635034));
#24343=CARTESIAN_POINT('Ctrl Pts',(1.11643729240337,0.510455723374658,1.14130666672621));
#24344=CARTESIAN_POINT('Ctrl Pts',(1.15799828028599,0.500065917147829,1.10727038327973));
#24345=CARTESIAN_POINT('Ctrl Pts',(0.964710998256926,0.488533777383804,
1.28727233489076));
#24346=CARTESIAN_POINT('Ctrl Pts',(1.04310952295002,0.552615413818275,1.39987124007464));
#24347=CARTESIAN_POINT('Ctrl Pts',(1.09769367964031,0.629833086622262,1.50346488650363));
#24348=CARTESIAN_POINT('Ctrl Pts',(1.16666286599128,0.832357123065218,1.715480776583));
#24349=CARTESIAN_POINT('Ctrl Pts',(1.16815913695893,0.964772942765737,1.81902921434248));
#24350=CARTESIAN_POINT('Ctrl Pts',(1.13295228123076,1.11743425489732,1.90869858745619));
#24351=CARTESIAN_POINT('Ctrl Pts',(1.15799828028599,0.500065917147829,1.10727038327973));
#24352=CARTESIAN_POINT('Ctrl Pts',(1.22729623661065,0.55155050162963,1.18103565901047));
#24353=CARTESIAN_POINT('Ctrl Pts',(1.28900548463589,0.61497248470904,1.25302429310896));
#24354=CARTESIAN_POINT('Ctrl Pts',(1.38528731335191,0.774686679112512,1.39260788389887));
#24355=CARTESIAN_POINT('Ctrl Pts',(1.41556887304308,0.867524531197783,1.45574709063869));
#24356=CARTESIAN_POINT('Ctrl Pts',(1.43300950021463,1.05077615643305,1.55895701082594));
#24357=CARTESIAN_POINT('Ctrl Pts',(1.42795915557246,1.13327165021096,1.59904902099413));
#24358=CARTESIAN_POINT('Ctrl Pts',(1.4127766116927,1.21572094522251,1.63615580822897));
#24359=CARTESIAN_POINT('Ctrl Pts',(1.0071890534957,0.769785488061409,1.10157231096021));
#24360=CARTESIAN_POINT('Ctrl Pts',(1.18205566887762,0.97450109754457,1.31988785480615));
#24361=CARTESIAN_POINT('Ctrl Pts',(1.2025174778094,1.23029122098199,1.4989096332868));
#24362=CARTESIAN_POINT('Ctrl Pts',(1.06857448029104,1.53715585837368,1.63863764640214));
#24363=CARTESIAN_POINT('Ctrl Pts',(0.997643737342948,0.737752459617965,
1.12589971949674));
#24364=CARTESIAN_POINT('Ctrl Pts',(1.17198622962025,0.935409478625221,1.34900830339198));
#24365=CARTESIAN_POINT('Ctrl Pts',(1.19593106769121,1.1854758699488,1.53195557707745));
#24366=CARTESIAN_POINT('Ctrl Pts',(1.06961874977298,1.48791342961567,1.67474624941239));
#24367=CARTESIAN_POINT('Ctrl Pts',(0.978058304401187,0.688180702732142,
1.1676928969232));
#24368=CARTESIAN_POINT('Ctrl Pts',(1.15057481942775,0.874714575228634,1.39903559589058));
#24369=CARTESIAN_POINT('Ctrl Pts',(1.17936426310359,1.11509475695032,1.58878350409041));
#24370=CARTESIAN_POINT('Ctrl Pts',(1.06451007676443,1.40943605051226,1.73684040906712));
#24371=CARTESIAN_POINT('Ctrl Pts',(0.941905889318168,0.63008137483939,1.22804259109412));
#24372=CARTESIAN_POINT('Ctrl Pts',(1.10945716971861,0.802861060594562,1.47142146109874));
#24373=CARTESIAN_POINT('Ctrl Pts',(1.14213429484135,1.02990257473199,1.6709984207319));
#24374=CARTESIAN_POINT('Ctrl Pts',(1.0399297097943,1.31121645145953,1.8267671245121));
#24375=CARTESIAN_POINT('Ctrl Pts',(0.913831635565082,0.607581608892784,
1.2635364344865));
#24376=CARTESIAN_POINT('Ctrl Pts',(1.07654853959332,0.77439864068878,1.51398418220584));
#24377=CARTESIAN_POINT('Ctrl Pts',(1.10871279290583,0.994033737629162,1.71946457116168));
#24378=CARTESIAN_POINT('Ctrl Pts',(1.01051512770394,1.26672757950422,1.87977332297458));
#24379=CARTESIAN_POINT('Ctrl Pts',(0.89639666323125,0.598371737953918,1.28318517919043));
#24380=CARTESIAN_POINT('Ctrl Pts',(1.055870911185,0.762508109189138,1.53754499301448));
#24381=CARTESIAN_POINT('Ctrl Pts',(1.08713566171041,0.978375060596136,1.74612783237292));
#24382=CARTESIAN_POINT('Ctrl Pts',(0.990190914807483,1.24597259217491,1.90893369726574));
#24383=CARTESIAN_POINT('',(0.89895057878464,0.601016155111926,1.28727233489076));
#24384=CARTESIAN_POINT('Ctrl Pts',(1.00491994924733,0.762339710524744,1.10727038327973));
#24385=CARTESIAN_POINT('Ctrl Pts',(0.997681325972119,0.737557128050518,
1.12801545944052));
#24386=CARTESIAN_POINT('Ctrl Pts',(0.988065537220638,0.71113725783727,1.15133239961424));
#24387=CARTESIAN_POINT('Ctrl Pts',(0.965645393507445,0.666938606676742,
1.19509600545531));
#24388=CARTESIAN_POINT('Ctrl Pts',(0.955188244340171,0.650035056039365,
1.21324740617484));
#24389=CARTESIAN_POINT('Ctrl Pts',(0.933545365639553,0.624654954884687,
1.24538218411132));
#24390=CARTESIAN_POINT('Ctrl Pts',(0.919941956007271,0.612130376113047,
1.26364457695043));
#24391=CARTESIAN_POINT('Ctrl Pts',(0.89895057878464,0.601016155111926,1.28727233489076));
#24392=CARTESIAN_POINT('Ctrl Pts',(0.89895057878464,0.601016155111926,1.28727233489076));
#24393=CARTESIAN_POINT('Ctrl Pts',(0.969072704191387,0.674061841710201,
1.39987124007464));
#24394=CARTESIAN_POINT('Ctrl Pts',(1.01397342270847,0.757283981982513,1.50346488650363));
#24395=CARTESIAN_POINT('Ctrl Pts',(1.05808377148838,0.966632999495317,1.715480776583));
#24396=CARTESIAN_POINT('Ctrl Pts',(1.04364312863621,1.09826755410688,1.81902921434248));
#24397=CARTESIAN_POINT('Ctrl Pts',(0.990330805779366,1.24558623976355,1.90869858745619));
#24398=CARTESIAN_POINT('Ctrl Pts',(0.89895057878464,0.601016155111926,1.28727233489076));
#24399=CARTESIAN_POINT('Ctrl Pts',(1.056615168778,0.76525416360778,1.54044292999951));
#24400=CARTESIAN_POINT('Ctrl Pts',(1.08677467590956,0.980938531722803,1.74808806061869));
#24401=CARTESIAN_POINT('Ctrl Pts',(0.989429100179332,1.248069259457,1.91020772674828));
#24402=CARTESIAN_POINT('Ctrl Pts',(0.920870718608735,0.563522029202552,
1.28727233489076));
#24403=CARTESIAN_POINT('Ctrl Pts',(1.08473827279984,0.721041695541498,1.54044292999952));
#24404=CARTESIAN_POINT('Ctrl Pts',(1.12347180680941,0.934995043558669,1.74808806061869));
#24405=CARTESIAN_POINT('Ctrl Pts',(1.03707132063747,1.20538207325406,1.91020772674828));
#24406=CARTESIAN_POINT('Ctrl Pts',(0.94279085843283,0.526027903293178,1.28727233489076));
#24407=CARTESIAN_POINT('Ctrl Pts',(1.11286137682168,0.676829227475218,1.54044292999952));
#24408=CARTESIAN_POINT('Ctrl Pts',(1.16016893770927,0.889051555394535,1.74808806061869));
#24409=CARTESIAN_POINT('Ctrl Pts',(1.0847135410956,1.16269488705113,1.91020772674828));
#24410=CARTESIAN_POINT('Ctrl Pts',(0.964710998256926,0.488533777383804,
1.28727233489076));
#24411=CARTESIAN_POINT('Ctrl Pts',(1.14098448084351,0.632616759408936,1.54044292999951));
#24412=CARTESIAN_POINT('Ctrl Pts',(1.19686606860912,0.843108067230401,1.74808806061869));
#24413=CARTESIAN_POINT('Ctrl Pts',(1.13235576155374,1.1200077008482,1.91020772674828));
#24414=CARTESIAN_POINT('Ctrl Pts',(0.89895057878464,0.601016155111926,1.28727233489076));
#24415=CARTESIAN_POINT('Ctrl Pts',(0.910394151125278,0.582641108525671,
1.28797191329047));
#24416=CARTESIAN_POINT('Ctrl Pts',(0.921585610967822,0.564108942884268,
1.28831907556383));
#24417=CARTESIAN_POINT('Ctrl Pts',(0.932520162364073,0.545413589903933,
1.288319084765));
#24418=CARTESIAN_POINT('Ctrl Pts',(0.943523135293241,0.52660125318435,1.28831909402374));
#24419=CARTESIAN_POINT('Ctrl Pts',(0.954254829541784,0.507642661237886,
1.28796761487395));
#24420=CARTESIAN_POINT('Ctrl Pts',(0.964710998256926,0.488533777383804,
1.28727233489076));
#24421=CARTESIAN_POINT('Origin',(0.,0.,1.37171309575435));
#24422=CARTESIAN_POINT('',(1.19131159212569,0.414490807021285,1.10727038327973));
#24423=CARTESIAN_POINT('Ctrl Pts',(1.4914400228729,1.11782012388912,1.63615580822897));
#24424=CARTESIAN_POINT('Ctrl Pts',(1.5020161229969,1.01102129689834,1.58735805514606));
#24425=CARTESIAN_POINT('Ctrl Pts',(1.49715899547356,0.913758385849943,1.53858095020834));
#24426=CARTESIAN_POINT('Ctrl Pts',(1.45747849623498,0.726719999074329,1.42806953503215));
#24427=CARTESIAN_POINT('Ctrl Pts',(1.41812713365386,0.638450508815867,1.36461306044572));
#24428=CARTESIAN_POINT('Ctrl Pts',(1.31319488582046,0.501744424014179,1.23357020765532));
#24429=CARTESIAN_POINT('Ctrl Pts',(1.25539949095026,0.452483071915572,1.17136442658356));
#24430=CARTESIAN_POINT('Ctrl Pts',(1.19131159212569,0.414490807021284,1.10727038327973));
#24431=CARTESIAN_POINT('Origin',(0.,0.,1.10727038327973));
#24432=CARTESIAN_POINT('Ctrl Pts',(1.19577051030242,0.420870970491663,1.1015723109602));
#24433=CARTESIAN_POINT('Ctrl Pts',(1.42533914668799,0.561530328976111,1.31988785480614));
#24434=CARTESIAN_POINT('Ctrl Pts',(1.52384297854318,0.798478145979632,1.49890963328678));
#24435=CARTESIAN_POINT('Ctrl Pts',(1.49128200586798,1.13171442150222,1.63863764640213));
#24436=CARTESIAN_POINT('Ctrl Pts',(1.17679362500493,0.393355414961738,1.12589971949673));
#24437=CARTESIAN_POINT('Ctrl Pts',(1.40368256628313,0.527463617924691,1.34900830339197));
#24438=CARTESIAN_POINT('Ctrl Pts',(1.50373022520314,0.7578915270079,1.53195557707743));
#24439=CARTESIAN_POINT('Ctrl Pts',(1.47705841783302,1.08455939173708,1.67474624941237));
#24440=CARTESIAN_POINT('Ctrl Pts',(1.14284817765567,0.352262141476103,1.16769296545954));
#24441=CARTESIAN_POINT('Ctrl Pts',(1.36456327006819,0.476355861470107,1.39903566442691));
#24442=CARTESIAN_POINT('Ctrl Pts',(1.466225176644,0.696074558068182,1.58878359776798));
#24443=CARTESIAN_POINT('Ctrl Pts',(1.44794881615932,1.01150165877889,1.73684050274469));
#24444=CARTESIAN_POINT('Ctrl Pts',(1.09051150146367,0.30817808510559,1.22804267083047));
#24445=CARTESIAN_POINT('Ctrl Pts',(1.30325409768321,0.420725138053454,1.47142154083508));
#24446=CARTESIAN_POINT('Ctrl Pts',(1.40449154295595,0.626556636662132,1.67099852964048));
#24447=CARTESIAN_POINT('Ctrl Pts',(1.39421997501402,0.925684985930674,1.82676723342069));
#24448=CARTESIAN_POINT('Ctrl Pts',(1.05685857441837,0.295454942931511,1.2635364344865));
#24449=CARTESIAN_POINT('Ctrl Pts',(1.26316084408195,0.403825079433301,1.51398418220583));
#24450=CARTESIAN_POINT('Ctrl Pts',(1.36162184430235,0.602771168700615,1.71946457116167));
#24451=CARTESIAN_POINT('Ctrl Pts',(1.35249734632791,0.892463171324756,1.87977332297457));
#24452=CARTESIAN_POINT('Ctrl Pts',(1.03743092373275,0.292083537908477,1.28318517919043));
#24453=CARTESIAN_POINT('Ctrl Pts',(1.23982087453714,0.398906250549898,1.53754499301447));
#24454=CARTESIAN_POINT('Ctrl Pts',(1.33626197576335,0.594546582101038,1.7461278323729));
#24455=CARTESIAN_POINT('Ctrl Pts',(1.32675422741137,0.879004532561896,1.90893369726572));
#24456=CARTESIAN_POINT('',(1.04067701160391,0.293809324770207,1.28727233489076));
#24457=CARTESIAN_POINT('Ctrl Pts',(1.04067701160391,0.293809324770207,1.28727233489076));
#24458=CARTESIAN_POINT('Ctrl Pts',(1.12993947443311,0.341610972564374,1.39987124007464));
#24459=CARTESIAN_POINT('Ctrl Pts',(1.19835965101752,0.406884846288962,1.50346488650363));
#24460=CARTESIAN_POINT('Ctrl Pts',(1.30500348982786,0.592356746173702,1.715480776583));
#24461=CARTESIAN_POINT('Ctrl Pts',(1.33194693676576,0.722011051157661,1.81902921434248));
#24462=CARTESIAN_POINT('Ctrl Pts',(1.32676788217082,0.878593860895847,1.90869858745619));
#24463=CARTESIAN_POINT('Ctrl Pts',(1.19131159212569,0.414490807021285,1.10727038327973));
#24464=CARTESIAN_POINT('Ctrl Pts',(1.17676901314193,0.393158028076719,1.12801545944028));
#24465=CARTESIAN_POINT('Ctrl Pts',(1.15945966570543,0.371002680489165,1.15133239961405));
#24466=CARTESIAN_POINT('Ctrl Pts',(1.12447870759406,0.335895470715595,1.19509600545462));
#24467=CARTESIAN_POINT('Ctrl Pts',(1.10930988332456,0.323050675538658,1.21324740617407));
#24468=CARTESIAN_POINT('Ctrl Pts',(1.08088339992896,0.305600782276809,1.24538218411082));
#24469=CARTESIAN_POINT('Ctrl Pts',(1.06407548086649,0.297892884779809,1.26364457695002));
#24470=CARTESIAN_POINT('Ctrl Pts',(1.04067701160391,0.293809324770207,1.28727233489076));
#24471=CARTESIAN_POINT('Ctrl Pts',(1.04067701160391,0.293809324770207,1.28727233489076));
#24472=CARTESIAN_POINT('Ctrl Pts',(1.24137728305361,0.401287915254421,1.54044292999952));
#24473=CARTESIAN_POINT('Ctrl Pts',(1.3367108140079,0.59709613876759,1.74808806061869));
#24474=CARTESIAN_POINT('Ctrl Pts',(1.32667760446677,0.881233995309716,1.91020772674828));
#24475=CARTESIAN_POINT('Ctrl Pts',(1.04993798132648,0.251376596276585,1.28727233489076));
#24476=CARTESIAN_POINT('Ctrl Pts',(1.25446154039628,0.35054884232117,1.54044292999952));
#24477=CARTESIAN_POINT('Ctrl Pts',(1.35741454085596,0.542061247874906,1.74808806061869));
#24478=CARTESIAN_POINT('Ctrl Pts',(1.3587969827055,0.825913812937791,1.91020772674828));
#24479=CARTESIAN_POINT('Ctrl Pts',(1.05919895104906,0.208943867782964,1.28727233489076));
#24480=CARTESIAN_POINT('Ctrl Pts',(1.26754579773896,0.29980976938792,1.54044292999952));
#24481=CARTESIAN_POINT('Ctrl Pts',(1.37811826770401,0.487026356982221,1.74808806061869));
#24482=CARTESIAN_POINT('Ctrl Pts',(1.39091636094422,0.770593630565866,1.91020772674828));
#24483=CARTESIAN_POINT('Ctrl Pts',(1.06845992077163,0.166511139289342,1.28727233489076));
#24484=CARTESIAN_POINT('Ctrl Pts',(1.28063005508163,0.24907069645467,1.54044292999952));
#24485=CARTESIAN_POINT('Ctrl Pts',(1.39882199455207,0.431991466089536,1.74808806061869));
#24486=CARTESIAN_POINT('Ctrl Pts',(1.42303573918295,0.715273448193941,1.91020772674828));
#24487=CARTESIAN_POINT('',(1.06845992077163,0.166511139289342,1.28727233489076));
#24488=CARTESIAN_POINT('Ctrl Pts',(1.06845992077163,0.166511139289342,1.28727233489076));
#24489=CARTESIAN_POINT('Ctrl Pts',(1.16282366323453,0.203229920731113,1.39987124007464));
#24490=CARTESIAN_POINT('Ctrl Pts',(1.23859785430383,0.259800859583567,1.50346488650363));
#24491=CARTESIAN_POINT('Ctrl Pts',(1.36677481743678,0.431100013478375,1.715480776583));
#24492=CARTESIAN_POINT('Ctrl Pts',(1.40911659430226,0.556572568507924,1.81902921434248));
#24493=CARTESIAN_POINT('Ctrl Pts',(1.42280782457595,0.712641620935351,1.90869858745619));
#24494=CARTESIAN_POINT('Ctrl Pts',(1.04067701160391,0.293809324770207,1.28727233489076));
#24495=CARTESIAN_POINT('Ctrl Pts',(1.04588229398058,0.272797358647518,1.28797191329046));
#24496=CARTESIAN_POINT('Ctrl Pts',(1.05079925066492,0.251713870469983,1.28831907556383));
#24497=CARTESIAN_POINT('Ctrl Pts',(1.05542144523633,0.230554570986284,1.288319084765));
#24498=CARTESIAN_POINT('Ctrl Pts',(1.06007256258898,0.209262869938632,1.28831909402374));
#24499=CARTESIAN_POINT('Ctrl Pts',(1.06442048323406,0.187915901626936,1.28796761487395));
#24500=CARTESIAN_POINT('Ctrl Pts',(1.06845992077163,0.166511139289342,1.28727233489076));
#24501=CARTESIAN_POINT('Ctrl Pts',(1.06503024383179,0.165188454748262,1.28318567027397));
#24502=CARTESIAN_POINT('Ctrl Pts',(1.27876982080873,0.24688273138137,1.53751096017972));
#24503=CARTESIAN_POINT('Ctrl Pts',(1.39803761752215,0.429465330327861,1.74607168007008));
#24504=CARTESIAN_POINT('Ctrl Pts',(1.42283363397204,0.712936251587734,1.90886782994506));
#24505=CARTESIAN_POINT('Ctrl Pts',(1.07930558594879,0.168932913531384,1.26847940010162));
#24506=CARTESIAN_POINT('Ctrl Pts',(1.29586765564979,0.25202684428835,1.51987665322459));
#24507=CARTESIAN_POINT('Ctrl Pts',(1.41640054440424,0.437225780288049,1.72611612827485));
#24508=CARTESIAN_POINT('Ctrl Pts',(1.44116225705855,0.724629310334688,1.88704325648017));
#24509=CARTESIAN_POINT('Ctrl Pts',(1.10652474870094,0.172580460092753,1.24117906537517));
#24510=CARTESIAN_POINT('Ctrl Pts',(1.32856177300787,0.257658341550684,1.48716667186368));
#24511=CARTESIAN_POINT('Ctrl Pts',(1.45233913898617,0.447493258920483,1.6888878960876));
#24512=CARTESIAN_POINT('Ctrl Pts',(1.47786361346603,0.742078309759803,1.84634469876801));
#24513=CARTESIAN_POINT('Ctrl Pts',(1.171005693206,0.161305070542798,1.18072695962338));
#24514=CARTESIAN_POINT('Ctrl Pts',(1.40706779462019,0.246868029800146,1.41461248446319));
#24515=CARTESIAN_POINT('Ctrl Pts',(1.54132997390971,0.444855864337703,1.60644654213684));
#24516=CARTESIAN_POINT('Ctrl Pts',(1.57392460995617,0.755334809435779,1.75614031701006));
#24517=CARTESIAN_POINT('Ctrl Pts',(1.22396679065338,0.13682174968142,1.13430117558029));
#24518=CARTESIAN_POINT('Ctrl Pts',(1.47209169926766,0.21960593824905,1.35902160674437));
#24519=CARTESIAN_POINT('Ctrl Pts',(1.6171469931418,0.422262554132517,1.54332567193682));
#24520=CARTESIAN_POINT('Ctrl Pts',(1.65939158627328,0.744733799933235,1.68715809360678));
#24521=CARTESIAN_POINT('Ctrl Pts',(1.26214347192869,0.114044962799315,1.10192284729582));
#24522=CARTESIAN_POINT('Ctrl Pts',(1.51913070253036,0.193861398098012,1.32027771712106));
#24523=CARTESIAN_POINT('Ctrl Pts',(1.67281935264038,0.399166585072146,1.4993370241196));
#24524=CARTESIAN_POINT('Ctrl Pts',(1.72320942225876,0.729960523721717,1.63910076829144));
#24525=CARTESIAN_POINT('',(1.25585067703094,0.117749801015222,1.10727038327973));
#24526=CARTESIAN_POINT('Ctrl Pts',(1.25585067703094,0.117749801015222,1.10727038327973));
#24527=CARTESIAN_POINT('Ctrl Pts',(1.33766656151264,0.145300304395604,1.18103565901045));
#24528=CARTESIAN_POINT('Ctrl Pts',(1.4159540145512,0.186548988329726,1.25302429310892));
#24529=CARTESIAN_POINT('Ctrl Pts',(1.55687787546595,0.308693492339194,1.39260788389881));
#24530=CARTESIAN_POINT('Ctrl Pts',(1.61436582414944,0.387630019962978,1.45574709063864));
#24531=CARTESIAN_POINT('Ctrl Pts',(1.68758071271377,0.556523222076105,1.55895701082591));
#24532=CARTESIAN_POINT('Ctrl Pts',(1.70827005906903,0.636541741320481,1.59904902099412));
#24533=CARTESIAN_POINT('Ctrl Pts',(1.71930883511106,0.71964734468187,1.63615580822897));
#24534=CARTESIAN_POINT('Ctrl Pts',(1.06845992077163,0.166511139289342,1.28727233489076));
#24535=CARTESIAN_POINT('Ctrl Pts',(1.10004620708046,0.174823883464324,1.25478273943439));
#24536=CARTESIAN_POINT('Ctrl Pts',(1.12726776497768,0.172667519342153,1.22829923781239));
#24537=CARTESIAN_POINT('Ctrl Pts',(1.18657278434634,0.154814727716086,1.17205963503281));
#24538=CARTESIAN_POINT('Ctrl Pts',(1.21953445537525,0.14047414548817,1.14130666672491));
#24539=CARTESIAN_POINT('Ctrl Pts',(1.25585067703094,0.117749801015222,1.10727038327973));
#24540=CARTESIAN_POINT('Ctrl Pts',(1.2673016181377,0.0307586699497107,1.1015723109602));
#24541=CARTESIAN_POINT('Ctrl Pts',(1.52910049789877,0.0935930593956198,
1.31988785480615));
#24542=CARTESIAN_POINT('Ctrl Pts',(1.69600411129882,0.288504466724436,1.49890963328679));
#24543=CARTESIAN_POINT('Ctrl Pts',(1.76801245833786,0.615492891936159,1.63863764640214));
#24544=CARTESIAN_POINT('Ctrl Pts',(1.23190046521827,0.00368577884439299,
1.13400885567558));
#24545=CARTESIAN_POINT('Ctrl Pts',(1.48760761670895,0.0593992442947171,
1.35870212368824));
#24546=CARTESIAN_POINT('Ctrl Pts',(1.65386565639404,0.245271053169412,1.54297833728479));
#24547=CARTESIAN_POINT('Ctrl Pts',(1.73054693613328,0.56155720138891,1.6867824504158));
#24548=CARTESIAN_POINT('Ctrl Pts',(1.18197455396454,-0.0267745014609978,
1.18052159225508));
#24549=CARTESIAN_POINT('Ctrl Pts',(1.42871036910363,0.0203421811660883,
1.41439816169908));
#24550=CARTESIAN_POINT('Ctrl Pts',(1.59277760615935,0.194600327489428,1.60621915369239));
#24551=CARTESIAN_POINT('Ctrl Pts',(1.67419193839781,0.496164143986696,1.75589578968676));
#24552=CARTESIAN_POINT('Ctrl Pts',(1.11906265670396,-0.0454087437059702,
1.24109759607728));
#24553=CARTESIAN_POINT('Ctrl Pts',(1.35343612743123,-0.00502457427851058,
1.48710236189544));
#24554=CARTESIAN_POINT('Ctrl Pts',(1.51172442238932,0.157227158096703,1.68883153964047));
#24555=CARTESIAN_POINT('Ctrl Pts',(1.59391973364072,0.441350654339689,1.84628730593333));
#24556=CARTESIAN_POINT('Ctrl Pts',(1.09155317863394,-0.0448936420229278,
1.26844862066248));
#24557=CARTESIAN_POINT('Ctrl Pts',(1.32019136139833,-0.00558636246918835,
1.51987386218776));
#24558=CARTESIAN_POINT('Ctrl Pts',(1.47464748824823,0.152483274684963,1.72613059618619));
#24559=CARTESIAN_POINT('Ctrl Pts',(1.55492717401663,0.429627033563921,1.88706341654737));
#24560=CARTESIAN_POINT('Ctrl Pts',(1.07691421721301,-0.0427958338931188,
1.28318517919043));
#24561=CARTESIAN_POINT('Ctrl Pts',(1.30240853234962,-0.00374333123643632,
1.53754499301448));
#24562=CARTESIAN_POINT('Ctrl Pts',(1.45458565734394,0.152519741700297,1.74612783237292));
#24563=CARTESIAN_POINT('Ctrl Pts',(1.53344559219597,0.425993384917079,1.90893369726574));
#24564=CARTESIAN_POINT('',(1.08053472770428,-0.042157609369957,1.28727233489076));
#24565=CARTESIAN_POINT('Ctrl Pts',(1.08053472770428,-0.042157609369957,
1.28727233489076));
#24566=CARTESIAN_POINT('Ctrl Pts',(1.18019989616608,-0.0242791587196548,
1.39987124007464));
#24567=CARTESIAN_POINT('Ctrl Pts',(1.26544208722232,0.0166569869072258,
1.50346488650363));
#24568=CARTESIAN_POINT('Ctrl Pts',(1.42418037408903,0.16009648734447,1.715480776583));
#24569=CARTESIAN_POINT('Ctrl Pts',(1.48987049850469,0.275079075974333,1.81902921434248));
#24570=CARTESIAN_POINT('Ctrl Pts',(1.53333167412,0.425598593400271,1.90869858745619));
#24571=CARTESIAN_POINT('',(1.26108935601086,0.0260686553993157,1.10727038327973));
#24572=CARTESIAN_POINT('Ctrl Pts',(1.26108935601086,0.0260686553993156,
1.10727038327973));
#24573=CARTESIAN_POINT('Ctrl Pts',(1.2406663502733,0.0102738810212643,1.12801545944048));
#24574=CARTESIAN_POINT('Ctrl Pts',(1.21735780368012,-0.00544822415320415,
1.15133239961429));
#24575=CARTESIAN_POINT('Ctrl Pts',(1.17324021107684,-0.0280274542414253,
1.19509600545496));
#24576=CARTESIAN_POINT('Ctrl Pts',(1.15484454191165,-0.0355561559109166,
1.21324740617461));
#24577=CARTESIAN_POINT('Ctrl Pts',(1.12241703607502,-0.0433677241466835,
1.24538218411131));
#24578=CARTESIAN_POINT('Ctrl Pts',(1.10404988380787,-0.0455044376575776,
1.26364457695046));
#24579=CARTESIAN_POINT('Ctrl Pts',(1.08053472770428,-0.0421576093699569,
1.28727233489076));
#24580=CARTESIAN_POINT('Ctrl Pts',(1.76386916735272,0.602229799711917,1.63615580822897));
#24581=CARTESIAN_POINT('Ctrl Pts',(1.74092498377317,0.497389884697104,1.58735805514604));
#24582=CARTESIAN_POINT('Ctrl Pts',(1.70624968855527,0.406388294299235,1.53858095020832));
#24583=CARTESIAN_POINT('Ctrl Pts',(1.61071325107043,0.240766166368977,1.42806953503213));
#24584=CARTESIAN_POINT('Ctrl Pts',(1.54601110868789,0.168977132257998,1.36461306044571));
#24585=CARTESIAN_POINT('Ctrl Pts',(1.40397010717826,0.0713877673286496,
1.23357020765531));
#24586=CARTESIAN_POINT('Ctrl Pts',(1.33378082531076,0.0423971966252646,
1.17136442658356));
#24587=CARTESIAN_POINT('Ctrl Pts',(1.26108935601086,0.0260686553993155,
1.10727038327973));
#24588=CARTESIAN_POINT('Ctrl Pts',(1.08053472770428,-0.042157609369957,
1.28727233489076));
#24589=CARTESIAN_POINT('Ctrl Pts',(1.30462473967982,-0.00195919018135088,
1.54044292999952));
#24590=CARTESIAN_POINT('Ctrl Pts',(1.45580038421926,0.154805815536382,1.74808806061869));
#24591=CARTESIAN_POINT('Ctrl Pts',(1.5340616613226,0.428137407783241,1.91020772674828));
#24592=CARTESIAN_POINT('Ctrl Pts',(1.07622999908393,-0.0853753293366666,
1.28727233489076));
#24593=CARTESIAN_POINT('Ctrl Pts',(1.30138937207125,-0.0542581740029552,
1.54044292999952));
#24594=CARTESIAN_POINT('Ctrl Pts',(1.45848408198029,0.0960667204863551,
1.74808806061869));
#24595=CARTESIAN_POINT('Ctrl Pts',(1.54751412881105,0.365599354131263,1.91020772674828));
#24596=CARTESIAN_POINT('Ctrl Pts',(1.07192527046357,-0.128593049303376,
1.28727233489076));
#24597=CARTESIAN_POINT('Ctrl Pts',(1.29815400446268,-0.106557157824559,
1.54044292999952));
#24598=CARTESIAN_POINT('Ctrl Pts',(1.46116777974132,0.0373276254363271,
1.74808806061869));
#24599=CARTESIAN_POINT('Ctrl Pts',(1.56096659629949,0.303061300479284,1.91020772674828));
#24600=CARTESIAN_POINT('Ctrl Pts',(1.06762054184321,-0.171810769270086,
1.28727233489076));
#24601=CARTESIAN_POINT('Ctrl Pts',(1.29491863685411,-0.158856141646164,
1.54044292999952));
#24602=CARTESIAN_POINT('Ctrl Pts',(1.46385147750235,-0.0214114696136997,
1.74808806061869));
#24603=CARTESIAN_POINT('Ctrl Pts',(1.57441906378793,0.240523246827306,1.91020772674828));
#24604=CARTESIAN_POINT('',(1.06762054184321,-0.171810769270086,1.28727233489076));
#24605=CARTESIAN_POINT('Ctrl Pts',(1.06762054184321,-0.171810769270086,
1.28727233489076));
#24606=CARTESIAN_POINT('Ctrl Pts',(1.16871252149279,-0.166049132983329,
1.39987124007464));
#24607=CARTESIAN_POINT('Ctrl Pts',(1.2582594411694,-0.135662485730195,1.50346488650363));
#24608=CARTESIAN_POINT('Ctrl Pts',(1.43309732687145,-0.0123561690781439,
1.715480776583));
#24609=CARTESIAN_POINT('Ctrl Pts',(1.51213990150266,0.0938909933754471,
1.81902921434248));
#24610=CARTESIAN_POINT('Ctrl Pts',(1.57338902476662,0.238090659850088,1.90869858745619));
#24611=CARTESIAN_POINT('Ctrl Pts',(1.08053472770428,-0.0421576093699569,
1.28727233489076));
#24612=CARTESIAN_POINT('Ctrl Pts',(1.07899219081063,-0.063749697386048,
1.28797191329047));
#24613=CARTESIAN_POINT('Ctrl Pts',(1.07715333835806,-0.085320709379581,
1.28831907556383));
#24614=CARTESIAN_POINT('Ctrl Pts',(1.07501072349525,-0.106872735707655,
1.288319084765));
#24615=CARTESIAN_POINT('Ctrl Pts',(1.07285470149866,-0.128559621036836,
1.28831909402374));
#24616=CARTESIAN_POINT('Ctrl Pts',(1.07039324377381,-0.150205375722348,
1.28796761487395));
#24617=CARTESIAN_POINT('Ctrl Pts',(1.06762054184321,-0.171810769270086,
1.28727233489076));
#24618=CARTESIAN_POINT('Ctrl Pts',(1.06394999323939,-0.172008888562255,
1.28318567027397));
#24619=CARTESIAN_POINT('Ctrl Pts',(1.29246819705105,-0.160362437711244,
1.53750524708654));
#24620=CARTESIAN_POINT('Ctrl Pts',(1.46231724071037,-0.0235777272478809,
1.74606230994598));
#24621=CARTESIAN_POINT('Ctrl Pts',(1.57349712421737,0.238345242827835,1.90885685885231));
#24622=CARTESIAN_POINT('Ctrl Pts',(1.07868660104758,-0.172859184352678,
1.26847655615066));
#24623=CARTESIAN_POINT('Ctrl Pts',(1.3103222134962,-0.160753680728286,1.51986758573726));
#24624=CARTESIAN_POINT('Ctrl Pts',(1.48218330046157,-0.021871343434585,
1.72610301145358));
#24625=CARTESIAN_POINT('Ctrl Pts',(1.59454602809666,0.243802951242388,1.88702818957259));
#24626=CARTESIAN_POINT('Ctrl Pts',(1.10570674896705,-0.177804653077212,
1.24116990569733));
#24627=CARTESIAN_POINT('Ctrl Pts',(1.34316333686973,-0.165504346014847,
1.48715046268483));
#24628=CARTESIAN_POINT('Ctrl Pts',(1.51954463753721,-0.0232151943402924,
1.68886632718445));
#24629=CARTESIAN_POINT('Ctrl Pts',(1.6348527774955,0.24905417978714,1.84632060216323));
#24630=CARTESIAN_POINT('Ctrl Pts',(1.16355922492391,-0.208466679481999,
1.18070487506193));
#24631=CARTESIAN_POINT('Ctrl Pts',(1.41450672434568,-0.200040692821152,
1.41458132511535));
#24632=CARTESIAN_POINT('Ctrl Pts',(1.60338306284494,-0.0532381927575528,
1.60640786607656));
#24633=CARTESIAN_POINT('Ctrl Pts',(1.73033000148215,0.231963750155414,1.75609772232067));
#24634=CARTESIAN_POINT('Ctrl Pts',(1.20636704429046,-0.248125323472877,
1.13427377111504));
#24635=CARTESIAN_POINT('Ctrl Pts',(1.46792997975155,-0.246071577739378,
1.35898374075971));
#24636=CARTESIAN_POINT('Ctrl Pts',(1.66851401508092,-0.0981643196522479,
1.54328012485139));
#24637=CARTESIAN_POINT('Ctrl Pts',(1.80834740097598,0.195461560119271,1.68710766933124));
#24638=CARTESIAN_POINT('Ctrl Pts',(1.23564132105363,-0.2815945488883,1.10188997515679));
#24639=CARTESIAN_POINT('Ctrl Pts',(1.50471693589153,-0.285103641318398,
1.32023346555538));
#24640=CARTESIAN_POINT('Ctrl Pts',(1.71433203676124,-0.137346033394656,
1.49928432698175));
#24641=CARTESIAN_POINT('Ctrl Pts',(1.86448662366276,0.161678274882928,1.63904255943589));
#24642=CARTESIAN_POINT('Ctrl Pts',(1.06762054184321,-0.171810769270086,
1.28727233489076));
#24643=CARTESIAN_POINT('Ctrl Pts',(1.10022966448202,-0.173665579012752,
1.2547827394351));
#24644=CARTESIAN_POINT('Ctrl Pts',(1.12545255134417,-0.184128327165875,
1.22829923781307));
#24645=CARTESIAN_POINT('Ctrl Pts',(1.17633816045211,-0.219433599811049,
1.17205963503587));
#24646=CARTESIAN_POINT('Ctrl Pts',(1.20325508885486,-0.243258020496387,
1.14130666672786));
#24647=CARTESIAN_POINT('Ctrl Pts',(1.23077165948193,-0.27609248605186,1.10727038327973));
#24648=CARTESIAN_POINT('Origin',(0.,0.,1.38794976669063));
#24649=CARTESIAN_POINT('',(-0.7,-8.57252759403147E-17,1.66862915010152));
#24650=CARTESIAN_POINT('Origin',(0.,0.,1.66862915010152));
#24651=CARTESIAN_POINT('',(-0.980679383410898,-1.20098586788396E-16,1.38794976669063));
#24652=CARTESIAN_POINT('Origin',(0.,0.,1.10727038327973));
#24653=CARTESIAN_POINT('Origin',(0.,0.,1.37171309575435));
#24654=CARTESIAN_POINT('Origin',(1.,0.,2.1));
#24655=CARTESIAN_POINT('Origin',(0.541,0.,2.6));
#24656=CARTESIAN_POINT('',(-0.541,-6.62533918338718E-17,2.6));
#24657=CARTESIAN_POINT('Origin',(0.,0.,2.6));
#24658=CARTESIAN_POINT('Origin',(0.,0.,2.58));
#24659=CARTESIAN_POINT('',(-0.501,-6.13548046372824E-17,2.56));
#24660=CARTESIAN_POINT('',(-0.521,-6.38040982355771E-17,2.58));
#24661=CARTESIAN_POINT('Origin',(0.,0.,2.56));
#24662=CARTESIAN_POINT('Origin',(0.,0.,2.13431457505076));
#24663=CARTESIAN_POINT('',(-0.501,-6.13548046372824E-17,1.70862915010152));
#24664=CARTESIAN_POINT('',(-0.501,-6.13548046372824E-17,2.13431457505076));
#24665=CARTESIAN_POINT('Origin',(0.,0.,1.70862915010152));
#24666=CARTESIAN_POINT('Origin',(0.,0.,1.68862915010152));
#24667=CARTESIAN_POINT('',(-0.541,-6.62533918338718E-17,1.66862915010152));
#24668=CARTESIAN_POINT('',(-0.521,-6.38040982355771E-17,1.68862915010152));
#24669=CARTESIAN_POINT('Origin',(0.,0.,1.66862915010152));
#24670=CARTESIAN_POINT('Origin',(0.7,0.,1.66862915010152));
#31617=UNCERTAINTY_MEASURE_WITH_UNIT(LENGTH_MEASURE(0.001),#31639,
'DISTANCE_ACCURACY_VALUE',
'Maximum model space distance between geometric entities at asserted c
onnectivities');
#31625=UNCERTAINTY_MEASURE_WITH_UNIT(LENGTH_MEASURE(0.001),#31639,
'DISTANCE_ACCURACY_VALUE',
'Maximum model space distance between geometric entities at asserted c
onnectivities');
#31630=(
GEOMETRIC_REPRESENTATION_CONTEXT(3)
GLOBAL_UNCERTAINTY_ASSIGNED_CONTEXT((#31617))
GLOBAL_UNIT_ASSIGNED_CONTEXT((#31639,#31641,#31642))
REPRESENTATION_CONTEXT('','3D')
);
#31638=(
GEOMETRIC_REPRESENTATION_CONTEXT(3)
GLOBAL_UNCERTAINTY_ASSIGNED_CONTEXT((#31625))
GLOBAL_UNIT_ASSIGNED_CONTEXT((#31639,#31641,#31642))
REPRESENTATION_CONTEXT('','3D')
);
#31639=(
LENGTH_UNIT()
NAMED_UNIT(*)
SI_UNIT(.CENTI.,.METRE.)
);
#31641=(
NAMED_UNIT(*)
PLANE_ANGLE_UNIT()
SI_UNIT($,.RADIAN.)
);
#31642=(
NAMED_UNIT(*)
SI_UNIT($,.STERADIAN.)
SOLID_ANGLE_UNIT()
);
#31647=SHAPE_DEFINITION_REPRESENTATION(#31659,#31708);
#31659=PRODUCT_DEFINITION_SHAPE('',$,#31721);
#31708=SHAPE_REPRESENTATION('',(#12900),#31630);
#31716=PRODUCT_DEFINITION_CONTEXT('part definition',#31754,'design');
#31721=PRODUCT_DEFINITION('2026-10-22-02-42-16-551',
'04_Spiral_Bevel_Side_Gear_m1.75_z20_RH_Output',#31733,#31716);
#31733=PRODUCT_DEFINITION_FORMATION('',$,#31760);
#31754=APPLICATION_CONTEXT(
'Core Data for Automotive Mechanical Design Process');
#31755=PRODUCT_CONTEXT('part definition',#31754,'mechanical');
#31760=PRODUCT('2026-10-22-02-42-16-551',
'04_Spiral_Bevel_Side_Gear_m1.75_z20_RH_Output',$,(#31755));
#31817=COLOUR_RGB('Sky Blue',0.24,0.69,0.87);
#31818=FILL_AREA_STYLE_COLOUR('',#31817);
#31819=FILL_AREA_STYLE('',(#31818));
#31820=SURFACE_STYLE_FILL_AREA(#31819);
#31821=SURFACE_SIDE_STYLE('',(#31820));
#31822=SURFACE_STYLE_USAGE(.BOTH.,#31821);
#31823=PRESENTATION_STYLE_ASSIGNMENT((#31822));
ENDSEC;
END-ISO-10303-21;
